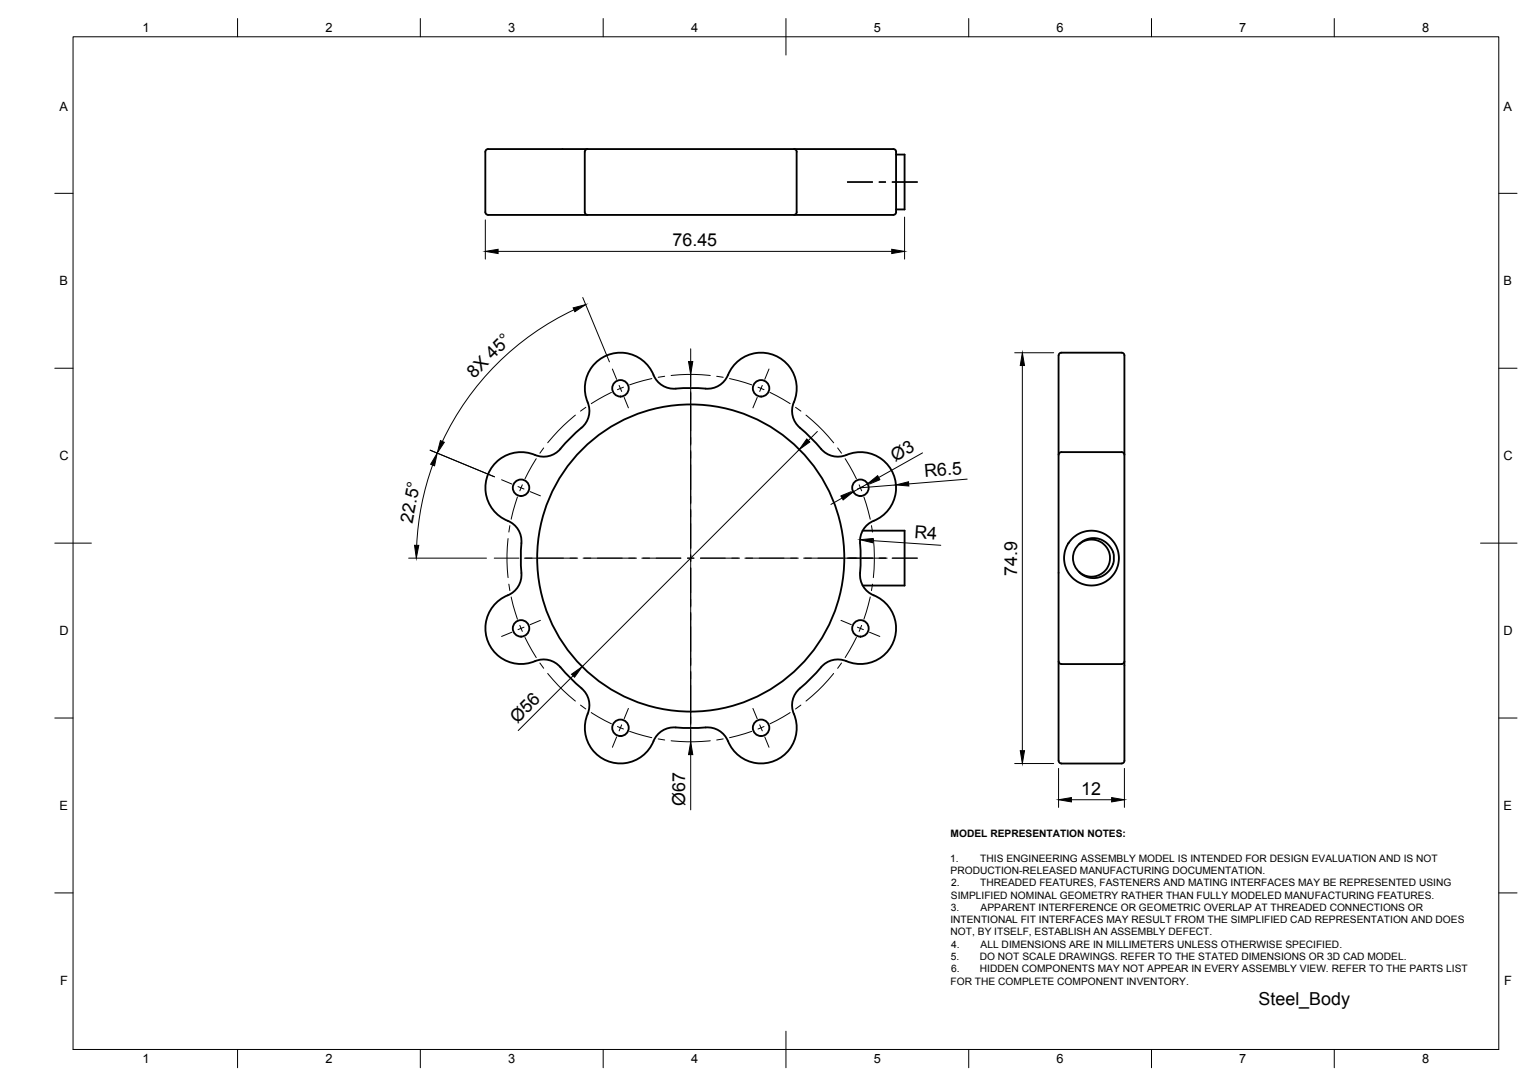
ISO-10303-21;
HEADER;
/* Generated by software containing ST-Developer
 * from STEP Tools, Inc. (www.steptools.com) 
 */

FILE_DESCRIPTION(
/* description */ (''),
/* implementation_level */ '2;1');

FILE_NAME(
/* name */ 'Steel_Body.step',
/* time_stamp */ '2026-10-06T12:52:28-07:00',
/* author */ (''),
/* organization */ (''),
/* preprocessor_version */ 'ST-DEVELOPER v20.2',
/* originating_system */ 'Autodesk Translation Framework v15.15.0.0',
/* authorisation */ '');

FILE_SCHEMA (('AUTOMOTIVE_DESIGN { 1 0 10303 214 3 1 1 }'));
ENDSEC;

DATA;
#10=MECHANICAL_DESIGN_GEOMETRIC_PRESENTATION_REPRESENTATION('',(#79),#34403);
#55=B_SPLINE_SURFACE_WITH_KNOTS('',3,3,((#32660,#32661,#32662,#32663,#32664,
#32665,#32666,#32667,#32668,#32669,#32670,#32671,#32672,#32673,#32674,#32675,
#32676,#32677,#32678,#32679,#32680,#32681,#32682,#32683,#32684,#32685,#32686,
#32687,#32688,#32689,#32690,#32691,#32692,#32693,#32694,#32695,#32696,#32697,
#32698,#32699,#32700,#32701,#32702,#32703,#32704,#32705,#32706,#32707,#32708,
#32709,#32710,#32711,#32712,#32713,#32714,#32715,#32716,#32717,#32718,#32719,
#32720),(#32721,#32722,#32723,#32724,#32725,#32726,#32727,#32728,#32729,
#32730,#32731,#32732,#32733,#32734,#32735,#32736,#32737,#32738,#32739,#32740,
#32741,#32742,#32743,#32744,#32745,#32746,#32747,#32748,#32749,#32750,#32751,
#32752,#32753,#32754,#32755,#32756,#32757,#32758,#32759,#32760,#32761,#32762,
#32763,#32764,#32765,#32766,#32767,#32768,#32769,#32770,#32771,#32772,#32773,
#32774,#32775,#32776,#32777,#32778,#32779,#32780,#32781),(#32782,#32783,
#32784,#32785,#32786,#32787,#32788,#32789,#32790,#32791,#32792,#32793,#32794,
#32795,#32796,#32797,#32798,#32799,#32800,#32801,#32802,#32803,#32804,#32805,
#32806,#32807,#32808,#32809,#32810,#32811,#32812,#32813,#32814,#32815,#32816,
#32817,#32818,#32819,#32820,#32821,#32822,#32823,#32824,#32825,#32826,#32827,
#32828,#32829,#32830,#32831,#32832,#32833,#32834,#32835,#32836,#32837,#32838,
#32839,#32840,#32841,#32842),(#32843,#32844,#32845,#32846,#32847,#32848,
#32849,#32850,#32851,#32852,#32853,#32854,#32855,#32856,#32857,#32858,#32859,
#32860,#32861,#32862,#32863,#32864,#32865,#32866,#32867,#32868,#32869,#32870,
#32871,#32872,#32873,#32874,#32875,#32876,#32877,#32878,#32879,#32880,#32881,
#32882,#32883,#32884,#32885,#32886,#32887,#32888,#32889,#32890,#32891,#32892,
#32893,#32894,#32895,#32896,#32897,#32898,#32899,#32900,#32901,#32902,#32903)),
 .UNSPECIFIED.,.F.,.F.,.F.,(4,4),(4,1,1,1,1,1,1,1,1,1,1,1,1,1,1,1,1,1,1,
1,1,1,1,1,1,1,1,1,1,1,1,1,1,1,1,1,1,1,1,1,1,1,1,1,1,1,1,1,1,1,1,1,1,1,1,
1,1,1,4),(-0.000677904662105755,0.0806892635940671),(11.8568599181543,12.8456361179191,
13.8337344130217,14.8218327081244,15.8099310032271,16.7980292983297,17.7861275934324,
18.774225888535,19.7623241836377,20.7504224787404,21.738520773843,22.7266190689457,
23.7147173640484,24.702815659151,25.6909139542537,26.6790122493564,27.667110544459,
28.6552088395617,29.6433071346644,30.631405429767,31.6195037248697,32.6076020199723,
33.595700315075,34.5837986101777,35.5718969052803,36.559995200383,37.5480934954857,
38.5361917905883,39.524290085691,40.5123883807937,41.5004866758963,42.488584970999,
43.4766832661016,44.4647815612043,45.452879856307,46.4409781514096,47.4290764465123,
48.417174741615,49.4052730367176,50.3933713318203,51.381469626923,52.3695679220256,
53.3576662171283,54.345764512231,55.3338628073336,56.3219611024363,57.3100593975389,
58.2981576926416,59.2862559877443,60.2743542828469,61.2624525779496,62.2505508730523,
63.2386491681549,64.2267474632576,65.2148457583603,66.2029440534629,67.1910423485656,
68.1791406436682,69.1672389387709),.UNSPECIFIED.);
#56=B_SPLINE_SURFACE_WITH_KNOTS('',3,3,((#33092,#33093,#33094,#33095,#33096,
#33097,#33098,#33099,#33100,#33101,#33102,#33103,#33104,#33105,#33106,#33107,
#33108,#33109,#33110,#33111,#33112,#33113,#33114,#33115,#33116,#33117,#33118,
#33119,#33120,#33121,#33122,#33123,#33124,#33125,#33126,#33127,#33128,#33129,
#33130,#33131,#33132,#33133,#33134,#33135,#33136,#33137,#33138,#33139,#33140,
#33141,#33142,#33143,#33144,#33145,#33146,#33147,#33148,#33149,#33150,#33151,
#33152),(#33153,#33154,#33155,#33156,#33157,#33158,#33159,#33160,#33161,
#33162,#33163,#33164,#33165,#33166,#33167,#33168,#33169,#33170,#33171,#33172,
#33173,#33174,#33175,#33176,#33177,#33178,#33179,#33180,#33181,#33182,#33183,
#33184,#33185,#33186,#33187,#33188,#33189,#33190,#33191,#33192,#33193,#33194,
#33195,#33196,#33197,#33198,#33199,#33200,#33201,#33202,#33203,#33204,#33205,
#33206,#33207,#33208,#33209,#33210,#33211,#33212,#33213),(#33214,#33215,
#33216,#33217,#33218,#33219,#33220,#33221,#33222,#33223,#33224,#33225,#33226,
#33227,#33228,#33229,#33230,#33231,#33232,#33233,#33234,#33235,#33236,#33237,
#33238,#33239,#33240,#33241,#33242,#33243,#33244,#33245,#33246,#33247,#33248,
#33249,#33250,#33251,#33252,#33253,#33254,#33255,#33256,#33257,#33258,#33259,
#33260,#33261,#33262,#33263,#33264,#33265,#33266,#33267,#33268,#33269,#33270,
#33271,#33272,#33273,#33274),(#33275,#33276,#33277,#33278,#33279,#33280,
#33281,#33282,#33283,#33284,#33285,#33286,#33287,#33288,#33289,#33290,#33291,
#33292,#33293,#33294,#33295,#33296,#33297,#33298,#33299,#33300,#33301,#33302,
#33303,#33304,#33305,#33306,#33307,#33308,#33309,#33310,#33311,#33312,#33313,
#33314,#33315,#33316,#33317,#33318,#33319,#33320,#33321,#33322,#33323,#33324,
#33325,#33326,#33327,#33328,#33329,#33330,#33331,#33332,#33333,#33334,#33335)),
 .UNSPECIFIED.,.F.,.F.,.F.,(4,4),(4,1,1,1,1,1,1,1,1,1,1,1,1,1,1,1,1,1,1,
1,1,1,1,1,1,1,1,1,1,1,1,1,1,1,1,1,1,1,1,1,1,1,1,1,1,1,1,1,1,1,1,1,1,1,1,
1,1,1,4),(-0.000408738892527466,0.0809585600709479),(14.3991256467175,15.3872239418202,
16.3753222369229,17.3634205320255,18.3515188271282,19.3396171222308,20.3277154173335,
21.3158137124362,22.3039120075388,23.2920103026415,24.2801085977442,25.2682068928468,
26.2563051879495,27.2444034830521,28.2325017781548,29.2206000732575,30.2086983683601,
31.1967966634628,32.1848949585655,33.1729932536681,34.1610915487708,35.1491898438735,
36.1372881389761,37.1253864340788,38.1134847291814,39.1015830242841,40.0896813193868,
41.0777796144894,42.0658779095921,43.0539762046948,44.0420744997974,45.0301727949001,
46.0182710900028,47.0063693851054,47.9944676802081,48.9825659753107,49.9706642704134,
50.9587625655161,51.9468608606187,52.9349591557214,53.9230574508241,54.9111557459267,
55.8992540410294,56.8873523361321,57.8754506312347,58.8635489263374,59.85164722144,
60.8397455165427,61.8278438116454,62.815942106748,63.8040404018507,64.7921386969534,
65.780236992056,66.7683352871587,67.7564335822614,68.744531877364,69.7326301724667,
70.7207284675693,71.7095047678121),.UNSPECIFIED.);
#63=SHAPE_REPRESENTATION_RELATIONSHIP('SRR','None',#34441,#71);
#71=ADVANCED_BREP_SHAPE_REPRESENTATION('',(#87),#34401);
#79=STYLED_ITEM('',(#34484),#87);
#87=MANIFOLD_SOLID_BREP('Body1',#4388);
#102=FACE_BOUND('',#855,.T.);
#103=FACE_BOUND('',#858,.T.);
#104=FACE_BOUND('',#914,.T.);
#105=FACE_BOUND('',#915,.T.);
#106=FACE_BOUND('',#916,.T.);
#107=FACE_BOUND('',#917,.T.);
#108=FACE_BOUND('',#918,.T.);
#109=FACE_BOUND('',#919,.T.);
#110=FACE_BOUND('',#920,.T.);
#111=FACE_BOUND('',#921,.T.);
#112=FACE_BOUND('',#922,.T.);
#113=FACE_BOUND('',#970,.T.);
#114=FACE_BOUND('',#971,.T.);
#115=FACE_BOUND('',#972,.T.);
#116=FACE_BOUND('',#973,.T.);
#117=FACE_BOUND('',#974,.T.);
#118=FACE_BOUND('',#975,.T.);
#119=FACE_BOUND('',#976,.T.);
#120=FACE_BOUND('',#977,.T.);
#121=FACE_BOUND('',#978,.T.);
#122=FACE_BOUND('',#981,.T.);
#123=FACE_BOUND('',#982,.T.);
#143=PLANE('',#4620);
#144=PLANE('',#4625);
#145=PLANE('',#4794);
#146=PLANE('',#4928);
#207=CIRCLE('',#4606,4.085);
#208=CIRCLE('',#4615,4.085);
#209=CIRCLE('',#4617,3.38975);
#210=CIRCLE('',#4618,3.38975);
#211=CIRCLE('',#4621,5.);
#212=CIRCLE('',#4622,5.);
#213=CIRCLE('',#4624,5.);
#214=CIRCLE('',#4630,4.);
#215=CIRCLE('',#4631,4.);
#216=CIRCLE('',#4633,31.);
#217=CIRCLE('',#4635,4.);
#218=CIRCLE('',#4636,4.);
#219=CIRCLE('',#4638,31.);
#220=CIRCLE('',#4640,0.499999999999994);
#221=CIRCLE('',#4641,4.5);
#222=CIRCLE('',#4642,0.5);
#223=CIRCLE('',#4644,0.5);
#224=CIRCLE('',#4645,6.5);
#225=CIRCLE('',#4646,6.);
#226=CIRCLE('',#4648,0.5);
#227=CIRCLE('',#4649,4.);
#228=CIRCLE('',#4650,4.5);
#229=CIRCLE('',#4652,0.5);
#230=CIRCLE('',#4653,31.);
#231=CIRCLE('',#4654,30.5);
#232=CIRCLE('',#4656,0.5);
#233=CIRCLE('',#4657,4.);
#234=CIRCLE('',#4658,4.5);
#235=CIRCLE('',#4660,0.5);
#236=CIRCLE('',#4661,6.5);
#237=CIRCLE('',#4662,6.);
#238=CIRCLE('',#4664,0.5);
#239=CIRCLE('',#4665,4.);
#240=CIRCLE('',#4666,4.5);
#241=CIRCLE('',#4668,0.5);
#242=CIRCLE('',#4669,31.);
#243=CIRCLE('',#4670,30.5);
#244=CIRCLE('',#4672,0.5);
#245=CIRCLE('',#4673,4.);
#246=CIRCLE('',#4674,4.5);
#247=CIRCLE('',#4676,0.5);
#248=CIRCLE('',#4677,6.5);
#249=CIRCLE('',#4678,6.);
#250=CIRCLE('',#4680,0.5);
#251=CIRCLE('',#4681,4.);
#252=CIRCLE('',#4682,4.5);
#253=CIRCLE('',#4684,0.5);
#254=CIRCLE('',#4685,31.);
#255=CIRCLE('',#4686,30.5);
#256=CIRCLE('',#4688,0.5);
#257=CIRCLE('',#4689,4.);
#258=CIRCLE('',#4690,4.5);
#259=CIRCLE('',#4692,0.5);
#260=CIRCLE('',#4693,6.5);
#261=CIRCLE('',#4694,6.);
#262=CIRCLE('',#4696,0.5);
#263=CIRCLE('',#4697,4.5);
#264=CIRCLE('',#4699,0.5);
#265=CIRCLE('',#4700,31.);
#266=CIRCLE('',#4701,30.5);
#267=CIRCLE('',#4703,0.5);
#268=CIRCLE('',#4704,4.);
#269=CIRCLE('',#4705,4.5);
#270=CIRCLE('',#4707,0.5);
#271=CIRCLE('',#4708,6.5);
#272=CIRCLE('',#4709,6.);
#273=CIRCLE('',#4711,0.5);
#274=CIRCLE('',#4712,4.);
#275=CIRCLE('',#4713,4.5);
#276=CIRCLE('',#4715,0.5);
#277=CIRCLE('',#4716,31.);
#278=CIRCLE('',#4717,30.5);
#279=CIRCLE('',#4719,0.5);
#280=CIRCLE('',#4720,4.);
#281=CIRCLE('',#4721,4.5);
#282=CIRCLE('',#4723,0.5);
#283=CIRCLE('',#4724,6.5);
#284=CIRCLE('',#4725,6.);
#285=CIRCLE('',#4727,0.5);
#286=CIRCLE('',#4728,4.);
#287=CIRCLE('',#4729,4.5);
#288=CIRCLE('',#4731,0.5);
#289=CIRCLE('',#4732,31.);
#290=CIRCLE('',#4733,30.5);
#291=CIRCLE('',#4735,0.5);
#292=CIRCLE('',#4736,4.);
#293=CIRCLE('',#4737,4.5);
#294=CIRCLE('',#4739,0.5);
#295=CIRCLE('',#4740,6.5);
#296=CIRCLE('',#4741,6.);
#297=CIRCLE('',#4743,0.5);
#298=CIRCLE('',#4744,4.);
#299=CIRCLE('',#4745,4.5);
#300=CIRCLE('',#4747,0.5);
#301=CIRCLE('',#4748,31.);
#302=CIRCLE('',#4749,30.5);
#303=CIRCLE('',#4751,0.5);
#304=CIRCLE('',#4752,4.);
#305=CIRCLE('',#4753,4.5);
#306=CIRCLE('',#4755,0.5);
#307=CIRCLE('',#4756,6.5);
#308=CIRCLE('',#4757,6.);
#309=CIRCLE('',#4759,0.5);
#310=CIRCLE('',#4760,4.);
#311=CIRCLE('',#4761,4.5);
#312=CIRCLE('',#4763,30.5);
#313=CIRCLE('',#4765,6.5);
#314=CIRCLE('',#4767,4.);
#315=CIRCLE('',#4769,31.);
#316=CIRCLE('',#4771,4.);
#317=CIRCLE('',#4773,6.5);
#318=CIRCLE('',#4775,4.);
#319=CIRCLE('',#4777,31.);
#320=CIRCLE('',#4779,4.);
#321=CIRCLE('',#4781,6.5);
#322=CIRCLE('',#4783,4.);
#323=CIRCLE('',#4785,31.);
#324=CIRCLE('',#4787,4.);
#325=CIRCLE('',#4789,6.5);
#326=CIRCLE('',#4791,4.);
#327=CIRCLE('',#4793,31.);
#328=CIRCLE('',#4795,28.5);
#329=CIRCLE('',#4796,1.5);
#330=CIRCLE('',#4797,1.5);
#331=CIRCLE('',#4798,1.5);
#332=CIRCLE('',#4799,1.5);
#333=CIRCLE('',#4800,1.5);
#334=CIRCLE('',#4801,1.5);
#335=CIRCLE('',#4802,1.5);
#336=CIRCLE('',#4803,1.5);
#337=CIRCLE('',#4805,0.500000000000001);
#338=CIRCLE('',#4806,4.5);
#339=CIRCLE('',#4807,0.5);
#340=CIRCLE('',#4808,4.);
#341=CIRCLE('',#4810,0.5);
#342=CIRCLE('',#4811,6.5);
#343=CIRCLE('',#4812,6.);
#344=CIRCLE('',#4814,0.5);
#345=CIRCLE('',#4815,4.5);
#346=CIRCLE('',#4817,0.5);
#347=CIRCLE('',#4818,30.5);
#348=CIRCLE('',#4820,0.5);
#349=CIRCLE('',#4821,4.5);
#350=CIRCLE('',#4823,0.5);
#351=CIRCLE('',#4824,6.);
#352=CIRCLE('',#4826,0.5);
#353=CIRCLE('',#4827,4.5);
#354=CIRCLE('',#4829,0.5);
#355=CIRCLE('',#4830,30.5);
#356=CIRCLE('',#4832,0.5);
#357=CIRCLE('',#4833,4.5);
#358=CIRCLE('',#4835,0.5);
#359=CIRCLE('',#4836,6.);
#360=CIRCLE('',#4838,0.5);
#361=CIRCLE('',#4839,4.5);
#362=CIRCLE('',#4841,0.5);
#363=CIRCLE('',#4842,30.5);
#364=CIRCLE('',#4844,0.5);
#365=CIRCLE('',#4845,4.5);
#366=CIRCLE('',#4847,0.5);
#367=CIRCLE('',#4848,6.);
#368=CIRCLE('',#4850,0.5);
#369=CIRCLE('',#4851,4.5);
#370=CIRCLE('',#4853,0.5);
#371=CIRCLE('',#4854,30.5);
#372=CIRCLE('',#4856,0.5);
#373=CIRCLE('',#4857,4.5);
#374=CIRCLE('',#4859,0.5);
#375=CIRCLE('',#4860,6.);
#376=CIRCLE('',#4862,0.5);
#377=CIRCLE('',#4863,4.);
#378=CIRCLE('',#4864,4.5);
#379=CIRCLE('',#4866,0.5);
#380=CIRCLE('',#4867,30.5);
#381=CIRCLE('',#4869,0.5);
#382=CIRCLE('',#4870,4.5);
#383=CIRCLE('',#4872,0.5);
#384=CIRCLE('',#4873,6.5);
#385=CIRCLE('',#4874,6.);
#386=CIRCLE('',#4876,0.5);
#387=CIRCLE('',#4877,4.);
#388=CIRCLE('',#4878,4.5);
#389=CIRCLE('',#4880,0.5);
#390=CIRCLE('',#4881,31.);
#391=CIRCLE('',#4882,30.5);
#392=CIRCLE('',#4884,0.5);
#393=CIRCLE('',#4885,4.);
#394=CIRCLE('',#4886,4.5);
#395=CIRCLE('',#4888,0.5);
#396=CIRCLE('',#4889,6.5);
#397=CIRCLE('',#4890,6.);
#398=CIRCLE('',#4892,0.5);
#399=CIRCLE('',#4893,4.);
#400=CIRCLE('',#4894,4.5);
#401=CIRCLE('',#4896,0.5);
#402=CIRCLE('',#4897,31.);
#403=CIRCLE('',#4898,30.5);
#404=CIRCLE('',#4900,0.5);
#405=CIRCLE('',#4901,4.);
#406=CIRCLE('',#4902,4.5);
#407=CIRCLE('',#4904,0.5);
#408=CIRCLE('',#4905,6.5);
#409=CIRCLE('',#4906,6.);
#410=CIRCLE('',#4908,0.5);
#411=CIRCLE('',#4909,4.);
#412=CIRCLE('',#4910,4.5);
#413=CIRCLE('',#4912,30.5);
#414=CIRCLE('',#4913,31.);
#415=CIRCLE('',#4929,28.5);
#416=CIRCLE('',#4930,1.5);
#417=CIRCLE('',#4931,1.5);
#418=CIRCLE('',#4932,1.5);
#419=CIRCLE('',#4933,1.5);
#420=CIRCLE('',#4934,1.5);
#421=CIRCLE('',#4935,1.5);
#422=CIRCLE('',#4936,1.5);
#423=CIRCLE('',#4937,1.5);
#424=CIRCLE('',#4939,0.5);
#425=CIRCLE('',#4940,28.);
#426=CIRCLE('',#4941,28.);
#427=CIRCLE('',#4943,28.);
#428=CIRCLE('',#4944,28.);
#429=CIRCLE('',#4946,0.5);
#450=TOROIDAL_SURFACE('',#4639,4.5,0.5);
#451=TOROIDAL_SURFACE('',#4643,6.,0.5);
#452=TOROIDAL_SURFACE('',#4647,4.5,0.5);
#453=TOROIDAL_SURFACE('',#4651,30.5,0.5);
#454=TOROIDAL_SURFACE('',#4655,4.5,0.5);
#455=TOROIDAL_SURFACE('',#4659,6.,0.5);
#456=TOROIDAL_SURFACE('',#4663,4.5,0.5);
#457=TOROIDAL_SURFACE('',#4667,30.5,0.5);
#458=TOROIDAL_SURFACE('',#4671,4.5,0.5);
#459=TOROIDAL_SURFACE('',#4675,6.,0.5);
#460=TOROIDAL_SURFACE('',#4679,4.5,0.5);
#461=TOROIDAL_SURFACE('',#4683,30.5,0.5);
#462=TOROIDAL_SURFACE('',#4687,4.5,0.5);
#463=TOROIDAL_SURFACE('',#4691,6.,0.5);
#464=TOROIDAL_SURFACE('',#4695,4.5,0.5);
#465=TOROIDAL_SURFACE('',#4698,30.5,0.5);
#466=TOROIDAL_SURFACE('',#4702,4.5,0.5);
#467=TOROIDAL_SURFACE('',#4706,6.,0.5);
#468=TOROIDAL_SURFACE('',#4710,4.5,0.5);
#469=TOROIDAL_SURFACE('',#4714,30.5,0.5);
#470=TOROIDAL_SURFACE('',#4718,4.5,0.5);
#471=TOROIDAL_SURFACE('',#4722,6.,0.5);
#472=TOROIDAL_SURFACE('',#4726,4.5,0.5);
#473=TOROIDAL_SURFACE('',#4730,30.5,0.5);
#474=TOROIDAL_SURFACE('',#4734,4.5,0.5);
#475=TOROIDAL_SURFACE('',#4738,6.,0.5);
#476=TOROIDAL_SURFACE('',#4742,4.5,0.5);
#477=TOROIDAL_SURFACE('',#4746,30.5,0.5);
#478=TOROIDAL_SURFACE('',#4750,4.5,0.5);
#479=TOROIDAL_SURFACE('',#4754,6.,0.5);
#480=TOROIDAL_SURFACE('',#4758,4.5,0.5);
#481=TOROIDAL_SURFACE('',#4762,30.5,0.5);
#482=TOROIDAL_SURFACE('',#4804,4.5,0.5);
#483=TOROIDAL_SURFACE('',#4809,6.,0.5);
#484=TOROIDAL_SURFACE('',#4813,4.5,0.5);
#485=TOROIDAL_SURFACE('',#4816,30.5,0.5);
#486=TOROIDAL_SURFACE('',#4819,4.5,0.5);
#487=TOROIDAL_SURFACE('',#4822,6.,0.5);
#488=TOROIDAL_SURFACE('',#4825,4.5,0.5);
#489=TOROIDAL_SURFACE('',#4828,30.5,0.5);
#490=TOROIDAL_SURFACE('',#4831,4.5,0.5);
#491=TOROIDAL_SURFACE('',#4834,6.,0.5);
#492=TOROIDAL_SURFACE('',#4837,4.5,0.5);
#493=TOROIDAL_SURFACE('',#4840,30.5,0.5);
#494=TOROIDAL_SURFACE('',#4843,4.5,0.5);
#495=TOROIDAL_SURFACE('',#4846,6.,0.5);
#496=TOROIDAL_SURFACE('',#4849,4.5,0.5);
#497=TOROIDAL_SURFACE('',#4852,30.5,0.5);
#498=TOROIDAL_SURFACE('',#4855,4.5,0.5);
#499=TOROIDAL_SURFACE('',#4858,6.,0.5);
#500=TOROIDAL_SURFACE('',#4861,4.5,0.5);
#501=TOROIDAL_SURFACE('',#4865,30.5,0.5);
#502=TOROIDAL_SURFACE('',#4868,4.5,0.5);
#503=TOROIDAL_SURFACE('',#4871,6.,0.5);
#504=TOROIDAL_SURFACE('',#4875,4.5,0.5);
#505=TOROIDAL_SURFACE('',#4879,30.5,0.5);
#506=TOROIDAL_SURFACE('',#4883,4.5,0.5);
#507=TOROIDAL_SURFACE('',#4887,6.,0.5);
#508=TOROIDAL_SURFACE('',#4891,4.5,0.5);
#509=TOROIDAL_SURFACE('',#4895,30.5,0.5);
#510=TOROIDAL_SURFACE('',#4899,4.5,0.5);
#511=TOROIDAL_SURFACE('',#4903,6.,0.5);
#512=TOROIDAL_SURFACE('',#4907,4.5,0.5);
#513=TOROIDAL_SURFACE('',#4911,30.5,0.5);
#514=TOROIDAL_SURFACE('',#4938,28.5,0.5);
#515=TOROIDAL_SURFACE('',#4945,28.5,0.5);
#597=FACE_OUTER_BOUND('',#841,.T.);
#598=FACE_OUTER_BOUND('',#842,.T.);
#599=FACE_OUTER_BOUND('',#843,.T.);
#600=FACE_OUTER_BOUND('',#844,.T.);
#601=FACE_OUTER_BOUND('',#845,.T.);
#602=FACE_OUTER_BOUND('',#846,.T.);
#603=FACE_OUTER_BOUND('',#847,.T.);
#604=FACE_OUTER_BOUND('',#848,.T.);
#605=FACE_OUTER_BOUND('',#849,.T.);
#606=FACE_OUTER_BOUND('',#850,.T.);
#607=FACE_OUTER_BOUND('',#851,.T.);
#608=FACE_OUTER_BOUND('',#852,.T.);
#609=FACE_OUTER_BOUND('',#853,.T.);
#610=FACE_OUTER_BOUND('',#854,.T.);
#611=FACE_OUTER_BOUND('',#856,.T.);
#612=FACE_OUTER_BOUND('',#857,.T.);
#613=FACE_OUTER_BOUND('',#859,.T.);
#614=FACE_OUTER_BOUND('',#860,.T.);
#615=FACE_OUTER_BOUND('',#861,.T.);
#616=FACE_OUTER_BOUND('',#862,.T.);
#617=FACE_OUTER_BOUND('',#863,.T.);
#618=FACE_OUTER_BOUND('',#864,.T.);
#619=FACE_OUTER_BOUND('',#865,.T.);
#620=FACE_OUTER_BOUND('',#866,.T.);
#621=FACE_OUTER_BOUND('',#867,.T.);
#622=FACE_OUTER_BOUND('',#868,.T.);
#623=FACE_OUTER_BOUND('',#869,.T.);
#624=FACE_OUTER_BOUND('',#870,.T.);
#625=FACE_OUTER_BOUND('',#871,.T.);
#626=FACE_OUTER_BOUND('',#872,.T.);
#627=FACE_OUTER_BOUND('',#873,.T.);
#628=FACE_OUTER_BOUND('',#874,.T.);
#629=FACE_OUTER_BOUND('',#875,.T.);
#630=FACE_OUTER_BOUND('',#876,.T.);
#631=FACE_OUTER_BOUND('',#877,.T.);
#632=FACE_OUTER_BOUND('',#878,.T.);
#633=FACE_OUTER_BOUND('',#879,.T.);
#634=FACE_OUTER_BOUND('',#880,.T.);
#635=FACE_OUTER_BOUND('',#881,.T.);
#636=FACE_OUTER_BOUND('',#882,.T.);
#637=FACE_OUTER_BOUND('',#883,.T.);
#638=FACE_OUTER_BOUND('',#884,.T.);
#639=FACE_OUTER_BOUND('',#885,.T.);
#640=FACE_OUTER_BOUND('',#886,.T.);
#641=FACE_OUTER_BOUND('',#887,.T.);
#642=FACE_OUTER_BOUND('',#888,.T.);
#643=FACE_OUTER_BOUND('',#889,.T.);
#644=FACE_OUTER_BOUND('',#890,.T.);
#645=FACE_OUTER_BOUND('',#891,.T.);
#646=FACE_OUTER_BOUND('',#892,.T.);
#647=FACE_OUTER_BOUND('',#893,.T.);
#648=FACE_OUTER_BOUND('',#894,.T.);
#649=FACE_OUTER_BOUND('',#895,.T.);
#650=FACE_OUTER_BOUND('',#896,.T.);
#651=FACE_OUTER_BOUND('',#897,.T.);
#652=FACE_OUTER_BOUND('',#898,.T.);
#653=FACE_OUTER_BOUND('',#899,.T.);
#654=FACE_OUTER_BOUND('',#900,.T.);
#655=FACE_OUTER_BOUND('',#901,.T.);
#656=FACE_OUTER_BOUND('',#902,.T.);
#657=FACE_OUTER_BOUND('',#903,.T.);
#658=FACE_OUTER_BOUND('',#904,.T.);
#659=FACE_OUTER_BOUND('',#905,.T.);
#660=FACE_OUTER_BOUND('',#906,.T.);
#661=FACE_OUTER_BOUND('',#907,.T.);
#662=FACE_OUTER_BOUND('',#908,.T.);
#663=FACE_OUTER_BOUND('',#909,.T.);
#664=FACE_OUTER_BOUND('',#910,.T.);
#665=FACE_OUTER_BOUND('',#911,.T.);
#666=FACE_OUTER_BOUND('',#912,.T.);
#667=FACE_OUTER_BOUND('',#913,.T.);
#668=FACE_OUTER_BOUND('',#923,.T.);
#669=FACE_OUTER_BOUND('',#924,.T.);
#670=FACE_OUTER_BOUND('',#925,.T.);
#671=FACE_OUTER_BOUND('',#926,.T.);
#672=FACE_OUTER_BOUND('',#927,.T.);
#673=FACE_OUTER_BOUND('',#928,.T.);
#674=FACE_OUTER_BOUND('',#929,.T.);
#675=FACE_OUTER_BOUND('',#930,.T.);
#676=FACE_OUTER_BOUND('',#931,.T.);
#677=FACE_OUTER_BOUND('',#932,.T.);
#678=FACE_OUTER_BOUND('',#933,.T.);
#679=FACE_OUTER_BOUND('',#934,.T.);
#680=FACE_OUTER_BOUND('',#935,.T.);
#681=FACE_OUTER_BOUND('',#936,.T.);
#682=FACE_OUTER_BOUND('',#937,.T.);
#683=FACE_OUTER_BOUND('',#938,.T.);
#684=FACE_OUTER_BOUND('',#939,.T.);
#685=FACE_OUTER_BOUND('',#940,.T.);
#686=FACE_OUTER_BOUND('',#941,.T.);
#687=FACE_OUTER_BOUND('',#942,.T.);
#688=FACE_OUTER_BOUND('',#943,.T.);
#689=FACE_OUTER_BOUND('',#944,.T.);
#690=FACE_OUTER_BOUND('',#945,.T.);
#691=FACE_OUTER_BOUND('',#946,.T.);
#692=FACE_OUTER_BOUND('',#947,.T.);
#693=FACE_OUTER_BOUND('',#948,.T.);
#694=FACE_OUTER_BOUND('',#949,.T.);
#695=FACE_OUTER_BOUND('',#950,.T.);
#696=FACE_OUTER_BOUND('',#951,.T.);
#697=FACE_OUTER_BOUND('',#952,.T.);
#698=FACE_OUTER_BOUND('',#953,.T.);
#699=FACE_OUTER_BOUND('',#954,.T.);
#700=FACE_OUTER_BOUND('',#955,.T.);
#701=FACE_OUTER_BOUND('',#956,.T.);
#702=FACE_OUTER_BOUND('',#957,.T.);
#703=FACE_OUTER_BOUND('',#958,.T.);
#704=FACE_OUTER_BOUND('',#959,.T.);
#705=FACE_OUTER_BOUND('',#960,.T.);
#706=FACE_OUTER_BOUND('',#961,.T.);
#707=FACE_OUTER_BOUND('',#962,.T.);
#708=FACE_OUTER_BOUND('',#963,.T.);
#709=FACE_OUTER_BOUND('',#964,.T.);
#710=FACE_OUTER_BOUND('',#965,.T.);
#711=FACE_OUTER_BOUND('',#966,.T.);
#712=FACE_OUTER_BOUND('',#967,.T.);
#713=FACE_OUTER_BOUND('',#968,.T.);
#714=FACE_OUTER_BOUND('',#969,.T.);
#715=FACE_OUTER_BOUND('',#979,.T.);
#716=FACE_OUTER_BOUND('',#980,.T.);
#717=FACE_OUTER_BOUND('',#983,.T.);
#718=FACE_OUTER_BOUND('',#984,.T.);
#719=FACE_OUTER_BOUND('',#985,.T.);
#720=FACE_OUTER_BOUND('',#986,.T.);
#721=FACE_OUTER_BOUND('',#987,.T.);
#722=FACE_OUTER_BOUND('',#988,.T.);
#723=FACE_OUTER_BOUND('',#989,.T.);
#724=FACE_OUTER_BOUND('',#990,.T.);
#725=FACE_OUTER_BOUND('',#991,.T.);
#726=FACE_OUTER_BOUND('',#992,.T.);
#841=EDGE_LOOP('',(#3249,#3250,#3251,#3252));
#842=EDGE_LOOP('',(#3253,#3254,#3255,#3256,#3257,#3258));
#843=EDGE_LOOP('',(#3259,#3260,#3261,#3262,#3263,#3264));
#844=EDGE_LOOP('',(#3265,#3266,#3267,#3268,#3269,#3270));
#845=EDGE_LOOP('',(#3271,#3272,#3273,#3274,#3275,#3276));
#846=EDGE_LOOP('',(#3277,#3278,#3279,#3280,#3281,#3282));
#847=EDGE_LOOP('',(#3283,#3284,#3285,#3286,#3287,#3288));
#848=EDGE_LOOP('',(#3289,#3290,#3291,#3292,#3293,#3294));
#849=EDGE_LOOP('',(#3295,#3296,#3297,#3298,#3299,#3300));
#850=EDGE_LOOP('',(#3301,#3302,#3303,#3304,#3305,#3306,#3307,#3308,#3309,
#3310,#3311,#3312,#3313,#3314,#3315));
#851=EDGE_LOOP('',(#3316,#3317,#3318,#3319,#3320,#3321));
#852=EDGE_LOOP('',(#3322,#3323,#3324,#3325,#3326,#3327,#3328,#3329,#3330,
#3331,#3332,#3333,#3334,#3335,#3336,#3337,#3338,#3339,#3340,#3341,#3342,
#3343,#3344,#3345,#3346,#3347,#3348,#3349));
#853=EDGE_LOOP('',(#3350,#3351,#3352,#3353,#3354,#3355,#3356,#3357,#3358,
#3359,#3360,#3361,#3362,#3363,#3364,#3365,#3366,#3367,#3368,#3369,#3370,
#3371,#3372,#3373,#3374,#3375,#3376));
#854=EDGE_LOOP('',(#3377,#3378));
#855=EDGE_LOOP('',(#3379,#3380,#3381,#3382));
#856=EDGE_LOOP('',(#3383,#3384,#3385,#3386,#3387,#3388,#3389,#3390));
#857=EDGE_LOOP('',(#3391));
#858=EDGE_LOOP('',(#3392,#3393,#3394,#3395));
#859=EDGE_LOOP('',(#3396,#3397));
#860=EDGE_LOOP('',(#3398,#3399));
#861=EDGE_LOOP('',(#3400,#3401,#3402,#3403,#3404,#3405,#3406,#3407));
#862=EDGE_LOOP('',(#3408,#3409,#3410,#3411,#3412,#3413,#3414));
#863=EDGE_LOOP('',(#3415,#3416,#3417,#3418));
#864=EDGE_LOOP('',(#3419,#3420,#3421,#3422,#3423,#3424,#3425));
#865=EDGE_LOOP('',(#3426,#3427,#3428,#3429));
#866=EDGE_LOOP('',(#3430,#3431,#3432,#3433));
#867=EDGE_LOOP('',(#3434,#3435,#3436,#3437));
#868=EDGE_LOOP('',(#3438,#3439,#3440,#3441));
#869=EDGE_LOOP('',(#3442,#3443,#3444,#3445));
#870=EDGE_LOOP('',(#3446,#3447,#3448,#3449));
#871=EDGE_LOOP('',(#3450,#3451,#3452,#3453));
#872=EDGE_LOOP('',(#3454,#3455,#3456,#3457));
#873=EDGE_LOOP('',(#3458,#3459,#3460,#3461));
#874=EDGE_LOOP('',(#3462,#3463,#3464,#3465));
#875=EDGE_LOOP('',(#3466,#3467,#3468,#3469));
#876=EDGE_LOOP('',(#3470,#3471,#3472,#3473));
#877=EDGE_LOOP('',(#3474,#3475,#3476,#3477));
#878=EDGE_LOOP('',(#3478,#3479,#3480,#3481));
#879=EDGE_LOOP('',(#3482,#3483,#3484,#3485));
#880=EDGE_LOOP('',(#3486,#3487,#3488,#3489));
#881=EDGE_LOOP('',(#3490,#3491,#3492,#3493));
#882=EDGE_LOOP('',(#3494,#3495,#3496,#3497));
#883=EDGE_LOOP('',(#3498,#3499,#3500,#3501));
#884=EDGE_LOOP('',(#3502,#3503,#3504,#3505));
#885=EDGE_LOOP('',(#3506,#3507,#3508,#3509));
#886=EDGE_LOOP('',(#3510,#3511,#3512,#3513));
#887=EDGE_LOOP('',(#3514,#3515,#3516,#3517));
#888=EDGE_LOOP('',(#3518,#3519,#3520,#3521));
#889=EDGE_LOOP('',(#3522,#3523,#3524,#3525));
#890=EDGE_LOOP('',(#3526,#3527,#3528,#3529));
#891=EDGE_LOOP('',(#3530,#3531,#3532,#3533));
#892=EDGE_LOOP('',(#3534,#3535,#3536,#3537));
#893=EDGE_LOOP('',(#3538,#3539,#3540,#3541));
#894=EDGE_LOOP('',(#3542,#3543,#3544,#3545));
#895=EDGE_LOOP('',(#3546,#3547,#3548,#3549));
#896=EDGE_LOOP('',(#3550,#3551,#3552,#3553));
#897=EDGE_LOOP('',(#3554,#3555,#3556,#3557));
#898=EDGE_LOOP('',(#3558,#3559,#3560,#3561));
#899=EDGE_LOOP('',(#3562,#3563,#3564,#3565));
#900=EDGE_LOOP('',(#3566,#3567,#3568,#3569));
#901=EDGE_LOOP('',(#3570,#3571,#3572,#3573));
#902=EDGE_LOOP('',(#3574,#3575,#3576,#3577));
#903=EDGE_LOOP('',(#3578,#3579,#3580,#3581));
#904=EDGE_LOOP('',(#3582,#3583,#3584,#3585));
#905=EDGE_LOOP('',(#3586,#3587,#3588,#3589));
#906=EDGE_LOOP('',(#3590,#3591,#3592,#3593));
#907=EDGE_LOOP('',(#3594,#3595,#3596,#3597));
#908=EDGE_LOOP('',(#3598,#3599,#3600,#3601));
#909=EDGE_LOOP('',(#3602,#3603,#3604,#3605));
#910=EDGE_LOOP('',(#3606,#3607,#3608,#3609));
#911=EDGE_LOOP('',(#3610,#3611,#3612,#3613,#3614,#3615));
#912=EDGE_LOOP('',(#3616,#3617,#3618,#3619));
#913=EDGE_LOOP('',(#3620,#3621,#3622,#3623,#3624,#3625,#3626,#3627,#3628,
#3629,#3630,#3631,#3632,#3633,#3634,#3635,#3636,#3637,#3638,#3639,#3640,
#3641,#3642,#3643,#3644,#3645,#3646,#3647,#3648,#3649,#3650,#3651));
#914=EDGE_LOOP('',(#3652));
#915=EDGE_LOOP('',(#3653));
#916=EDGE_LOOP('',(#3654));
#917=EDGE_LOOP('',(#3655));
#918=EDGE_LOOP('',(#3656));
#919=EDGE_LOOP('',(#3657));
#920=EDGE_LOOP('',(#3658));
#921=EDGE_LOOP('',(#3659));
#922=EDGE_LOOP('',(#3660));
#923=EDGE_LOOP('',(#3661,#3662,#3663,#3664));
#924=EDGE_LOOP('',(#3665,#3666,#3667,#3668));
#925=EDGE_LOOP('',(#3669,#3670,#3671,#3672));
#926=EDGE_LOOP('',(#3673,#3674,#3675,#3676));
#927=EDGE_LOOP('',(#3677,#3678,#3679,#3680));
#928=EDGE_LOOP('',(#3681,#3682,#3683,#3684));
#929=EDGE_LOOP('',(#3685,#3686,#3687,#3688));
#930=EDGE_LOOP('',(#3689,#3690,#3691,#3692));
#931=EDGE_LOOP('',(#3693,#3694,#3695,#3696));
#932=EDGE_LOOP('',(#3697,#3698,#3699,#3700));
#933=EDGE_LOOP('',(#3701,#3702,#3703,#3704));
#934=EDGE_LOOP('',(#3705,#3706,#3707,#3708));
#935=EDGE_LOOP('',(#3709,#3710,#3711,#3712));
#936=EDGE_LOOP('',(#3713,#3714,#3715,#3716));
#937=EDGE_LOOP('',(#3717,#3718,#3719,#3720));
#938=EDGE_LOOP('',(#3721,#3722,#3723,#3724));
#939=EDGE_LOOP('',(#3725,#3726,#3727,#3728));
#940=EDGE_LOOP('',(#3729,#3730,#3731,#3732));
#941=EDGE_LOOP('',(#3733,#3734,#3735,#3736));
#942=EDGE_LOOP('',(#3737,#3738,#3739,#3740));
#943=EDGE_LOOP('',(#3741,#3742,#3743,#3744));
#944=EDGE_LOOP('',(#3745,#3746,#3747,#3748));
#945=EDGE_LOOP('',(#3749,#3750,#3751,#3752));
#946=EDGE_LOOP('',(#3753,#3754,#3755,#3756));
#947=EDGE_LOOP('',(#3757,#3758,#3759,#3760));
#948=EDGE_LOOP('',(#3761,#3762,#3763,#3764));
#949=EDGE_LOOP('',(#3765,#3766,#3767,#3768));
#950=EDGE_LOOP('',(#3769,#3770,#3771,#3772));
#951=EDGE_LOOP('',(#3773,#3774,#3775,#3776));
#952=EDGE_LOOP('',(#3777,#3778,#3779,#3780));
#953=EDGE_LOOP('',(#3781,#3782,#3783,#3784));
#954=EDGE_LOOP('',(#3785,#3786,#3787,#3788));
#955=EDGE_LOOP('',(#3789,#3790,#3791,#3792,#3793,#3794));
#956=EDGE_LOOP('',(#3795,#3796,#3797,#3798));
#957=EDGE_LOOP('',(#3799,#3800,#3801,#3802));
#958=EDGE_LOOP('',(#3803,#3804,#3805,#3806));
#959=EDGE_LOOP('',(#3807,#3808,#3809,#3810));
#960=EDGE_LOOP('',(#3811,#3812,#3813,#3814));
#961=EDGE_LOOP('',(#3815,#3816,#3817,#3818));
#962=EDGE_LOOP('',(#3819,#3820,#3821,#3822));
#963=EDGE_LOOP('',(#3823,#3824,#3825,#3826));
#964=EDGE_LOOP('',(#3827,#3828,#3829,#3830));
#965=EDGE_LOOP('',(#3831,#3832,#3833,#3834));
#966=EDGE_LOOP('',(#3835,#3836,#3837,#3838));
#967=EDGE_LOOP('',(#3839,#3840,#3841,#3842));
#968=EDGE_LOOP('',(#3843,#3844,#3845,#3846));
#969=EDGE_LOOP('',(#3847,#3848,#3849,#3850,#3851,#3852,#3853,#3854,#3855,
#3856,#3857,#3858,#3859,#3860,#3861,#3862,#3863,#3864,#3865,#3866,#3867,
#3868,#3869,#3870,#3871,#3872,#3873,#3874,#3875,#3876,#3877,#3878));
#970=EDGE_LOOP('',(#3879));
#971=EDGE_LOOP('',(#3880));
#972=EDGE_LOOP('',(#3881));
#973=EDGE_LOOP('',(#3882));
#974=EDGE_LOOP('',(#3883));
#975=EDGE_LOOP('',(#3884));
#976=EDGE_LOOP('',(#3885));
#977=EDGE_LOOP('',(#3886));
#978=EDGE_LOOP('',(#3887));
#979=EDGE_LOOP('',(#3888,#3889,#3890,#3891,#3892));
#980=EDGE_LOOP('',(#3893,#3894,#3895,#3896,#3897,#3898));
#981=EDGE_LOOP('',(#3899));
#982=EDGE_LOOP('',(#3900,#3901));
#983=EDGE_LOOP('',(#3902,#3903,#3904,#3905,#3906));
#984=EDGE_LOOP('',(#3907,#3908,#3909,#3910));
#985=EDGE_LOOP('',(#3911,#3912,#3913,#3914));
#986=EDGE_LOOP('',(#3915,#3916,#3917,#3918));
#987=EDGE_LOOP('',(#3919,#3920,#3921,#3922));
#988=EDGE_LOOP('',(#3923,#3924,#3925,#3926));
#989=EDGE_LOOP('',(#3927,#3928,#3929,#3930));
#990=EDGE_LOOP('',(#3931,#3932,#3933,#3934));
#991=EDGE_LOOP('',(#3935,#3936,#3937,#3938));
#992=EDGE_LOOP('',(#3939,#3940,#3941,#3942));
#1068=LINE('',#26046,#1205);
#1069=LINE('',#26112,#1206);
#1070=LINE('',#26503,#1207);
#1071=LINE('',#26969,#1208);
#1072=LINE('',#27435,#1209);
#1073=LINE('',#27755,#1210);
#1074=LINE('',#28145,#1211);
#1075=LINE('',#28611,#1212);
#1076=LINE('',#29077,#1213);
#1077=LINE('',#33533,#1214);
#1078=LINE('',#33665,#1215);
#1079=LINE('',#33722,#1216);
#1080=LINE('',#33726,#1217);
#1081=LINE('',#33729,#1218);
#1082=LINE('',#33732,#1219);
#1083=LINE('',#33736,#1220);
#1084=LINE('',#33740,#1221);
#1085=LINE('',#33743,#1222);
#1086=LINE('',#33746,#1223);
#1087=LINE('',#33934,#1224);
#1088=LINE('',#33937,#1225);
#1089=LINE('',#33940,#1226);
#1090=LINE('',#33944,#1227);
#1091=LINE('',#33948,#1228);
#1092=LINE('',#33952,#1229);
#1093=LINE('',#33956,#1230);
#1094=LINE('',#33960,#1231);
#1095=LINE('',#33964,#1232);
#1096=LINE('',#33968,#1233);
#1097=LINE('',#33972,#1234);
#1098=LINE('',#33976,#1235);
#1099=LINE('',#33980,#1236);
#1100=LINE('',#33984,#1237);
#1101=LINE('',#33988,#1238);
#1102=LINE('',#34166,#1239);
#1103=LINE('',#34169,#1240);
#1104=LINE('',#34171,#1241);
#1105=LINE('',#34173,#1242);
#1106=LINE('',#34175,#1243);
#1107=LINE('',#34177,#1244);
#1108=LINE('',#34179,#1245);
#1109=LINE('',#34181,#1246);
#1110=LINE('',#34183,#1247);
#1111=LINE('',#34185,#1248);
#1112=LINE('',#34187,#1249);
#1113=LINE('',#34189,#1250);
#1114=LINE('',#34191,#1251);
#1115=LINE('',#34219,#1252);
#1116=LINE('',#34227,#1253);
#1117=LINE('',#34229,#1254);
#1118=LINE('',#34231,#1255);
#1119=LINE('',#34233,#1256);
#1120=LINE('',#34235,#1257);
#1121=LINE('',#34237,#1258);
#1122=LINE('',#34239,#1259);
#1123=LINE('',#34241,#1260);
#1205=VECTOR('',#5311,4.085);
#1206=VECTOR('',#5316,4.085);
#1207=VECTOR('',#5319,4.085);
#1208=VECTOR('',#5322,4.085);
#1209=VECTOR('',#5325,4.085);
#1210=VECTOR('',#5328,4.085);
#1211=VECTOR('',#5331,4.085);
#1212=VECTOR('',#5334,4.085);
#1213=VECTOR('',#5337,4.085);
#1214=VECTOR('',#5358,5.);
#1215=VECTOR('',#5367,5.);
#1216=VECTOR('',#5370,10.);
#1217=VECTOR('',#5373,10.);
#1218=VECTOR('',#5376,10.);
#1219=VECTOR('',#5379,10.);
#1220=VECTOR('',#5384,10.);
#1221=VECTOR('',#5387,10.);
#1222=VECTOR('',#5390,10.);
#1223=VECTOR('',#5393,10.);
#1224=VECTOR('',#5648,10.);
#1225=VECTOR('',#5651,10.);
#1226=VECTOR('',#5654,10.);
#1227=VECTOR('',#5659,10.);
#1228=VECTOR('',#5664,10.);
#1229=VECTOR('',#5669,10.);
#1230=VECTOR('',#5674,10.);
#1231=VECTOR('',#5679,10.);
#1232=VECTOR('',#5684,10.);
#1233=VECTOR('',#5689,10.);
#1234=VECTOR('',#5694,10.);
#1235=VECTOR('',#5699,10.);
#1236=VECTOR('',#5704,10.);
#1237=VECTOR('',#5709,10.);
#1238=VECTOR('',#5714,10.);
#1239=VECTOR('',#5963,10.);
#1240=VECTOR('',#5968,10.);
#1241=VECTOR('',#5971,10.);
#1242=VECTOR('',#5974,10.);
#1243=VECTOR('',#5977,10.);
#1244=VECTOR('',#5980,10.);
#1245=VECTOR('',#5983,10.);
#1246=VECTOR('',#5986,10.);
#1247=VECTOR('',#5989,10.);
#1248=VECTOR('',#5992,10.);
#1249=VECTOR('',#5995,10.);
#1250=VECTOR('',#5998,10.);
#1251=VECTOR('',#6001,10.);
#1252=VECTOR('',#6032,28.);
#1253=VECTOR('',#6045,1.5);
#1254=VECTOR('',#6048,1.5);
#1255=VECTOR('',#6051,1.5);
#1256=VECTOR('',#6054,1.5);
#1257=VECTOR('',#6057,1.5);
#1258=VECTOR('',#6060,1.5);
#1259=VECTOR('',#6063,1.5);
#1260=VECTOR('',#6066,1.5);
#1470=B_SPLINE_CURVE_WITH_KNOTS('',3,(#26048,#26049,#26050,#26051),
 .UNSPECIFIED.,.F.,.F.,(4,4),(68.198771421486,69.1672389387709),
 .UNSPECIFIED.);
#1471=B_SPLINE_CURVE_WITH_KNOTS('',3,(#26054,#26055,#26056,#26057,#26058,
#26059,#26060,#26061,#26062,#26063,#26064,#26065,#26066,#26067,#26068,#26069,
#26070,#26071,#26072,#26073,#26074,#26075,#26076,#26077,#26078,#26079,#26080,
#26081,#26082,#26083,#26084,#26085,#26086,#26087,#26088,#26089,#26090,#26091,
#26092,#26093,#26094,#26095,#26096,#26097,#26098,#26099,#26100,#26101,#26102,
#26103,#26104,#26105,#26106,#26107,#26108),.UNSPECIFIED.,.F.,.F.,(4,3,3,
3,3,3,3,3,3,3,3,3,3,3,3,3,3,3,4),(68.1990165158139,68.2867039372834,68.3743981543787,
68.4621196239386,68.5499348194578,68.6378063115861,68.7257986904822,68.744531877364,
68.8318666265745,68.9190930016561,69.0062345365395,69.0933171048388,69.1803688850522,
69.2674110254065,69.354464662252,69.4416035010195,69.5287857172442,69.6161043390497,
69.6911556575798),.UNSPECIFIED.);
#1472=B_SPLINE_CURVE_WITH_KNOTS('',3,(#26114,#26115,#26116,#26117,#26118,
#26119,#26120,#26121,#26122,#26123,#26124,#26125,#26126,#26127,#26128,#26129,
#26130,#26131,#26132,#26133,#26134,#26135,#26136,#26137,#26138,#26139,#26140,
#26141,#26142,#26143,#26144,#26145,#26146,#26147,#26148,#26149,#26150,#26151,
#26152,#26153,#26154,#26155,#26156,#26157,#26158,#26159,#26160,#26161,#26162,
#26163,#26164,#26165,#26166,#26167,#26168,#26169,#26170,#26171,#26172,#26173,
#26174,#26175,#26176,#26177,#26178,#26179,#26180,#26181,#26182,#26183,#26184,
#26185,#26186,#26187,#26188,#26189,#26190,#26191,#26192,#26193,#26194,#26195,
#26196,#26197,#26198,#26199,#26200,#26201,#26202,#26203,#26204,#26205,#26206,
#26207,#26208,#26209,#26210,#26211,#26212,#26213,#26214,#26215,#26216,#26217,
#26218,#26219,#26220,#26221,#26222,#26223,#26224,#26225,#26226,#26227,#26228,
#26229,#26230,#26231,#26232,#26233,#26234,#26235,#26236,#26237,#26238,#26239,
#26240,#26241,#26242,#26243,#26244,#26245,#26246,#26247,#26248,#26249,#26250,
#26251,#26252,#26253,#26254,#26255,#26256,#26257,#26258,#26259,#26260,#26261),
 .UNSPECIFIED.,.F.,.F.,(4,3,3,3,3,3,3,3,3,3,3,3,3,3,3,3,3,3,3,3,3,3,3,3,
3,3,3,3,3,3,3,3,3,3,3,3,3,3,3,3,3,3,3,3,3,3,3,3,3,4),(61.9152074670456,
62.0028392502741,62.0905179625085,62.1783353503388,62.2505508730523,62.3384131475251,
62.4261650959704,62.5138296608294,62.6044320992451,62.6919987313428,62.779552535813,
62.8671141164615,62.9547040775598,63.0423902308967,63.1301338862199,63.2180014802831,
63.2386491681549,63.3265146658182,63.4142701282254,63.5019384895468,63.5925396112606,
63.6801107100817,63.7676692197789,63.8552357377434,63.9428308619984,64.0305224830768,
64.1182717900469,64.2061452583331,64.2267474632576,64.3144870789918,64.4021162042687,
64.4896579267435,64.5803064056956,64.6677509157514,64.7551830721912,64.8426236080885,
64.9300932575184,65.0176607782296,65.1052866424268,65.1930385556437,65.2148457583603,
65.3017898443855,65.3885981523834,65.4753288625677,65.5620035755417,65.6486438406302,
65.7352974265419,65.8219556596735,65.9086836728027,65.9734457253856),
 .UNSPECIFIED.);
#1473=B_SPLINE_CURVE_WITH_KNOTS('',3,(#26262,#26263,#26264,#26265,#26266,
#26267,#26268),.UNSPECIFIED.,.F.,.F.,(4,1,1,1,4),(65.9734462067016,66.2029440534629,
67.1910423485656,68.1791406436682,68.198771421486),.UNSPECIFIED.);
#1474=B_SPLINE_CURVE_WITH_KNOTS('',3,(#26270,#26271,#26272,#26273,#26274,
#26275,#26276,#26277,#26278,#26279,#26280,#26281,#26282,#26283,#26284,#26285,
#26286,#26287,#26288,#26289,#26290,#26291,#26292,#26293,#26294,#26295,#26296,
#26297,#26298,#26299,#26300,#26301,#26302,#26303,#26304,#26305,#26306,#26307,
#26308,#26309,#26310,#26311,#26312,#26313,#26314,#26315,#26316,#26317,#26318,
#26319,#26320,#26321,#26322,#26323,#26324,#26325,#26326,#26327,#26328,#26329,
#26330,#26331,#26332,#26333,#26334,#26335,#26336,#26337,#26338,#26339,#26340,
#26341,#26342,#26343,#26344,#26345,#26346,#26347,#26348,#26349,#26350,#26351),
 .UNSPECIFIED.,.F.,.F.,(4,3,3,3,3,3,3,3,3,3,3,3,3,3,3,3,3,3,3,3,3,3,3,3,
3,3,3,4),(65.9734457255614,66.0599244006815,66.1484757614912,66.2348343901556,
66.3211731338775,66.4075137224388,66.4977191136188,66.5841760425287,66.6706891415639,
66.7573212530809,66.7683352871587,66.8560751038854,66.9437044304637,67.0312463543199,
67.1218947578126,67.2093394682341,67.2967718243368,67.3842125589907,67.4716824060662,
67.5592501218174,67.6468761797695,67.7346282834129,67.7564335822614,67.8444394353351,
67.9330837054548,68.0208783079558,68.1099474118848,68.1990165158139),
 .UNSPECIFIED.);
#1475=B_SPLINE_CURVE_WITH_KNOTS('',3,(#26352,#26353,#26354,#26355,#26356,
#26357,#26358,#26359,#26360,#26361,#26362,#26363,#26364,#26365,#26366,#26367,
#26368,#26369,#26370,#26371,#26372,#26373,#26374,#26375,#26376,#26377,#26378,
#26379,#26380,#26381,#26382,#26383,#26384,#26385,#26386,#26387,#26388,#26389,
#26390,#26391,#26392,#26393,#26394,#26395,#26396,#26397,#26398,#26399,#26400,
#26401,#26402,#26403,#26404,#26405,#26406,#26407,#26408,#26409,#26410,#26411,
#26412,#26413,#26414,#26415,#26416,#26417,#26418,#26419,#26420,#26421,#26422,
#26423,#26424,#26425,#26426,#26427,#26428,#26429,#26430,#26431,#26432,#26433,
#26434,#26435,#26436,#26437,#26438,#26439,#26440,#26441,#26442,#26443,#26444,
#26445,#26446,#26447,#26448,#26449,#26450,#26451,#26452,#26453,#26454,#26455,
#26456,#26457,#26458,#26459,#26460,#26461,#26462,#26463,#26464,#26465,#26466,
#26467,#26468,#26469,#26470,#26471,#26472,#26473,#26474,#26475,#26476,#26477,
#26478,#26479,#26480,#26481,#26482,#26483,#26484,#26485,#26486,#26487,#26488,
#26489,#26490,#26491,#26492,#26493,#26494,#26495,#26496,#26497,#26498,#26499),
 .UNSPECIFIED.,.F.,.F.,(4,3,3,3,3,3,3,3,3,3,3,3,3,3,3,3,3,3,3,3,3,3,3,3,
3,3,3,3,3,3,3,3,3,3,3,3,3,3,3,3,3,3,3,3,3,3,3,3,3,4),(61.9160292898655,
62.003765986239,62.0914154584642,62.1819812894997,62.2695333123404,62.3570727013311,
62.4446200755284,62.532196054615,62.6198685560932,62.7075987803768,62.7954531982411,
62.815942106748,62.9037916043167,62.9915308699443,63.0791828597822,63.1697900525408,
63.2573444543976,63.3448861767483,63.4324358359914,63.520014049116,63.6076887678098,
63.6954211583331,63.7832778180181,63.8040404018507,63.8918717835893,63.979592882304,
64.0672266762862,64.1578406788696,64.2453769286839,64.3329005466778,64.4204321688873,
64.5079924320004,64.5956494187184,64.6833641842158,64.7712035068591,64.7921386969534,
64.8800009524886,64.9677528821818,65.0554174284929,65.1460198739383,65.2335864881031,
65.3211402748971,65.4087018381435,65.4962917821319,65.5839779188708,65.6717215578754,
65.7595891361461,65.780236992056,65.9057469402362,65.9734457253856),
 .UNSPECIFIED.);
#1476=B_SPLINE_CURVE_WITH_KNOTS('',3,(#26505,#26506,#26507,#26508,#26509,
#26510,#26511,#26512,#26513,#26514,#26515,#26516,#26517,#26518,#26519,#26520,
#26521,#26522,#26523,#26524,#26525,#26526,#26527,#26528,#26529,#26530,#26531,
#26532,#26533,#26534,#26535,#26536,#26537,#26538,#26539,#26540,#26541,#26542,
#26543,#26544,#26545,#26546,#26547,#26548,#26549,#26550,#26551,#26552,#26553,
#26554,#26555,#26556,#26557,#26558,#26559,#26560,#26561,#26562,#26563,#26564,
#26565,#26566,#26567,#26568,#26569,#26570,#26571,#26572,#26573,#26574,#26575,
#26576,#26577,#26578,#26579,#26580,#26581,#26582,#26583,#26584,#26585,#26586,
#26587,#26588,#26589,#26590,#26591,#26592,#26593,#26594,#26595,#26596,#26597,
#26598,#26599,#26600,#26601,#26602,#26603,#26604,#26605,#26606,#26607,#26608,
#26609,#26610,#26611,#26612,#26613,#26614,#26615,#26616,#26617,#26618,#26619,
#26620,#26621,#26622,#26623,#26624,#26625,#26626,#26627,#26628,#26629,#26630,
#26631,#26632,#26633,#26634,#26635,#26636,#26637,#26638,#26639,#26640,#26641,
#26642,#26643,#26644,#26645,#26646,#26647,#26648,#26649,#26650,#26651,#26652),
 .UNSPECIFIED.,.F.,.F.,(4,3,3,3,3,3,3,3,3,3,3,3,3,3,3,3,3,3,3,3,3,3,3,3,
3,3,3,3,3,3,3,3,3,3,3,3,3,3,3,3,3,3,3,3,3,3,3,3,3,4),(55.6329415823545,
55.7205103087394,55.8080534505669,55.8955916358262,55.9831454839555,56.0707895120438,
56.1584796275128,56.2463091812715,56.3219611024363,56.4098069678268,56.4975425704886,
56.5851908713359,56.6757994371112,56.7633501093486,56.8508880936569,56.9384340105917,
57.0260084812995,57.1136794763125,57.2014081498481,57.2892611303658,57.3100593975389,
57.3979057700926,57.4856418852267,57.5732907031754,57.6638990768587,57.7514502743065,
57.8389887858891,57.9265352315721,58.014110231911,58.1017817551768,58.1895109567624,
58.2773644610362,58.2981576926416,58.3860015379222,58.4737351205031,58.5613814036833,
58.6519907266909,58.7395393999614,58.8270753956588,58.9146193364734,59.0021918456963,
59.0898609105614,59.1775876700309,59.265438774201,59.2862559877443,59.3872570953136,
59.4837999140162,59.5800852540891,59.6759906400734,59.6902604180213),
 .UNSPECIFIED.);
#1477=B_SPLINE_CURVE_WITH_KNOTS('',3,(#26653,#26654,#26655,#26656,#26657,
#26658,#26659,#26660,#26661,#26662,#26663,#26664,#26665,#26666,#26667,#26668,
#26669,#26670,#26671,#26672,#26673,#26674,#26675,#26676,#26677,#26678,#26679,
#26680,#26681,#26682,#26683,#26684,#26685,#26686,#26687,#26688,#26689,#26690,
#26691,#26692,#26693,#26694,#26695,#26696,#26697,#26698,#26699,#26700,#26701,
#26702,#26703,#26704,#26705,#26706,#26707,#26708,#26709,#26710,#26711,#26712,
#26713,#26714,#26715,#26716,#26717,#26718,#26719,#26720,#26721,#26722,#26723,
#26724,#26725,#26726,#26727,#26728,#26729,#26730,#26731,#26732,#26733,#26734),
 .UNSPECIFIED.,.F.,.F.,(4,3,3,3,3,3,3,3,3,3,3,3,3,3,3,3,3,3,3,3,3,3,3,3,
3,3,3,4),(59.6902604182061,59.7791601363368,59.8680903388289,59.9570692322848,
60.0461757616844,60.1353527655857,60.2246849720358,60.2743542828469,60.362203797533,
60.4499430803699,60.5375950874869,60.6282022737948,60.715756692995,60.8032984326827,
60.8908481092374,60.978426339629,61.0661010754383,61.153833483008,61.2416901595109,
61.2624525779496,61.350268063159,61.4379804811472,61.525610640487,61.6131792828027,
61.7007144613418,61.7882299492699,61.875765618165,61.9152074670456),
 .UNSPECIFIED.);
#1478=B_SPLINE_CURVE_WITH_KNOTS('',3,(#26736,#26737,#26738,#26739,#26740,
#26741,#26742,#26743,#26744,#26745,#26746,#26747,#26748,#26749,#26750,#26751,
#26752,#26753,#26754,#26755,#26756,#26757,#26758,#26759,#26760,#26761,#26762,
#26763,#26764,#26765,#26766,#26767,#26768,#26769,#26770,#26771,#26772,#26773,
#26774,#26775,#26776,#26777,#26778,#26779,#26780,#26781,#26782,#26783,#26784,
#26785,#26786,#26787,#26788,#26789,#26790,#26791,#26792,#26793,#26794,#26795,
#26796,#26797,#26798,#26799,#26800,#26801,#26802,#26803,#26804,#26805,#26806,
#26807,#26808,#26809,#26810,#26811,#26812,#26813,#26814,#26815,#26816,#26817),
 .UNSPECIFIED.,.F.,.F.,(4,3,3,3,3,3,3,3,3,3,3,3,3,3,3,3,3,3,3,3,3,3,3,3,
3,3,3,4),(59.6902604182061,59.8288576938286,59.85164722144,59.9394935907456,
60.0272297026167,60.114878517291,60.2054868921975,60.2930380863645,60.3805765946698,
60.4681230370823,60.5556980341614,60.6433695541988,60.7310987525705,60.8189522536764,
60.8397455165427,60.9275893686412,61.0153229580445,61.1029692480439,61.1935785684941,
61.2811272485317,61.3686632509655,61.4562071984788,61.5437797143553,61.6314487857747,
61.7191755517482,61.8070266623,61.8278438116454,61.9160292898655),
 .UNSPECIFIED.);
#1479=B_SPLINE_CURVE_WITH_KNOTS('',3,(#26818,#26819,#26820,#26821,#26822,
#26823,#26824,#26825,#26826,#26827,#26828,#26829,#26830,#26831,#26832,#26833,
#26834,#26835,#26836,#26837,#26838,#26839,#26840,#26841,#26842,#26843,#26844,
#26845,#26846,#26847,#26848,#26849,#26850,#26851,#26852,#26853,#26854,#26855,
#26856,#26857,#26858,#26859,#26860,#26861,#26862,#26863,#26864,#26865,#26866,
#26867,#26868,#26869,#26870,#26871,#26872,#26873,#26874,#26875,#26876,#26877,
#26878,#26879,#26880,#26881,#26882,#26883,#26884,#26885,#26886,#26887,#26888,
#26889,#26890,#26891,#26892,#26893,#26894,#26895,#26896,#26897,#26898,#26899,
#26900,#26901,#26902,#26903,#26904,#26905,#26906,#26907,#26908,#26909,#26910,
#26911,#26912,#26913,#26914,#26915,#26916,#26917,#26918,#26919,#26920,#26921,
#26922,#26923,#26924,#26925,#26926,#26927,#26928,#26929,#26930,#26931,#26932,
#26933,#26934,#26935,#26936,#26937,#26938,#26939,#26940,#26941,#26942,#26943,
#26944,#26945,#26946,#26947,#26948,#26949,#26950,#26951,#26952,#26953,#26954,
#26955,#26956,#26957,#26958,#26959,#26960,#26961,#26962,#26963,#26964,#26965),
 .UNSPECIFIED.,.F.,.F.,(4,3,3,3,3,3,3,3,3,3,3,3,3,3,3,3,3,3,3,3,3,3,3,3,
3,3,3,3,3,3,3,3,3,3,3,3,3,3,3,3,3,3,3,3,3,3,3,3,3,4),(55.6319201599848,
55.7196005837777,55.8094273124036,55.8992540410294,55.9870997806171,56.0748352588762,
56.162483436848,56.2530920492585,56.3406426031537,56.4281804709919,56.5157262734477,
56.603300631787,56.6909715180913,56.7787000849292,56.8665529624602,56.8873523361321,
56.9751981693186,57.0629337418575,57.1505820146696,57.2411905917402,57.3287412412526,
57.4162792048268,57.5038251030318,57.591399557027,57.6790705383681,57.7667991999897,
57.8546521712214,57.8754506312347,57.9632961259926,58.051031359628,58.1386792934676,
58.2292879975763,58.3168383100931,58.4043759379858,58.4919215021854,58.5794956242163,
58.6671662782576,58.7548946149278,58.8427472670603,58.8635489263374,58.9501115740607,
59.0365644100789,59.1229218421432,59.2092266551714,59.2955006634414,59.3817656498755,
59.4680807244374,59.554422813523,59.6408625970588,59.6902604180514),
 .UNSPECIFIED.);
#1480=B_SPLINE_CURVE_WITH_KNOTS('',3,(#26971,#26972,#26973,#26974,#26975,
#26976,#26977,#26978,#26979,#26980,#26981,#26982,#26983,#26984,#26985,#26986,
#26987,#26988,#26989,#26990,#26991,#26992,#26993,#26994,#26995,#26996,#26997,
#26998,#26999,#27000,#27001,#27002,#27003,#27004,#27005,#27006,#27007,#27008,
#27009,#27010,#27011,#27012,#27013,#27014,#27015,#27016,#27017,#27018,#27019,
#27020,#27021,#27022,#27023,#27024,#27025,#27026,#27027,#27028,#27029,#27030,
#27031,#27032,#27033,#27034,#27035,#27036,#27037,#27038,#27039,#27040,#27041,
#27042,#27043,#27044,#27045,#27046,#27047,#27048,#27049,#27050,#27051,#27052,
#27053,#27054,#27055,#27056,#27057,#27058,#27059,#27060,#27061,#27062,#27063,
#27064,#27065,#27066,#27067,#27068,#27069,#27070,#27071,#27072,#27073,#27074,
#27075,#27076,#27077,#27078,#27079,#27080,#27081,#27082,#27083,#27084,#27085,
#27086,#27087,#27088,#27089,#27090,#27091,#27092,#27093,#27094,#27095,#27096,
#27097,#27098,#27099,#27100,#27101,#27102,#27103,#27104,#27105,#27106,#27107,
#27108,#27109,#27110,#27111,#27112,#27113,#27114,#27115,#27116,#27117,#27118,
#27119,#27120,#27121),.UNSPECIFIED.,.F.,.F.,(4,3,3,3,3,3,3,3,3,3,3,3,3,
3,3,3,3,3,3,3,3,3,3,3,3,3,3,3,3,3,3,3,3,3,3,3,3,3,3,3,3,3,3,3,3,3,3,3,3,
3,4),(49.3489872945652,49.4052730367176,49.4931187667722,49.5808542357431,
49.6685024046791,49.7591110205717,49.8466615661085,49.9341994258518,50.0217452204837,
50.109319571278,50.1969904504838,50.2847190104756,50.3725718815769,50.3933713318203,
50.4812170646052,50.5689525362668,50.6566007078512,50.7472093227352,50.8347598707998,
50.9222977330224,51.0098435300823,51.0974178832511,51.1850887647406,51.2728173269658,
51.3606702002109,51.381469626923,51.4693153753648,51.5570508627688,51.6446990501612,
51.7353076591443,51.8228582230782,51.9103961011649,51.9979419140664,52.0855162830366,
52.1731871801893,52.2609157580148,52.3487686466512,52.3695679220256,52.4574136261298,
52.5451490691642,52.6327972122078,52.7234058378229,52.8109563577401,52.8984941920087,
52.9860399613381,53.0736142870294,53.1612851415514,53.2490136770757,53.3368665242072,
53.3576662171283,53.4070751110265),.UNSPECIFIED.);
#1481=B_SPLINE_CURVE_WITH_KNOTS('',3,(#27122,#27123,#27124,#27125,#27126,
#27127,#27128,#27129,#27130,#27131,#27132,#27133,#27134,#27135,#27136,#27137,
#27138,#27139,#27140,#27141,#27142,#27143,#27144,#27145,#27146,#27147,#27148,
#27149,#27150,#27151,#27152,#27153,#27154,#27155,#27156,#27157,#27158,#27159,
#27160,#27161,#27162,#27163,#27164,#27165,#27166,#27167,#27168,#27169,#27170,
#27171,#27172,#27173,#27174,#27175,#27176,#27177,#27178,#27179,#27180,#27181,
#27182,#27183,#27184,#27185,#27186,#27187,#27188,#27189,#27190,#27191,#27192,
#27193,#27194,#27195,#27196,#27197,#27198,#27199,#27200,#27201,#27202,#27203),
 .UNSPECIFIED.,.F.,.F.,(4,3,3,3,3,3,3,3,3,3,3,3,3,3,3,3,3,3,3,3,3,3,3,3,
3,3,3,4),(53.4070751111794,53.4942487792892,53.581315479733,53.6682989026037,
53.7552259023249,53.8421238514233,53.9290140393189,54.0159177450201,54.102908698297,
54.1899450618072,54.2771175328094,54.345764512231,54.4336103459984,54.5213459191207,
54.6089941925175,54.6996027693695,54.7871534194668,54.8746913836249,54.9622372824117,
55.0498117369875,55.1374827189024,55.2252113810947,55.3130643528886,55.3338628073336,
55.4216973721277,55.5094350678335,55.5970786676283,55.6329415823545),
 .UNSPECIFIED.);
#1482=B_SPLINE_CURVE_WITH_KNOTS('',3,(#27205,#27206,#27207,#27208,#27209,
#27210,#27211,#27212,#27213,#27214,#27215,#27216,#27217,#27218,#27219,#27220,
#27221,#27222,#27223,#27224,#27225,#27226,#27227,#27228,#27229,#27230,#27231,
#27232,#27233,#27234,#27235,#27236,#27237,#27238,#27239,#27240,#27241,#27242,
#27243,#27244,#27245,#27246,#27247,#27248,#27249,#27250,#27251,#27252,#27253,
#27254,#27255,#27256,#27257,#27258,#27259,#27260,#27261,#27262,#27263,#27264,
#27265,#27266,#27267,#27268,#27269,#27270,#27271,#27272,#27273,#27274,#27275,
#27276,#27277,#27278,#27279,#27280,#27281,#27282,#27283,#27284,#27285,#27286),
 .UNSPECIFIED.,.F.,.F.,(4,3,3,3,3,3,3,3,3,3,3,3,3,3,3,3,3,3,3,3,3,3,3,3,
3,3,3,4),(53.4070751110265,53.4979084720332,53.5888357596706,53.6799484289355,
53.7711596831757,53.8625643336905,53.9230574508241,54.0109031991677,54.0986386864732,
54.186286873767,54.276895482787,54.3644460466224,54.4519839246107,54.5395297374141,
54.6271041062866,54.7147750033428,54.8025035810724,54.8903564696145,54.9111557459267,
55.001251297684,55.0889717707487,55.176611913228,55.2641924455928,55.3561243741908,
55.4436628150252,55.5312019731037,55.61878222435,55.6319201599848),
 .UNSPECIFIED.);
#1483=B_SPLINE_CURVE_WITH_KNOTS('',3,(#27287,#27288,#27289,#27290,#27291,
#27292,#27293,#27294,#27295,#27296,#27297,#27298,#27299,#27300,#27301,#27302,
#27303,#27304,#27305,#27306,#27307,#27308,#27309,#27310,#27311,#27312,#27313,
#27314,#27315,#27316,#27317,#27318,#27319,#27320,#27321,#27322,#27323,#27324,
#27325,#27326,#27327,#27328,#27329,#27330,#27331,#27332,#27333,#27334,#27335,
#27336,#27337,#27338,#27339,#27340,#27341,#27342,#27343,#27344,#27345,#27346,
#27347,#27348,#27349,#27350,#27351,#27352,#27353,#27354,#27355,#27356,#27357,
#27358,#27359,#27360,#27361,#27362,#27363,#27364,#27365,#27366,#27367,#27368,
#27369,#27370,#27371,#27372,#27373,#27374,#27375,#27376,#27377,#27378,#27379,
#27380,#27381,#27382,#27383,#27384,#27385,#27386,#27387,#27388,#27389,#27390,
#27391,#27392,#27393,#27394,#27395,#27396,#27397,#27398,#27399,#27400,#27401,
#27402,#27403,#27404,#27405,#27406,#27407,#27408,#27409,#27410,#27411,#27412,
#27413,#27414,#27415,#27416,#27417,#27418,#27419,#27420,#27421,#27422,#27423,
#27424,#27425,#27426,#27427,#27428,#27429,#27430,#27431),.UNSPECIFIED.,
 .F.,.F.,(4,3,3,3,3,3,3,3,3,3,3,3,3,3,3,3,3,3,3,3,3,3,3,3,3,3,3,3,3,3,3,
3,3,3,3,3,3,3,3,3,3,3,3,3,3,3,3,3,4),(49.3496195384547,49.4371668507027,
49.5247045899421,49.612253376003,49.7018560996056,49.7895356797267,49.8800999750701,
49.9706642704134,50.0585100036378,50.1462454757683,50.2338936478499,50.3245022625582,
50.4120528111866,50.4995906739965,50.5871364716665,50.6747108254672,50.7623817076176,
50.8501102705212,50.9379631444655,50.9587625655161,51.0466083011504,51.134343775701,
51.2219919502098,51.3126005640109,51.4001511150689,51.487688980305,51.5752347803949,
51.6628091366067,51.7504800211437,51.8382085864225,51.9260614627063,51.9468608606187,
52.0347065906943,52.1224420596861,52.2100902286431,52.3006988445279,52.3882493900852,
52.4757872498489,52.5633330445013,52.650907395315,52.7385782745406,52.8263068345526,
52.9141597056729,52.9349591557214,53.0281706542195,53.1228967683669,53.2156926069346,
53.311383858872,53.4070751108094),.UNSPECIFIED.);
#1484=B_SPLINE_CURVE_WITH_KNOTS('',3,(#27437,#27438,#27439,#27440,#27441,
#27442,#27443,#27444),.UNSPECIFIED.,.F.,.F.,(4,1,1,1,1,4),(43.0656672236125,
43.4766832661016,44.4647815612043,45.452879856307,46.4409781514096,47.1238898038469),
 .UNSPECIFIED.);
#1485=B_SPLINE_CURVE_WITH_KNOTS('',3,(#27445,#27446,#27447,#27448,#27449,
#27450,#27451,#27452,#27453,#27454,#27455,#27456,#27457,#27458,#27459,#27460,
#27461,#27462,#27463,#27464,#27465,#27466,#27467,#27468,#27469,#27470,#27471,
#27472,#27473,#27474,#27475,#27476,#27477,#27478,#27479,#27480,#27481,#27482,
#27483,#27484,#27485,#27486,#27487,#27488,#27489,#27490,#27491,#27492,#27493,
#27494,#27495,#27496,#27497,#27498,#27499,#27500,#27501,#27502,#27503,#27504,
#27505,#27506,#27507,#27508,#27509,#27510,#27511,#27512,#27513,#27514,#27515,
#27516,#27517,#27518,#27519,#27520,#27521,#27522,#27523),.UNSPECIFIED.,
 .F.,.F.,(4,3,3,3,3,3,3,3,3,3,3,3,3,3,3,3,3,3,3,3,3,3,3,3,3,3,4),(47.1238899834251,
47.2279237124283,47.3331422464939,47.4290764465123,47.5169221797334,47.6046576518605,
47.6923058239389,47.7829144386485,47.8704649872736,47.9580028500801,48.0455486477467,
48.1331230015439,48.2207938836911,48.3085224465917,48.3963753205325,48.417174741615,
48.5050237765636,48.5927617437342,48.6804116075757,48.7679951400718,48.8555434981,
48.9430773171428,49.0306172170903,49.1182278887984,49.2058765988617,49.2936398438844,
49.3489872945652),.UNSPECIFIED.);
#1486=B_SPLINE_CURVE_WITH_KNOTS('',3,(#27525,#27526,#27527,#27528,#27529,
#27530,#27531,#27532,#27533,#27534,#27535,#27536,#27537,#27538,#27539,#27540,
#27541,#27542,#27543,#27544,#27545,#27546,#27547,#27548,#27549,#27550,#27551,
#27552,#27553,#27554,#27555,#27556,#27557,#27558,#27559,#27560,#27561,#27562,
#27563,#27564,#27565,#27566,#27567,#27568,#27569,#27570,#27571,#27572,#27573,
#27574,#27575,#27576,#27577,#27578,#27579,#27580,#27581,#27582,#27583,#27584,
#27585,#27586,#27587,#27588,#27589,#27590,#27591,#27592,#27593,#27594,#27595,
#27596,#27597,#27598,#27599,#27600,#27601,#27602,#27603,#27604,#27605,#27606),
 .UNSPECIFIED.,.F.,.F.,(4,3,3,3,3,3,3,3,3,3,3,3,3,3,3,3,3,3,3,3,3,3,3,3,
3,3,3,4),(47.1238898040527,47.210492156019,47.2969993784341,47.3841829161559,
47.4705790288969,47.5569581549671,47.6433419919605,47.7311234140224,47.8176268261185,
47.9060472531633,47.9944676802081,48.0823134140176,48.1700488867384,48.2576970594146,
48.3483056739016,48.4358562231318,48.5233940865448,48.6109398848189,48.6985142392238,
48.7861851219757,48.8739136854801,48.9617665600191,48.9825659753107,49.0743293660967,
49.162052739274,49.2496992777742,49.3372797397587,49.3496195384547),
 .UNSPECIFIED.);
#1487=B_SPLINE_CURVE_WITH_KNOTS('',3,(#27607,#27608,#27609,#27610,#27611,
#27612,#27613,#27614,#27615,#27616,#27617,#27618,#27619,#27620,#27621,#27622,
#27623,#27624,#27625,#27626,#27627,#27628,#27629,#27630,#27631,#27632,#27633,
#27634,#27635,#27636,#27637,#27638,#27639,#27640,#27641,#27642,#27643,#27644,
#27645,#27646,#27647,#27648,#27649,#27650,#27651,#27652,#27653,#27654,#27655,
#27656,#27657,#27658,#27659,#27660,#27661,#27662,#27663,#27664,#27665,#27666,
#27667,#27668,#27669,#27670,#27671,#27672,#27673,#27674,#27675,#27676,#27677,
#27678,#27679,#27680,#27681,#27682,#27683,#27684,#27685,#27686,#27687,#27688,
#27689,#27690,#27691,#27692,#27693,#27694,#27695,#27696,#27697,#27698,#27699,
#27700,#27701,#27702,#27703,#27704,#27705,#27706,#27707,#27708,#27709,#27710,
#27711,#27712,#27713,#27714,#27715,#27716,#27717,#27718,#27719,#27720,#27721,
#27722,#27723,#27724,#27725,#27726,#27727,#27728,#27729,#27730,#27731,#27732,
#27733,#27734,#27735,#27736,#27737,#27738,#27739,#27740,#27741,#27742,#27743,
#27744,#27745,#27746,#27747,#27748,#27749,#27750,#27751),.UNSPECIFIED.,
 .F.,.F.,(4,3,3,3,3,3,3,3,3,3,3,3,3,3,3,3,3,3,3,3,3,3,3,3,3,3,3,3,3,3,3,
3,3,3,3,3,3,3,3,3,3,3,3,3,3,3,3,3,4),(43.0661513688595,43.1539804562812,
43.2417024687189,43.3293403545273,43.4184321226861,43.505980034342,43.5935177611447,
43.6810659230641,43.7713180672474,43.8589965048089,43.9505355023032,44.0420744997974,
44.1299202333019,44.217655705717,44.3053038780874,44.395912492689,44.4834630416144,
44.5710009047237,44.6585467026954,44.7461210567996,44.8337919392548,44.9215205024643,
45.0093733767133,45.0301727949001,45.1180185284566,45.2057540009238,45.2934021733465,
45.3840107879285,45.471561336906,45.5590992000672,45.6466449980905,45.7342193522462,
45.8218902347522,45.9096187980123,45.997471672311,46.0182710900028,46.1061168234813,
46.1938522958706,46.2815004682155,46.3721090828267,46.4596596317277,46.5471974948129,
46.6347432927609,46.7223176468418,46.8099885292745,46.8977170924621,46.9855699666899,
47.0063693851054,47.1238898038469),.UNSPECIFIED.);
#1488=B_SPLINE_CURVE_WITH_KNOTS('',3,(#27757,#27758,#27759,#27760,#27761,
#27762,#27763,#27764,#27765,#27766,#27767,#27768,#27769,#27770,#27771,#27772,
#27773,#27774,#27775,#27776,#27777,#27778,#27779,#27780,#27781,#27782,#27783,
#27784,#27785,#27786,#27787,#27788,#27789,#27790,#27791,#27792,#27793,#27794,
#27795,#27796,#27797,#27798,#27799,#27800,#27801,#27802,#27803,#27804,#27805,
#27806,#27807,#27808,#27809,#27810,#27811,#27812,#27813,#27814,#27815,#27816,
#27817,#27818,#27819,#27820,#27821,#27822,#27823,#27824,#27825,#27826,#27827,
#27828,#27829,#27830,#27831,#27832,#27833,#27834,#27835,#27836,#27837,#27838,
#27839,#27840,#27841,#27842,#27843,#27844,#27845,#27846,#27847,#27848,#27849,
#27850,#27851,#27852,#27853,#27854,#27855,#27856,#27857,#27858,#27859,#27860,
#27861,#27862,#27863,#27864,#27865,#27866,#27867,#27868,#27869,#27870,#27871,
#27872,#27873,#27874,#27875,#27876,#27877,#27878,#27879,#27880,#27881,#27882,
#27883,#27884,#27885,#27886,#27887,#27888,#27889,#27890,#27891,#27892,#27893,
#27894,#27895,#27896,#27897,#27898,#27899,#27900,#27901,#27902,#27903,#27904),
 .UNSPECIFIED.,.F.,.F.,(4,3,3,3,3,3,3,3,3,3,3,3,3,3,3,3,3,3,3,3,3,3,3,3,
3,3,3,3,3,3,3,3,3,3,3,3,3,3,3,3,3,3,3,3,3,3,3,3,3,4),(36.7834594513572,
36.8710696055442,36.9586338461866,37.0461753273144,37.1337146746301,37.2212725072833,
37.308921977867,37.3966200728502,37.4844541454934,37.5480934954857,37.6359392290401,
37.7236747015056,37.811322873927,37.9019314885097,37.9894820374872,38.0770199006489,
38.1645656986731,38.2521400528301,38.3398109353381,38.4275394986005,38.5153923729021,
38.5361917905883,38.6240375240927,38.7117729965076,38.7994211688778,38.8900297834795,
38.9775803324048,39.0651181955139,39.1526639934854,39.2402383475895,39.3279092300444,
39.4156377932538,39.5034906675027,39.524290085691,39.6121358192108,39.6998712916411,
39.7875194640268,39.8781280786227,39.9656786275633,40.0532164906878,40.1407622886745,
40.2283366427937,40.3160075252636,40.4037360884876,40.491588962751,40.5123883807937,
40.6152734140351,40.7176836287931,40.819249582201,40.8407042874444),
 .UNSPECIFIED.);
#1489=B_SPLINE_CURVE_WITH_KNOTS('',3,(#27905,#27906,#27907,#27908,#27909,
#27910),.UNSPECIFIED.,.F.,.F.,(4,1,1,4),(40.8407044966673,41.5004866758963,
42.488584970999,43.0656672236125),.UNSPECIFIED.);
#1490=B_SPLINE_CURVE_WITH_KNOTS('',3,(#27912,#27913,#27914,#27915,#27916,
#27917,#27918,#27919,#27920,#27921,#27922,#27923,#27924,#27925,#27926,#27927,
#27928,#27929,#27930,#27931,#27932,#27933,#27934,#27935,#27936,#27937,#27938,
#27939,#27940,#27941,#27942,#27943,#27944,#27945,#27946,#27947,#27948,#27949,
#27950,#27951,#27952,#27953,#27954,#27955,#27956,#27957,#27958,#27959,#27960,
#27961,#27962,#27963,#27964,#27965,#27966,#27967,#27968,#27969,#27970,#27971,
#27972,#27973,#27974,#27975,#27976,#27977,#27978,#27979,#27980,#27981,#27982,
#27983,#27984,#27985,#27986,#27987,#27988,#27989,#27990,#27991,#27992,#27993),
 .UNSPECIFIED.,.F.,.F.,(4,3,3,3,3,3,3,3,3,3,3,3,3,3,3,3,3,3,3,3,3,3,3,3,
3,3,3,4),(40.840704496801,40.9592420556452,41.0777796144894,41.165625347994,
41.2533608204091,41.3410089927796,41.4316176073812,41.5191681563067,41.606706019416,
41.6942518173877,41.7818261714919,41.869497053947,41.9572256171564,42.0450784914055,
42.0658779095921,42.1537236431118,42.2414591155421,42.3291072879277,42.4197159025236,
42.5072664514642,42.5948043145885,42.6823501125752,42.7699244666943,42.8575953491641,
42.9453239123882,43.0331767866515,43.0539762046948,43.0661513688595),
 .UNSPECIFIED.);
#1491=B_SPLINE_CURVE_WITH_KNOTS('',3,(#27994,#27995,#27996,#27997,#27998,
#27999,#28000,#28001,#28002,#28003,#28004,#28005,#28006,#28007,#28008,#28009,
#28010,#28011,#28012,#28013,#28014,#28015,#28016,#28017,#28018,#28019,#28020,
#28021,#28022,#28023,#28024,#28025,#28026,#28027,#28028,#28029,#28030,#28031,
#28032,#28033,#28034,#28035,#28036,#28037,#28038,#28039,#28040,#28041,#28042,
#28043,#28044,#28045,#28046,#28047,#28048,#28049,#28050,#28051,#28052,#28053,
#28054,#28055,#28056,#28057,#28058,#28059,#28060,#28061,#28062,#28063,#28064,
#28065,#28066,#28067,#28068,#28069,#28070,#28071,#28072,#28073,#28074,#28075,
#28076,#28077,#28078,#28079,#28080,#28081,#28082,#28083,#28084,#28085,#28086,
#28087,#28088,#28089,#28090,#28091,#28092,#28093,#28094,#28095,#28096,#28097,
#28098,#28099,#28100,#28101,#28102,#28103,#28104,#28105,#28106,#28107,#28108,
#28109,#28110,#28111,#28112,#28113,#28114,#28115,#28116,#28117,#28118,#28119,
#28120,#28121,#28122,#28123,#28124,#28125,#28126,#28127,#28128,#28129,#28130,
#28131,#28132,#28133,#28134,#28135,#28136,#28137,#28138,#28139,#28140,#28141),
 .UNSPECIFIED.,.F.,.F.,(4,3,3,3,3,3,3,3,3,3,3,3,3,3,3,3,3,3,3,3,3,3,3,3,
3,3,3,3,3,3,3,3,3,3,3,3,3,3,3,3,3,3,3,3,3,3,3,3,3,4),(36.782489025435,36.8701315883539,
36.9578193726307,37.0456477851092,37.1253864340788,37.2132321678722,37.3009676405799,
37.388615813246,37.4792244277379,37.5667749769658,37.6543128403794,37.7418586386567,
37.8294329930681,37.9171038758305,38.004832439348,38.0926853139034,38.1134847291814,
38.2013304626339,38.2890659349965,38.3767141073143,38.4673227219356,38.5548732708085,
38.6424111338651,38.7299569317841,38.8175312858352,38.9052021682385,38.9929307313962,
39.0807836055944,39.1015830242841,39.1894287577675,39.2771642301606,39.3648124025089,
39.4554210171186,39.5429715660202,39.6305094291052,39.7180552270518,39.8056295811307,
39.8933004635602,39.9810290267434,40.0688819009665,40.0896813193868,40.1764746119568,
40.2631324614172,40.3497129319938,40.4362377296806,40.5227285080445,40.609232549189,
40.6957418296306,40.7823191590372,40.8407044966673),.UNSPECIFIED.);
#1492=B_SPLINE_CURVE_WITH_KNOTS('',3,(#28147,#28148,#28149,#28150,#28151,
#28152,#28153,#28154,#28155,#28156,#28157,#28158,#28159,#28160,#28161,#28162,
#28163,#28164,#28165,#28166,#28167,#28168,#28169,#28170,#28171,#28172,#28173,
#28174,#28175,#28176,#28177,#28178,#28179,#28180,#28181,#28182,#28183,#28184,
#28185,#28186,#28187,#28188,#28189,#28190,#28191,#28192,#28193,#28194,#28195,
#28196,#28197,#28198,#28199,#28200,#28201,#28202,#28203,#28204,#28205,#28206,
#28207,#28208,#28209,#28210,#28211,#28212,#28213,#28214,#28215,#28216,#28217,
#28218,#28219,#28220,#28221,#28222,#28223,#28224,#28225,#28226,#28227,#28228,
#28229,#28230,#28231,#28232,#28233,#28234,#28235,#28236,#28237,#28238,#28239,
#28240,#28241,#28242,#28243,#28244,#28245,#28246,#28247,#28248,#28249,#28250,
#28251,#28252,#28253,#28254,#28255,#28256,#28257,#28258,#28259,#28260,#28261,
#28262,#28263,#28264,#28265,#28266,#28267,#28268,#28269,#28270,#28271,#28272,
#28273,#28274,#28275,#28276,#28277,#28278,#28279,#28280,#28281,#28282,#28283,
#28284,#28285,#28286,#28287,#28288,#28289,#28290,#28291,#28292,#28293,#28294),
 .UNSPECIFIED.,.F.,.F.,(4,3,3,3,3,3,3,3,3,3,3,3,3,3,3,3,3,3,3,3,3,3,3,3,
3,3,3,3,3,3,3,3,3,3,3,3,3,3,3,3,3,3,3,3,3,3,3,3,3,4),(30.4992123502324,
30.5870542145733,30.631405429767,30.7192511601337,30.8069866293569,30.8946347984857,
30.9852434142837,31.0727939598643,31.1603318195962,31.2478776141616,31.3354519648342,
31.4231228438373,31.5108514035789,31.5987042743628,31.6195037248697,31.707349460417,
31.7950849349003,31.8827331093615,31.9733417231879,32.0608922742473,32.1484301395027,
32.2359759396303,32.3235502958981,32.4112211805172,32.4989497458933,32.5868026222967,
32.6076020199723,32.69544775317,32.7831832252783,32.8708313973422,32.9614400120588,
33.0489905606806,33.1365284234879,33.2240742211596,33.311648574966,33.3993194571285,
33.4870480200478,33.5749008940125,33.595700315075,33.6831656270259,33.7705208710584,
33.857789457399,33.9452556738879,34.0324300625443,34.1195929028326,34.2067652159563,
34.2944537092947,34.3817525654606,34.4696358773854,34.5575191893102),
 .UNSPECIFIED.);
#1493=B_SPLINE_CURVE_WITH_KNOTS('',3,(#28295,#28296,#28297,#28298,#28299,
#28300,#28301,#28302,#28303,#28304,#28305,#28306,#28307,#28308,#28309,#28310,
#28311,#28312,#28313,#28314,#28315,#28316,#28317,#28318,#28319,#28320,#28321,
#28322,#28323,#28324,#28325,#28326,#28327,#28328,#28329,#28330,#28331,#28332,
#28333,#28334,#28335,#28336,#28337,#28338,#28339,#28340,#28341,#28342,#28343,
#28344,#28345,#28346,#28347,#28348,#28349,#28350,#28351,#28352,#28353,#28354,
#28355,#28356,#28357,#28358,#28359,#28360,#28361,#28362,#28363,#28364,#28365,
#28366,#28367,#28368,#28369,#28370,#28371,#28372,#28373,#28374,#28375,#28376,
#28377,#28378,#28379),.UNSPECIFIED.,.F.,.F.,(4,3,3,3,3,3,3,3,3,3,3,3,3,
3,3,3,3,3,3,3,3,3,3,3,3,3,3,3,4),(34.5575191894877,34.5837986101777,34.6716443439734,
34.7593798166834,34.8470279893519,34.937636603843,35.0251871530733,35.1127250164892,
35.2002708147692,35.287845169183,35.3755160519479,35.4632446154677,35.5510974900254,
35.5718969052803,35.6597426387321,35.7474781110943,35.8351262834116,35.925734898033,
36.0132854469052,36.1008233099611,36.1883691078795,36.2759434619307,36.3636143443333,
36.4513429074904,36.5391957816878,36.559995200383,36.6478465408607,36.7355748488331,
36.7834594513572),.UNSPECIFIED.);
#1494=B_SPLINE_CURVE_WITH_KNOTS('',3,(#28381,#28382,#28383,#28384,#28385,
#28386,#28387,#28388,#28389,#28390,#28391,#28392,#28393,#28394,#28395,#28396,
#28397,#28398,#28399,#28400,#28401,#28402,#28403,#28404,#28405,#28406,#28407,
#28408,#28409,#28410,#28411,#28412,#28413,#28414,#28415,#28416,#28417,#28418,
#28419,#28420,#28421,#28422,#28423,#28424,#28425,#28426,#28427,#28428,#28429,
#28430,#28431,#28432,#28433,#28434,#28435,#28436,#28437,#28438,#28439,#28440,
#28441,#28442,#28443,#28444,#28445,#28446,#28447,#28448,#28449,#28450,#28451,
#28452,#28453,#28454,#28455,#28456,#28457,#28458,#28459,#28460,#28461,#28462),
 .UNSPECIFIED.,.F.,.F.,(4,3,3,3,3,3,3,3,3,3,3,3,3,3,3,3,3,3,3,3,3,3,3,3,
3,3,3,4),(34.5575191894877,34.6462452281606,34.7349963989685,34.8237912713786,
34.9127093964719,35.001694277295,35.0908349295251,35.1491898438735,35.2370355770745,
35.3247710491863,35.4124192212535,35.5030278359688,35.5905783845939,35.6781162474045,
35.7656620450795,35.8532363988891,35.9409072810548,36.0286358439772,36.1164887179452,
36.1372881389761,36.2251186640309,36.3128459868409,36.4004909011797,36.4880741337705,
36.5756228794804,36.6631518391531,36.7506985294834,36.782489025435),
 .UNSPECIFIED.);
#1495=B_SPLINE_CURVE_WITH_KNOTS('',3,(#28463,#28464,#28465,#28466,#28467,
#28468,#28469,#28470,#28471,#28472,#28473,#28474,#28475,#28476,#28477,#28478,
#28479,#28480,#28481,#28482,#28483,#28484,#28485,#28486,#28487,#28488,#28489,
#28490,#28491,#28492,#28493,#28494,#28495,#28496,#28497,#28498,#28499,#28500,
#28501,#28502,#28503,#28504,#28505,#28506,#28507,#28508,#28509,#28510,#28511,
#28512,#28513,#28514,#28515,#28516,#28517,#28518,#28519,#28520,#28521,#28522,
#28523,#28524,#28525,#28526,#28527,#28528,#28529,#28530,#28531,#28532,#28533,
#28534,#28535,#28536,#28537,#28538,#28539,#28540,#28541,#28542,#28543,#28544,
#28545,#28546,#28547,#28548,#28549,#28550,#28551,#28552,#28553,#28554,#28555,
#28556,#28557,#28558,#28559,#28560,#28561,#28562,#28563,#28564,#28565,#28566,
#28567,#28568,#28569,#28570,#28571,#28572,#28573,#28574,#28575,#28576,#28577,
#28578,#28579,#28580,#28581,#28582,#28583,#28584,#28585,#28586,#28587,#28588,
#28589,#28590,#28591,#28592,#28593,#28594,#28595,#28596,#28597,#28598,#28599,
#28600,#28601,#28602,#28603,#28604,#28605,#28606,#28607),.UNSPECIFIED.,
 .F.,.F.,(4,3,3,3,3,3,3,3,3,3,3,3,3,3,3,3,3,3,3,3,3,3,3,3,3,3,3,3,3,3,3,
3,3,3,3,3,3,3,3,3,3,3,3,3,3,3,3,3,4),(30.5002119601245,30.5877840746677,
30.6753288207514,30.7628668275658,30.8504187144882,30.9380598353038,31.0257454406997,
31.1135727002447,31.1967966634628,31.2846424112103,31.3723778980337,31.4600260849591,
31.5506346941599,31.6381852579116,31.7257231359216,31.8132689488522,31.9008433179572,
31.9885142154005,32.0762427936085,32.1640956827569,32.1848949585655,32.2727406910854,
32.3604761625352,32.4481243339609,32.5387329489243,32.6262834969632,32.7138213592091,
32.8013671563419,32.888941509632,32.9766123913153,33.0643409537762,33.1521938273171,
33.1729932536681,33.2608389840538,33.3485744532963,33.4362226224444,33.5268312382352,
33.614381783836,33.7019196435887,33.7894654381741,33.8770397888678,33.9647106678921,
34.0524392276545,34.1402920984597,34.1610915487708,34.2601984589017,34.3572237828832,
34.4573714860888,34.5575191892943),.UNSPECIFIED.);
#1496=B_SPLINE_CURVE_WITH_KNOTS('',3,(#28613,#28614,#28615,#28616,#28617,
#28618,#28619,#28620,#28621,#28622,#28623,#28624,#28625,#28626,#28627,#28628,
#28629,#28630,#28631,#28632,#28633,#28634,#28635,#28636,#28637,#28638,#28639,
#28640,#28641,#28642,#28643,#28644,#28645,#28646,#28647,#28648,#28649,#28650,
#28651,#28652,#28653,#28654,#28655,#28656,#28657,#28658,#28659,#28660,#28661,
#28662,#28663,#28664,#28665,#28666,#28667,#28668,#28669,#28670,#28671,#28672,
#28673,#28674,#28675,#28676,#28677,#28678,#28679,#28680,#28681,#28682,#28683,
#28684,#28685,#28686,#28687,#28688,#28689,#28690,#28691,#28692,#28693,#28694,
#28695,#28696,#28697,#28698,#28699,#28700,#28701,#28702,#28703,#28704,#28705,
#28706,#28707,#28708,#28709,#28710,#28711,#28712,#28713,#28714,#28715,#28716,
#28717,#28718,#28719,#28720,#28721,#28722,#28723,#28724,#28725,#28726,#28727,
#28728,#28729,#28730,#28731,#28732,#28733,#28734,#28735,#28736,#28737,#28738,
#28739,#28740,#28741,#28742,#28743,#28744,#28745,#28746,#28747,#28748,#28749,
#28750,#28751,#28752,#28753,#28754,#28755,#28756,#28757,#28758,#28759,#28760),
 .UNSPECIFIED.,.F.,.F.,(4,3,3,3,3,3,3,3,3,3,3,3,3,3,3,3,3,3,3,3,3,3,3,3,
3,3,3,3,3,3,3,3,3,3,3,3,3,3,3,3,3,3,3,3,3,3,3,3,3,4),(24.2165026702176,
24.304043926345,24.3916073461436,24.479264250075,24.5669730854259,24.6548135226413,
24.702815659151,24.7906611702751,24.8783964169397,24.9660443604867,25.0566530597075,
25.1442033736151,25.2317409998204,25.3192865592566,25.406860673447,25.4945313151421,
25.5822596368198,25.6701122702235,25.6909139542537,25.7787597849543,25.8664953555964,
25.9541436270979,26.0447522048802,26.1323028545467,26.2198408188163,26.3073867182571,
26.3949611740288,26.4826321579353,26.5703608225863,26.6582137974992,26.6790122493564,
26.7668579861124,26.854593462076,26.9422416382858,27.0328502515574,27.1204008050279,
27.2079386729366,27.2954844759584,27.3830588353586,27.470729723451,27.5584582925036,
27.6463111728529,27.667110544459,27.7558874872272,27.844547755712,27.9331107998525,
28.02158503414,28.1100063153203,28.198402509401,28.2743338823081),
 .UNSPECIFIED.);
#1497=B_SPLINE_CURVE_WITH_KNOTS('',3,(#28761,#28762,#28763,#28764,#28765,
#28766,#28767,#28768,#28769,#28770,#28771,#28772,#28773,#28774,#28775,#28776,
#28777,#28778,#28779,#28780,#28781,#28782,#28783,#28784,#28785,#28786,#28787,
#28788,#28789,#28790,#28791,#28792,#28793,#28794,#28795,#28796,#28797,#28798,
#28799,#28800,#28801,#28802,#28803,#28804,#28805,#28806,#28807,#28808,#28809,
#28810,#28811,#28812,#28813,#28814,#28815,#28816,#28817,#28818,#28819,#28820,
#28821,#28822,#28823,#28824,#28825,#28826,#28827,#28828,#28829,#28830,#28831,
#28832,#28833,#28834,#28835,#28836,#28837,#28838,#28839),.UNSPECIFIED.,
 .F.,.F.,(4,3,3,3,3,3,3,3,3,3,3,3,3,3,3,3,3,3,3,3,3,3,3,3,3,3,4),(28.274333882515,
28.3719019718884,28.4698037533802,28.5681844676917,28.6552088395617,28.7430545874032,
28.8307900743218,28.9184382613433,29.0090468705085,29.0965974343581,29.1841353124666,
29.271681125496,29.3592554947003,29.4469263922428,29.5346549705495,29.6225078597965,
29.6433071346644,29.731160848353,29.8189024061471,29.9065417520996,29.9941237136733,
30.0816689585669,30.169198122729,30.2567665282248,30.34435384216,30.4320320091579,
30.4992123502324),.UNSPECIFIED.);
#1498=B_SPLINE_CURVE_WITH_KNOTS('',3,(#28841,#28842,#28843,#28844,#28845,
#28846,#28847,#28848,#28849,#28850,#28851,#28852,#28853,#28854,#28855,#28856,
#28857,#28858,#28859,#28860,#28861,#28862,#28863,#28864,#28865,#28866,#28867,
#28868,#28869,#28870,#28871,#28872,#28873,#28874,#28875,#28876,#28877,#28878,
#28879,#28880,#28881,#28882,#28883,#28884,#28885,#28886,#28887,#28888,#28889,
#28890,#28891,#28892,#28893,#28894,#28895,#28896,#28897,#28898,#28899,#28900,
#28901,#28902,#28903,#28904,#28905,#28906,#28907,#28908,#28909,#28910,#28911,
#28912,#28913,#28914,#28915,#28916,#28917,#28918,#28919,#28920,#28921,#28922),
 .UNSPECIFIED.,.F.,.F.,(4,3,3,3,3,3,3,3,3,3,3,3,3,3,3,3,3,3,3,3,3,3,3,3,
3,3,3,4),(28.2743338824402,28.3615964636159,28.4487512272485,28.5358217800874,
28.6228345545296,28.709817282874,28.796791179032,28.883777445679,28.970850571241,
29.0579679319872,29.1452235371721,29.2206000732575,29.3084458100498,29.3961812860485,
29.4838294622926,29.5744380755511,29.6619886290536,29.7495264969936,29.8370723000451,
29.9246466594751,30.0123175475949,30.1000461166736,30.1878989970478,30.2086983683601,
30.2965346095156,30.3842739178244,30.471919062604,30.5002119601245),
 .UNSPECIFIED.);
#1499=B_SPLINE_CURVE_WITH_KNOTS('',3,(#28923,#28924,#28925,#28926,#28927,
#28928,#28929,#28930,#28931,#28932,#28933,#28934,#28935,#28936,#28937,#28938,
#28939,#28940,#28941,#28942,#28943,#28944,#28945,#28946,#28947,#28948,#28949,
#28950,#28951,#28952,#28953,#28954,#28955,#28956,#28957,#28958,#28959,#28960,
#28961,#28962,#28963,#28964,#28965,#28966,#28967,#28968,#28969,#28970,#28971,
#28972,#28973,#28974,#28975,#28976,#28977,#28978,#28979,#28980,#28981,#28982,
#28983,#28984,#28985,#28986,#28987,#28988,#28989,#28990,#28991,#28992,#28993,
#28994,#28995,#28996,#28997,#28998,#28999,#29000,#29001,#29002,#29003,#29004,
#29005,#29006,#29007,#29008,#29009,#29010,#29011,#29012,#29013,#29014,#29015,
#29016,#29017,#29018,#29019,#29020,#29021,#29022,#29023,#29024,#29025,#29026,
#29027,#29028,#29029,#29030,#29031,#29032,#29033,#29034,#29035,#29036,#29037,
#29038,#29039,#29040,#29041,#29042,#29043,#29044,#29045,#29046,#29047,#29048,
#29049,#29050,#29051,#29052,#29053,#29054,#29055,#29056,#29057,#29058,#29059,
#29060,#29061,#29062,#29063,#29064,#29065,#29066,#29067,#29068,#29069,#29070,
#29071,#29072,#29073),.UNSPECIFIED.,.F.,.F.,(4,3,3,3,3,3,3,3,3,3,3,3,3,
3,3,3,3,3,3,3,3,3,3,3,3,3,3,3,3,3,3,3,3,3,3,3,3,3,3,3,3,3,3,3,3,3,3,3,3,
3,4),(24.2162169687424,24.2801085977442,24.3679525734171,24.4556862627458,
24.5433326291174,24.6339419120835,24.7214906094836,24.809026607426,24.8965705285987,
24.9841429962742,25.0718119874431,25.1595386543509,25.2473896392159,25.2682068928468,
25.3560532509127,25.443789353695,25.531438161423,25.6220465397388,25.7095977323268,
25.7971362410408,25.8846826858492,25.9722576873129,26.0599292146498,26.1476584220326,
26.2355119345706,26.2563051879495,26.3441510274158,26.4318866090919,26.5195348938718,
26.6101434675193,26.6976941360126,26.7852321211407,26.8727780434585,26.9603525241144,
27.0480235357698,27.1357522298776,27.2236052365278,27.2444034830521,27.332248995167,
27.4199842428374,27.507632187404,27.5982408862479,27.6857912012032,27.7733288284647,
27.8608743889645,27.9484485042248,28.0361191469941,28.1238474697496,28.2117001042282,
28.2325017781548,28.2743338823081),.UNSPECIFIED.);
#1500=B_SPLINE_CURVE_WITH_KNOTS('',3,(#29079,#29080,#29081,#29082,#29083,
#29084,#29085,#29086,#29087,#29088,#29089,#29090,#29091,#29092,#29093,#29094,
#29095,#29096,#29097,#29098,#29099,#29100,#29101,#29102,#29103,#29104,#29105,
#29106,#29107,#29108,#29109,#29110,#29111,#29112,#29113,#29114,#29115,#29116,
#29117,#29118,#29119,#29120,#29121,#29122,#29123,#29124,#29125,#29126,#29127,
#29128,#29129,#29130,#29131,#29132,#29133,#29134,#29135,#29136,#29137,#29138,
#29139,#29140,#29141,#29142,#29143,#29144,#29145,#29146,#29147,#29148,#29149,
#29150,#29151,#29152,#29153,#29154,#29155,#29156,#29157,#29158,#29159,#29160),
 .UNSPECIFIED.,.F.,.F.,(4,3,3,3,3,3,3,3,3,3,3,3,3,3,3,3,3,3,3,3,3,3,3,3,
3,3,3,4),(15.7079632679489,15.7947000247825,15.8814152765578,15.9681303731201,
16.0548666599654,16.1417000066177,16.2285855560594,16.3156125279741,16.3753222369229,
16.4632671529562,16.551101682674,16.6388486586907,16.7294201428575,16.8170681804461,
16.904702862179,16.9923446932266,17.0800141787253,17.1677783645445,17.2555992653293,
17.3435423677208,17.3634205320255,17.4513971777302,17.5392714562485,17.6270639960291,
17.7147927338977,17.8024841872462,17.8901701658632,17.9330836177785),
 .UNSPECIFIED.);
#1501=B_SPLINE_CURVE_WITH_KNOTS('',3,(#29162,#29163,#29164,#29165,#29166),
 .UNSPECIFIED.,.F.,.F.,(4,1,4),(14.3991256467175,15.3872239418202,15.7079550816507),
 .UNSPECIFIED.);
#1502=B_SPLINE_CURVE_WITH_KNOTS('',3,(#29170,#29171,#29172,#29173,#29174,
#29175,#29176,#29177,#29178,#29179,#29180,#29181,#29182,#29183,#29184,#29185,
#29186,#29187,#29188,#29189,#29190,#29191,#29192,#29193,#29194,#29195,#29196,
#29197,#29198,#29199,#29200,#29201,#29202,#29203,#29204,#29205,#29206,#29207,
#29208,#29209,#29210,#29211,#29212,#29213,#29214,#29215,#29216,#29217,#29218,
#29219,#29220,#29221,#29222,#29223,#29224,#29225,#29226,#29227,#29228,#29229,
#29230,#29231,#29232,#29233,#29234,#29235,#29236),.UNSPECIFIED.,.F.,.F.,
(4,3,3,3,3,3,3,3,3,3,3,3,3,3,3,3,3,3,3,3,3,3,4),(13.8752089252097,13.9625451768154,
14.0497728503132,14.1369154800046,14.2239988322353,14.3110512064015,14.3980937504697,
14.4851476003848,14.5722863531229,14.6594683187599,14.7467864178897,14.8218327081244,
14.9086977820188,14.9954555529545,15.0845190173028,15.1711346234622,15.2577220080351,
15.3443027284837,15.435217863298,15.5218933969664,15.6086174094582,15.6954502207414,
15.7079632677406),.UNSPECIFIED.);
#1503=B_SPLINE_CURVE_WITH_KNOTS('',3,(#29237,#29238,#29239,#29240,#29241,
#29242,#29243,#29244,#29245,#29246,#29247,#29248,#29249,#29250,#29251,#29252,
#29253,#29254,#29255,#29256,#29257,#29258,#29259,#29260,#29261,#29262,#29263,
#29264,#29265,#29266,#29267,#29268,#29269,#29270,#29271,#29272,#29273,#29274,
#29275,#29276,#29277,#29278,#29279,#29280,#29281,#29282,#29283,#29284,#29285,
#29286,#29287,#29288,#29289,#29290,#29291,#29292,#29293,#29294,#29295,#29296,
#29297,#29298,#29299,#29300,#29301,#29302,#29303,#29304,#29305,#29306,#29307,
#29308,#29309,#29310,#29311,#29312,#29313,#29314,#29315,#29316,#29317,#29318),
 .UNSPECIFIED.,.F.,.F.,(4,3,3,3,3,3,3,3,3,3,3,3,3,3,3,3,3,3,3,3,3,3,3,3,
3,3,3,4),(15.7079632679489,15.8099310032271,15.8976761278721,15.985309708943,
16.0728548384208,16.1635016459094,16.2509469329345,16.3383788932871,16.4258182602526,
16.5132857674034,16.6008497171709,16.6884711726235,16.7762174884443,16.7980292983297,
16.8858955432857,16.9736516099389,17.0613204330381,17.1519213280874,17.2394925318178,
17.3270510142323,17.4146173727509,17.5022122053289,17.589903340914,17.6776520485815,
17.7655247566336,17.7861275934324,17.873977809986,17.9338553089788),
 .UNSPECIFIED.);
#1504=B_SPLINE_CURVE_WITH_KNOTS('',3,(#29324,#29325,#29326,#29327,#29328,
#29329,#29330,#29331,#29332,#29333,#29334,#29335,#29336,#29337,#29338,#29339,
#29340,#29341,#29342,#29343,#29344,#29345,#29346,#29347,#29348,#29349,#29350,
#29351,#29352,#29353,#29354,#29355,#29356,#29357,#29358,#29359,#29360,#29361,
#29362,#29363),.UNSPECIFIED.,.F.,.F.,(4,3,3,3,3,3,3,3,3,3,3,3,3,4),(-55.2918140047847,
-55.200308089966,-55.1089206909327,-55.013481383397,-54.9222481364232,-54.8310438513113,
-54.7398442083826,-54.6486248978994,-54.5573105633689,-54.4659402820255,
-54.3744361879659,-54.3454062306465,-54.2237243441527,-54.1159079025692),
 .UNSPECIFIED.);
#1505=B_SPLINE_CURVE_WITH_KNOTS('',3,(#29365,#29366,#29367,#29368,#29369,
#29370,#29371,#29372,#29373,#29374),.UNSPECIFIED.,.F.,.F.,(4,1,1,1,1,1,
1,4),(-54.1159079025692,-53.3573079355439,-52.3692096404412,-51.3811113453385,
-50.3930130502359,-49.4049147551332,-48.4168164600305,-47.8327225953897),
 .UNSPECIFIED.);
#1506=B_SPLINE_CURVE_WITH_KNOTS('',3,(#29376,#29377,#29378,#29379,#29380,
#29381,#29382,#29383,#29384,#29385,#29386,#29387,#29388,#29389,#29390,#29391,
#29392,#29393,#29394,#29395,#29396,#29397,#29398,#29399,#29400,#29401,#29402,
#29403,#29404,#29405,#29406,#29407,#29408,#29409,#29410,#29411,#29412,#29413,
#29414,#29415,#29416,#29417,#29418,#29419,#29420,#29421,#29422,#29423,#29424,
#29425,#29426,#29427,#29428,#29429,#29430,#29431,#29432,#29433,#29434,#29435,
#29436,#29437,#29438,#29439,#29440,#29441,#29442,#29443,#29444,#29445,#29446,
#29447,#29448,#29449,#29450,#29451,#29452,#29453,#29454,#29455,#29456,#29457,
#29458,#29459,#29460,#29461,#29462,#29463,#29464,#29465,#29466,#29467,#29468,
#29469,#29470,#29471,#29472,#29473,#29474,#29475,#29476,#29477,#29478,#29479,
#29480,#29481,#29482,#29483,#29484,#29485,#29486,#29487,#29488,#29489,#29490,
#29491,#29492,#29493,#29494,#29495,#29496,#29497,#29498,#29499,#29500,#29501,
#29502,#29503,#29504,#29505,#29506,#29507,#29508,#29509,#29510,#29511,#29512,
#29513,#29514,#29515,#29516,#29517,#29518,#29519,#29520,#29521,#29522,#29523,
#29524,#29525,#29526,#29527,#29528,#29529,#29530,#29531,#29532,#29533,#29534,
#29535,#29536,#29537,#29538,#29539,#29540,#29541,#29542,#29543,#29544,#29545,
#29546,#29547,#29548,#29549,#29550,#29551,#29552,#29553,#29554,#29555,#29556,
#29557,#29558,#29559,#29560,#29561,#29562,#29563,#29564,#29565,#29566,#29567,
#29568,#29569,#29570,#29571,#29572,#29573,#29574,#29575,#29576,#29577,#29578,
#29579,#29580,#29581,#29582,#29583,#29584,#29585,#29586,#29587,#29588,#29589,
#29590,#29591,#29592,#29593,#29594,#29595,#29596,#29597,#29598,#29599,#29600,
#29601,#29602,#29603,#29604,#29605,#29606,#29607,#29608,#29609,#29610,#29611,
#29612,#29613,#29614,#29615,#29616,#29617,#29618,#29619,#29620,#29621,#29622,
#29623,#29624,#29625,#29626,#29627,#29628,#29629,#29630,#29631,#29632,#29633,
#29634,#29635,#29636,#29637,#29638,#29639,#29640,#29641,#29642,#29643,#29644,
#29645,#29646,#29647,#29648,#29649,#29650,#29651,#29652,#29653,#29654,#29655,
#29656,#29657,#29658,#29659,#29660,#29661,#29662,#29663,#29664,#29665,#29666,
#29667,#29668,#29669,#29670,#29671,#29672,#29673,#29674,#29675,#29676,#29677,
#29678,#29679,#29680,#29681,#29682,#29683,#29684,#29685,#29686,#29687,#29688,
#29689,#29690,#29691,#29692,#29693,#29694,#29695,#29696,#29697,#29698,#29699,
#29700,#29701,#29702,#29703,#29704,#29705,#29706,#29707,#29708,#29709,#29710,
#29711,#29712,#29713,#29714,#29715,#29716,#29717,#29718,#29719),
 .UNSPECIFIED.,.F.,.F.,(4,2,2,2,2,2,2,2,2,2,2,2,2,2,2,2,2,2,2,2,2,2,2,2,
2,2,2,2,2,2,2,2,2,2,2,2,2,2,2,2,2,2,2,2,2,2,2,2,2,2,2,2,2,2,2,2,2,2,2,2,
2,2,2,2,2,2,2,2,2,2,2,2,2,2,2,2,2,2,2,2,2,2,2,2,2,2,2,2,2,2,2,2,2,2,2,2,
2,2,2,2,2,2,2,2,2,2,2,2,2,2,2,2,2,2,2,2,2,2,2,2,2,2,2,2,2,2,2,2,2,2,2,2,
2,2,2,2,2,2,2,2,2,2,2,2,2,2,2,2,2,2,2,2,2,2,2,2,2,2,2,2,2,2,2,2,2,2,2,2,
2,2,2,4),(-4.26994477188097,-4.18620642098893,-4.14748543155145,-4.13836516395927,
-4.13271644558837,-4.1270209789431,-4.11767887414803,-4.07387176272375,
-4.01754675939132,-3.98526852873032,-3.97244252517069,-3.962928101753,-3.95263455188417,
-3.93561297279341,-3.86906486919751,-3.83032039001781,-3.80888467938486,
-3.80115287219542,-3.79576180824508,-3.78960303190388,-3.77835581422881,
-3.7362332495788,-3.68241613757305,-3.64973455052119,-3.63685676513584,
-3.62733391275226,-3.61705919469465,-3.60013604758476,-3.53178867699976,
-3.49419379877283,-3.4731285686711,-3.46544214860115,-3.46005724725163,
-3.45387538386639,-3.44251852409717,-3.39772741841958,-3.35693498688948,
-3.3294400047532,-3.30871723415067,-3.29770329336156,-3.28926037190288,
-3.27811268307046,-3.25732552411916,-3.18265367848997,-3.14387805607392,
-3.13291347210378,-3.12687793802281,-3.1215052928004,-3.11482851828834,
-3.09758541865381,-3.01707586610079,-2.97968868891503,-2.96627243337736,
-2.95666593248693,-2.9465806454064,-2.93060660716385,-2.84360477723358,
-2.80473702597104,-2.79560979365303,-2.7899593655879,-2.78426455654238,
-2.77492746042689,-2.73211187317539,-2.67505866187918,-2.64257356381414,
-2.62972052078187,-2.62020133905442,-2.60991692082377,-2.59294487551698,
-2.52538738746047,-2.48729318260763,-2.46606554778313,-2.45835895299769,
-2.4529712260203,-2.4467995486916,-2.43549124031871,-2.39171201103291,-2.35042959737762,
-2.30917187563767,-2.29538278530595,-2.2857123488288,-2.27573191572309,
-2.26029141076709,-2.17923413867982,-2.14829963663161,-2.13533478824122,
-2.12516345695904,-2.11929233086499,-2.11377547208397,-2.10531130332818,
-2.07676876291054,-2.00666750220054,-1.97247547910195,-1.95909672289662,
-1.94959075765524,-1.93951659775975,-1.92360179357811,-1.8514479429695,
-1.80226477432625,-1.79069313230599,-1.78446566593839,-1.77909249592087,
-1.7714923613653,-1.7511068894382,-1.71554791286426,-1.64362474358197,-1.62699472507492,
-1.61677806746921,-1.60723191970796,-1.594200400812,-1.56026258045255,-1.49766369007068,
-1.461899074237,-1.45279208968934,-1.44714568458261,-1.4414459482241,-1.43208640880257,
-1.38696841275484,-1.3053997793046,-1.29002649639216,-1.2800590989145,-1.2703795523322,
-1.25653905821626,-1.2146844741299,-1.17235755187968,-1.1302969132056,-1.11905357834372,
-1.11289563802632,-1.10750398798881,-1.09976958887906,-1.07831825775197,
-1.03952673566653,-0.972988352111049,-0.955961612124122,-0.945666289777868,
-0.936151098026857,-0.923325275213903,-0.891051311495818,-0.834734568395268,
-0.790981030348268,-0.781640398928958,-0.775944849883415,-0.77029522471581,
-0.761171506665113,-0.722397011506791,-0.63515619010766,-0.619222062684149,
-0.609144749818193,-0.599534133867639,-0.586092366400709,-0.548451508328222,
-0.466073284500351,-0.449999401583243,-0.443099403504667,-0.437782511925628,
-0.43116817181859,-0.417199430816387,-0.39719431811366,-0.321105245779795,
-0.292257616498562,-0.28080797748469,-0.271268815467881,-0.261256811036364,
-0.245652941595711,-0.183326665219496,-0.122229251623277,-0.111399598244366,
-0.105391929826403,-0.0999461477571767,-0.0918711243274098,-0.067426883443743,
-0.000960198174506648),.UNSPECIFIED.);
#1507=B_SPLINE_CURVE_WITH_KNOTS('',3,(#29721,#29722,#29723,#29724,#29725,
#29726,#29727,#29728,#29729,#29730,#29731,#29732,#29733,#29734,#29735,#29736,
#29737,#29738,#29739,#29740,#29741,#29742,#29743,#29744,#29745,#29746,#29747,
#29748,#29749,#29750,#29751,#29752,#29753,#29754,#29755,#29756,#29757,#29758,
#29759,#29760,#29761,#29762,#29763,#29764,#29765,#29766,#29767,#29768,#29769,
#29770,#29771,#29772,#29773,#29774,#29775,#29776,#29777,#29778,#29779,#29780,
#29781,#29782,#29783,#29784,#29785,#29786,#29787,#29788,#29789,#29790,#29791,
#29792,#29793,#29794,#29795,#29796,#29797,#29798,#29799,#29800,#29801,#29802,
#29803,#29804,#29805,#29806,#29807,#29808,#29809,#29810,#29811,#29812,#29813,
#29814,#29815,#29816,#29817,#29818,#29819,#29820,#29821,#29822,#29823,#29824,
#29825,#29826,#29827,#29828,#29829,#29830,#29831,#29832,#29833,#29834,#29835,
#29836,#29837,#29838,#29839,#29840,#29841,#29842,#29843,#29844,#29845,#29846,
#29847,#29848,#29849,#29850,#29851,#29852,#29853,#29854,#29855,#29856,#29857,
#29858,#29859,#29860,#29861,#29862,#29863,#29864,#29865,#29866,#29867,#29868,
#29869,#29870,#29871,#29872,#29873,#29874,#29875,#29876,#29877,#29878,#29879,
#29880,#29881,#29882,#29883,#29884,#29885,#29886,#29887,#29888,#29889,#29890,
#29891,#29892,#29893,#29894,#29895,#29896,#29897,#29898,#29899,#29900,#29901,
#29902,#29903,#29904,#29905,#29906,#29907,#29908,#29909,#29910,#29911,#29912,
#29913,#29914,#29915,#29916,#29917,#29918,#29919,#29920,#29921,#29922,#29923,
#29924,#29925,#29926,#29927,#29928,#29929,#29930,#29931,#29932,#29933,#29934,
#29935,#29936,#29937,#29938,#29939,#29940,#29941,#29942,#29943,#29944,#29945,
#29946,#29947,#29948,#29949,#29950,#29951,#29952,#29953,#29954,#29955,#29956,
#29957,#29958,#29959,#29960,#29961,#29962,#29963,#29964,#29965,#29966,#29967,
#29968,#29969,#29970,#29971,#29972,#29973,#29974,#29975,#29976,#29977,#29978,
#29979,#29980,#29981,#29982,#29983,#29984,#29985,#29986,#29987,#29988,#29989,
#29990,#29991,#29992,#29993,#29994,#29995,#29996,#29997,#29998,#29999,#30000,
#30001,#30002,#30003,#30004,#30005,#30006,#30007,#30008,#30009,#30010,#30011,
#30012,#30013,#30014,#30015,#30016,#30017,#30018,#30019,#30020,#30021,#30022,
#30023,#30024,#30025,#30026,#30027,#30028,#30029,#30030,#30031,#30032,#30033,
#30034,#30035,#30036,#30037,#30038,#30039,#30040,#30041,#30042,#30043,#30044,
#30045,#30046,#30047,#30048,#30049,#30050,#30051,#30052,#30053,#30054,#30055,
#30056,#30057,#30058,#30059,#30060,#30061,#30062,#30063,#30064,#30065,#30066,
#30067,#30068,#30069,#30070,#30071,#30072),.UNSPECIFIED.,.F.,.F.,(4,2,2,
2,2,2,2,2,2,2,2,2,2,2,2,2,2,2,2,2,2,2,2,2,2,2,2,2,2,2,2,2,2,2,2,2,2,2,2,
2,2,2,2,2,2,2,2,2,2,2,2,2,2,2,2,2,2,2,2,2,2,2,2,2,2,2,2,2,2,2,2,2,2,2,2,
2,2,2,2,2,2,2,2,2,2,2,2,2,2,2,2,2,2,2,2,2,2,2,2,2,2,2,2,2,2,2,2,2,2,2,2,
2,2,2,2,2,2,2,2,2,2,2,2,2,2,2,2,2,2,2,2,2,2,2,2,2,2,2,2,2,2,2,2,2,2,2,2,
2,2,2,2,2,2,2,2,2,2,2,2,2,2,2,2,2,2,2,2,2,2,2,2,2,2,2,2,4),(-4.27059191801562,
-4.24196876919374,-4.22385973473245,-4.21436402168296,-4.2047751676493,
-4.1946519009215,-4.17849128458808,-4.10207530338911,-4.05747736067456,
-4.04585741665701,-4.03968862220837,-4.03429922385486,-4.02658418269025,
-4.00679767812497,-3.9310481657219,-3.89246027380088,-3.87892045828133,
-3.86929214802734,-3.86044047903144,-3.8457657369372,-3.79189565768603,
-3.74022540558451,-3.7152300526998,-3.70709742187507,-3.70164114629446,
-3.69565476708377,-3.68493039532081,-3.61049175689382,-3.57596808241161,
-3.55175292576472,-3.5401162660358,-3.53072659874922,-3.51975526209588,
-3.49985900339185,-3.42410203867415,-3.38181942257708,-3.37255216081011,
-3.36687202864412,-3.36120720764951,-3.35201198631407,-3.31420107234795,
-3.25323492456459,-3.21970159510757,-3.2067186663568,-3.19718017740198,
-3.18694605318795,-3.17022679534539,-3.09929802141095,-3.04794558651569,
-3.03769477720689,-3.03180690703177,-3.02636517558088,-3.01801162993682,
-2.99289972927415,-2.92837390344399,-2.88610869428038,-2.87223170651612,
-2.86254525807201,-2.85258627550684,-2.83725810609607,-2.75543053189016,
-2.71051949034609,-2.70116659430284,-2.69546802786206,-2.69049786443901,
-2.68204508448587,-2.65583878926124,-2.59236284249322,-2.55030675706438,
-2.53644714973095,-2.52676350204291,-2.51797328147161,-2.50366247518195,
-2.46132376792588,-2.39983496424085,-2.37276281360786,-2.36442868823619,
-2.35893608386402,-2.35302212044934,-2.34264660271004,-2.27692567609068,
-2.21880559498243,-2.20296746036063,-2.19290845743233,-2.18339444586113,
-2.16996592539066,-2.13525690721975,-2.06667648989202,-2.03778568923793,
-2.02909722412373,-2.02408557196433,-2.01844794309958,-2.00938220832573,
-1.97181297484136,-1.88660392951311,-1.86890798361453,-1.85847973501213,
-1.8490062034207,-1.83648414335042,-1.80649587787756,-1.75750249923547,
-1.70720830751179,-1.69585139718436,-1.68966948180517,-1.68428492311556,
-1.67659913041973,-1.65553851933186,-1.6179587234071,-1.54951016229661,
-1.53258769638991,-1.52231333433264,-1.51279091052716,-1.49991386167171,
-1.46723239588009,-1.41340729504675,-1.37135559917556,-1.36011268812664,
-1.35395488018644,-1.34856327250305,-1.34082883144026,-1.31937668193981,
-1.28058225159961,-1.21404980802564,-1.19702304675881,-1.18672779987367,
-1.17721273327544,-1.16438716502752,-1.13211441026811,-1.07580124171744,
-1.03204421945698,-1.02270368075276,-1.01700819448616,-1.01135863898363,
-1.00223504342647,-0.963461333270413,-0.876220907429709,-0.860287097017765,
-0.850209928659237,-0.840599412291213,-0.8271577199114,-0.789516498328059,
-0.707133350560775,-0.691064464453122,-0.684165315413099,-0.678848525449104,
-0.672233600903381,-0.658261341206739,-0.638249000282644,-0.562076359109543,
-0.533305600417685,-0.521863388103103,-0.51232601324372,-0.502311323061108,
-0.48669338720172,-0.426505026314306,-0.362914715334719,-0.352305199504254,
-0.346343060858523,-0.340876490943651,-0.332682258085611,-0.307070922609296,
-0.252718367043309,-0.202067395795723,-0.187470412963257,-0.178632854184781,
-0.168995201225525,-0.155394106272744,-0.116158525585101,-0.0675072931087099,
-0.0670493361224295,-0.0450770216706815,-0.022366969529527,-0.0144508372849338,
-0.00907719224608754,-0.0047451534040328,-0.000959030470956043),
 .UNSPECIFIED.);
#1508=B_SPLINE_CURVE_WITH_KNOTS('',3,(#30074,#30075,#30076,#30077,#30078,
#30079,#30080,#30081,#30082,#30083,#30084,#30085,#30086,#30087,#30088,#30089,
#30090,#30091,#30092,#30093,#30094,#30095,#30096,#30097,#30098,#30099,#30100,
#30101,#30102,#30103,#30104,#30105,#30106,#30107,#30108,#30109,#30110,#30111,
#30112,#30113,#30114,#30115,#30116,#30117,#30118,#30119,#30120,#30121,#30122,
#30123,#30124,#30125,#30126,#30127,#30128,#30129,#30130,#30131,#30132,#30133,
#30134,#30135,#30136,#30137,#30138,#30139,#30140,#30141,#30142,#30143,#30144,
#30145,#30146,#30147,#30148,#30149,#30150,#30151,#30152,#30153,#30154,#30155,
#30156,#30157,#30158,#30159,#30160,#30161,#30162,#30163,#30164,#30165,#30166,
#30167,#30168,#30169,#30170,#30171,#30172,#30173,#30174,#30175,#30176,#30177,
#30178,#30179,#30180,#30181,#30182,#30183,#30184,#30185,#30186,#30187,#30188,
#30189,#30190,#30191,#30192,#30193,#30194,#30195,#30196,#30197,#30198,#30199,
#30200,#30201,#30202,#30203,#30204,#30205,#30206,#30207,#30208,#30209,#30210,
#30211,#30212,#30213,#30214,#30215,#30216,#30217,#30218,#30219,#30220,#30221,
#30222,#30223,#30224,#30225,#30226,#30227,#30228,#30229,#30230,#30231,#30232,
#30233,#30234,#30235,#30236,#30237,#30238,#30239,#30240,#30241,#30242,#30243,
#30244,#30245,#30246,#30247,#30248,#30249,#30250,#30251,#30252,#30253,#30254,
#30255,#30256,#30257,#30258,#30259,#30260,#30261,#30262,#30263,#30264,#30265,
#30266,#30267,#30268,#30269,#30270,#30271,#30272,#30273,#30274,#30275,#30276,
#30277,#30278,#30279,#30280,#30281,#30282,#30283,#30284,#30285,#30286,#30287,
#30288,#30289,#30290,#30291,#30292,#30293,#30294,#30295,#30296,#30297,#30298,
#30299,#30300,#30301,#30302,#30303,#30304,#30305,#30306,#30307,#30308,#30309,
#30310,#30311,#30312,#30313,#30314,#30315,#30316,#30317,#30318,#30319,#30320,
#30321,#30322,#30323,#30324,#30325,#30326,#30327,#30328,#30329,#30330,#30331,
#30332,#30333,#30334,#30335,#30336,#30337,#30338,#30339,#30340,#30341,#30342,
#30343,#30344,#30345,#30346,#30347,#30348,#30349,#30350,#30351,#30352,#30353,
#30354,#30355,#30356,#30357,#30358,#30359,#30360,#30361,#30362,#30363,#30364,
#30365,#30366,#30367,#30368,#30369,#30370,#30371,#30372,#30373,#30374,#30375,
#30376,#30377,#30378,#30379,#30380,#30381,#30382,#30383,#30384,#30385,#30386,
#30387,#30388,#30389,#30390,#30391,#30392,#30393,#30394,#30395,#30396,#30397,
#30398,#30399,#30400,#30401,#30402,#30403,#30404,#30405,#30406,#30407,#30408,
#30409,#30410,#30411,#30412,#30413,#30414,#30415,#30416,#30417,#30418,#30419,
#30420,#30421),.UNSPECIFIED.,.F.,.F.,(4,2,2,2,2,2,2,2,2,2,2,2,2,2,2,2,2,
2,2,2,2,2,2,2,2,2,2,2,2,2,2,2,2,2,2,2,2,2,2,2,2,2,2,2,2,2,2,2,2,2,2,2,2,
2,2,2,2,2,2,2,2,2,2,2,2,2,2,2,2,2,2,2,2,2,2,2,2,2,2,2,2,2,2,2,2,2,2,2,2,
2,2,2,2,2,2,2,2,2,2,2,2,2,2,2,2,2,2,2,2,2,2,2,2,2,2,2,2,2,2,2,2,2,2,2,2,
2,2,2,2,2,2,2,2,2,2,2,2,2,2,2,2,2,2,2,2,2,2,2,2,2,2,2,2,2,2,2,2,2,2,2,2,
2,2,2,2,2,2,2,2,2,2,2,2,4),(-4.27099291113195,-4.266464075548,-4.25846610092608,
-4.22284627987283,-4.14635119199378,-4.12647918566429,-4.1156252107863,
-4.1062249692604,-4.09442948881289,-4.06926244810299,-3.99011528523554,
-3.96830854467324,-3.95346837490451,-3.94670007660745,-3.94138754650563,
-3.93453804617796,-3.91922072323176,-3.83584698203982,-3.79806031281057,
-3.78460172090393,-3.77498736201644,-3.7649133777217,-3.7490002974327,-3.66762253793479,
-3.62340905519277,-3.61407699980543,-3.60838289395051,-3.60273079761969,
-3.59359710676578,-3.55710914958582,-3.49504748197602,-3.46123755733844,
-3.44822066030172,-3.43867653977123,-3.42845412352372,-3.41179586747999,
-3.34021578835372,-3.30450202143598,-3.29041457656111,-3.27959073875487,
-3.27358360377101,-3.26819858381542,-3.26146880012321,-3.24340801540968,
-3.16369703152365,-3.12642415779366,-3.11301856627768,-3.10341281972251,
-3.09332229619814,-3.07732659932846,-3.00017490859292,-2.95592437902261,
-2.94434122084579,-2.93817978999186,-2.93278823333152,-2.92627709777846,
-2.91016961746748,-2.82829614018731,-2.79071216369558,-2.77727426492673,
-2.76766321536158,-2.75758269966035,-2.74163727572168,-2.65447839340239,
-2.61568461334936,-2.60655987211153,-2.6009094857119,-2.5952131896192,-2.58587111963385,
-2.54248341076492,-2.48584218022855,-2.45347152157958,-2.44063196235395,
-2.43111386450161,-2.420822269382,-2.40381814841478,-2.33682795930802,-2.29836226612503,
-2.27701414368539,-2.26929205754578,-2.26390161694497,-2.25773650472261,
-2.24646125443373,-2.20357032769012,-2.16700473506239,-2.13606478807834,
-2.1135685383291,-2.10222937034251,-2.09284818677295,-2.08161537459901,
-2.05971027894229,-2.02994806028376,-1.99186116166522,-1.94848061949773,
-1.93718865135284,-1.93102000245057,-1.92563076012284,-1.91791598320443,
-1.89662793927592,-1.85835013282568,-1.79100066448291,-1.77401034316466,
-1.76372156539718,-1.75420267842852,-1.74135673226162,-1.7089312763956,
-1.65208699634823,-1.60903933941161,-1.59970120932987,-1.59400579612362,
-1.58835482119974,-1.57922670532033,-1.54037476529806,-1.45326322400859,
-1.43729871276704,-1.4272146040629,-1.41760598670955,-1.40418125471026,
-1.3667153212992,-1.28561399789435,-1.26891543270601,-1.2623120143564,-1.25690172972326,
-1.25080046643083,-1.23951427236896,-1.19797493461773,-1.11624440267149,
-1.10089580363026,-1.0909334432926,-1.08125090775278,-1.06739220833942,
-1.02532173857338,-0.961712205757408,-0.935704859037054,-0.927270708071229,
-0.922304264842921,-0.916601822835038,-0.907227809063822,-0.861559780905584,
-0.780832725859486,-0.765336953352046,-0.75534614776708,-0.745683764837783,
-0.731937761270912,-0.691145525187078,-0.650394722631387,-0.605678622013436,
-0.59432687984587,-0.588146235882582,-0.582761387013465,-0.575073374129285,
-0.553995070382472,-0.516359572221459,-0.448017162750547,-0.43108946189134,
-0.420814126135779,-0.411292149147035,-0.398417761941058,-0.365756510244991,
-0.31199608865096,-0.269864906689862,-0.258619690997774,-0.252461531790012,
-0.247070793091353,-0.239338863655453,-0.217901235764803,-0.179150092056855,
-0.112958905251992,-0.095720350753044,-0.0853839561810169,-0.0758848815394095,
-0.0631639249328616,-0.0421650876622171,-0.000963736707009938),
 .UNSPECIFIED.);
#1509=B_SPLINE_CURVE_WITH_KNOTS('',3,(#30423,#30424,#30425,#30426,#30427,
#30428,#30429,#30430,#30431,#30432,#30433,#30434,#30435,#30436,#30437,#30438,
#30439,#30440,#30441,#30442,#30443,#30444,#30445,#30446,#30447,#30448,#30449,
#30450,#30451,#30452,#30453,#30454,#30455,#30456,#30457,#30458,#30459,#30460,
#30461,#30462,#30463,#30464,#30465,#30466,#30467,#30468,#30469,#30470,#30471,
#30472,#30473,#30474,#30475,#30476,#30477,#30478,#30479,#30480,#30481,#30482,
#30483,#30484,#30485,#30486,#30487,#30488,#30489,#30490,#30491,#30492,#30493,
#30494,#30495,#30496,#30497,#30498,#30499,#30500,#30501,#30502,#30503,#30504,
#30505,#30506,#30507,#30508,#30509,#30510,#30511,#30512,#30513,#30514,#30515,
#30516,#30517,#30518,#30519,#30520,#30521,#30522,#30523,#30524,#30525,#30526,
#30527,#30528,#30529,#30530,#30531,#30532,#30533,#30534,#30535,#30536,#30537,
#30538,#30539,#30540,#30541,#30542,#30543,#30544,#30545,#30546,#30547,#30548,
#30549,#30550,#30551,#30552,#30553,#30554,#30555,#30556,#30557,#30558,#30559,
#30560,#30561,#30562,#30563,#30564,#30565,#30566,#30567,#30568,#30569,#30570,
#30571,#30572,#30573,#30574,#30575,#30576,#30577,#30578,#30579,#30580,#30581,
#30582,#30583,#30584,#30585,#30586,#30587,#30588,#30589,#30590,#30591,#30592,
#30593,#30594,#30595,#30596,#30597,#30598,#30599,#30600,#30601,#30602,#30603,
#30604,#30605,#30606,#30607,#30608,#30609,#30610,#30611,#30612,#30613,#30614,
#30615,#30616,#30617,#30618,#30619,#30620,#30621,#30622,#30623,#30624,#30625,
#30626,#30627,#30628,#30629,#30630,#30631,#30632,#30633),.UNSPECIFIED.,
 .F.,.F.,(4,3,3,3,3,3,3,3,3,3,3,3,3,3,3,3,3,3,3,3,3,3,3,3,3,3,3,3,3,3,3,
3,3,3,3,3,3,3,3,3,3,3,3,3,3,3,3,3,3,3,3,3,3,3,3,3,3,3,3,3,3,3,3,3,3,3,3,
3,3,3,4),(-10.1336107521151,-10.017486513996,-9.89908884700098,-9.88098295102664,
-9.78894122224417,-9.69701994766574,-9.60519272248596,-9.51343026067752,
-9.42170138808768,-9.32998237581279,-9.23824950910818,-9.14642186088112,
-9.05454468136134,-8.96251924502228,-8.89288465592398,-8.80084066000415,
-8.70891707457303,-8.61708749846466,-8.52532263580296,-8.43359133268255,
-8.34186986332005,-8.25013451607053,-8.15830436661682,-8.06642467072822,
-7.97439671930638,-7.90478636082131,-7.81276140508728,-7.72085691549409,
-7.6290464653389,-7.53730069544524,-7.44558845793987,-7.35388600441363,
-7.26216960055253,-7.17035816644906,-7.07849708693619,-6.98648740025403,
-6.91668806571865,-6.82463070078096,-6.73269385008227,-6.64085112820093,
-6.54907335094584,-6.45732927942366,-6.36559520220907,-6.27384742214499,
-6.18200518523899,-6.09011357583558,-5.99807411505652,-5.92858977061598,
-5.83652902859249,-5.74458848180794,-5.6527417543435,-5.56095952832278,
-5.46921073849288,-5.37747168097957,-5.28571866596906,-5.19387083580786,
-5.10197342617237,-5.00992788930343,-4.94049147551332,-4.84856262580369,
-4.75675446703766,-4.66504044681348,-4.57339086587097,-4.4817746379953,
-4.39016790339688,-4.29854681612798,-4.20682949572377,-4.11506200406451,
-4.02314408866267,-3.95239318041066,-3.85042544513253),.UNSPECIFIED.);
#1510=B_SPLINE_CURVE_WITH_KNOTS('',3,(#30635,#30636,#30637,#30638,#30639,
#30640,#30641,#30642,#30643,#30644,#30645,#30646,#30647,#30648,#30649,#30650,
#30651,#30652,#30653,#30654,#30655,#30656,#30657,#30658,#30659,#30660,#30661,
#30662,#30663,#30664,#30665,#30666,#30667,#30668,#30669,#30670,#30671,#30672,
#30673,#30674,#30675,#30676,#30677,#30678,#30679,#30680,#30681,#30682,#30683,
#30684,#30685,#30686,#30687,#30688,#30689,#30690,#30691,#30692,#30693,#30694,
#30695,#30696,#30697,#30698,#30699,#30700,#30701,#30702,#30703,#30704,#30705,
#30706,#30707,#30708,#30709,#30710,#30711,#30712,#30713,#30714,#30715,#30716,
#30717,#30718,#30719,#30720,#30721,#30722,#30723,#30724,#30725,#30726,#30727,
#30728,#30729,#30730,#30731,#30732,#30733,#30734,#30735,#30736,#30737,#30738,
#30739,#30740,#30741,#30742,#30743,#30744,#30745,#30746,#30747,#30748,#30749,
#30750,#30751,#30752,#30753,#30754,#30755,#30756,#30757,#30758,#30759,#30760,
#30761,#30762,#30763,#30764),.UNSPECIFIED.,.F.,.F.,(4,3,3,3,3,3,3,3,3,3,
3,3,3,3,3,3,3,3,3,3,3,3,3,3,3,3,3,3,3,3,3,3,3,3,3,3,3,3,3,3,3,3,3,4),(-3.85042544488316,
-3.75945190295832,-3.66858690682526,-3.5778051867396,-3.48706798717163,
-3.39635049713639,-3.30562792853275,-3.21482096840684,-3.12397023871895,
-3.03297757043926,-2.96429488530799,-2.87216006434223,-2.78014388468642,
-2.68822009607798,-2.59635901488637,-2.50453030368522,-2.41271036638796,
-2.32087562022036,-2.22894526869475,-2.13696478019728,-2.04483612179992,
-1.97619659020533,-1.88505763453743,-1.79403955625527,-1.70311489517017,
-1.61225058727509,-1.52141701981664,-1.43058953389116,-1.33974348102385,
-1.24878999878472,-1.15778146793944,-1.06660647517532,-0.988098295102664,
-0.893598760241011,-0.799235993918247,-0.704988418491972,-0.610850401373128,
-0.516776419061244,-0.422747137412085,-0.328743266848281,-0.234720546922284,
-0.140689749940641,-0.0465973135355168,0.),.UNSPECIFIED.);
#1511=B_SPLINE_CURVE_WITH_KNOTS('',3,(#30768,#30769,#30770,#30771,#30772,
#30773,#30774,#30775,#30776,#30777,#30778,#30779,#30780,#30781,#30782,#30783,
#30784,#30785,#30786,#30787,#30788,#30789,#30790,#30791,#30792,#30793,#30794,
#30795,#30796,#30797,#30798,#30799,#30800,#30801,#30802,#30803,#30804,#30805,
#30806,#30807,#30808,#30809,#30810,#30811,#30812,#30813,#30814,#30815,#30816,
#30817,#30818,#30819,#30820,#30821,#30822,#30823,#30824,#30825,#30826,#30827,
#30828,#30829,#30830,#30831,#30832,#30833,#30834,#30835,#30836,#30837,#30838,
#30839,#30840,#30841,#30842,#30843,#30844,#30845,#30846,#30847,#30848,#30849,
#30850,#30851,#30852,#30853,#30854,#30855,#30856,#30857,#30858,#30859,#30860,
#30861,#30862,#30863,#30864,#30865,#30866,#30867,#30868,#30869,#30870,#30871,
#30872,#30873,#30874,#30875,#30876,#30877,#30878,#30879,#30880,#30881,#30882,
#30883,#30884,#30885,#30886,#30887,#30888,#30889,#30890,#30891,#30892,#30893,
#30894,#30895,#30896,#30897,#30898,#30899,#30900,#30901,#30902,#30903,#30904,
#30905,#30906,#30907,#30908,#30909,#30910,#30911,#30912,#30913,#30914,#30915,
#30916,#30917,#30918,#30919,#30920,#30921,#30922,#30923,#30924,#30925,#30926,
#30927,#30928,#30929,#30930,#30931,#30932,#30933,#30934,#30935,#30936,#30937,
#30938,#30939,#30940,#30941,#30942,#30943,#30944,#30945,#30946,#30947,#30948,
#30949,#30950,#30951,#30952,#30953,#30954,#30955,#30956,#30957),
 .UNSPECIFIED.,.F.,.F.,(4,3,3,3,3,3,3,3,3,3,3,3,3,3,3,3,3,3,3,3,3,3,3,3,
3,3,3,3,3,3,3,3,3,3,3,3,3,3,3,3,3,3,3,3,3,3,3,3,3,3,3,3,3,3,3,3,3,3,3,3,
3,3,3,4),(2.01768719304049,2.10919291876739,2.20058006524129,2.29604441774963,
2.38727725380577,2.47848107942686,2.56968021481692,2.66089897020055,2.75221272523854,
2.84358238516307,2.93508590684933,2.96429488530799,3.0564803252153,3.14854810958801,
3.24052442375695,3.33243923003933,3.42432238696052,3.51619743540617,3.6080879034695,
3.70007461531119,3.79211190089602,3.88429752531008,3.95239318041065,4.04432800087469,
4.13614097705616,4.22785866602567,4.31951017706319,4.41112726861152,4.5027338011772,
4.59435362057034,4.6860680271731,4.77783168822558,4.8697443072756,4.94049147551332,
5.03255291168521,5.12449399472506,5.21634110133997,5.30812346936105,5.39987225566984,
5.49161116437988,5.5833638854286,5.67521119852403,5.76710796646895,5.85915266427401,
5.92858977061598,6.02064516556175,6.11258043755713,6.20442197039764,6.29619914784264,
6.38794298120279,6.47967718160351,6.57142544618978,6.66326872452,6.75516168605004,
6.84720299360337,6.91668806571864,7.00839095829693,7.09997843134294,7.19147474290257,
7.28290406726057,7.37430063642504,7.46567838122102,7.55708352464962,7.59202292841098),
 .UNSPECIFIED.);
#1512=B_SPLINE_CURVE_WITH_KNOTS('',3,(#30959,#30960,#30961,#30962,#30963,
#30964,#30965,#30966,#30967,#30968,#30969),.UNSPECIFIED.,.F.,.F.,(4,1,1,
1,1,1,1,1,4),(7.59202890078445,7.9047863608213,8.89288465592397,9.88098295102663,
10.8690812461293,11.857179541232,12.8452778363346,13.8333761314373,13.8752082355906),
 .UNSPECIFIED.);
#1513=B_SPLINE_CURVE_WITH_KNOTS('',3,(#30971,#30972,#30973,#30974,#30975,
#30976,#30977,#30978,#30979,#30980,#30981,#30982,#30983,#30984,#30985,#30986,
#30987,#30988,#30989,#30990,#30991,#30992,#30993,#30994,#30995,#30996,#30997,
#30998,#30999,#31000,#31001,#31002,#31003,#31004,#31005,#31006,#31007,#31008,
#31009,#31010,#31011,#31012,#31013,#31014,#31015,#31016,#31017,#31018,#31019,
#31020,#31021,#31022,#31023,#31024,#31025,#31026,#31027,#31028,#31029,#31030,
#31031,#31032,#31033,#31034,#31035,#31036,#31037,#31038,#31039,#31040,#31041,
#31042,#31043,#31044,#31045,#31046,#31047,#31048,#31049,#31050,#31051,#31052,
#31053,#31054,#31055,#31056,#31057,#31058,#31059,#31060,#31061,#31062,#31063,
#31064,#31065,#31066,#31067,#31068,#31069,#31070,#31071,#31072,#31073,#31074,
#31075,#31076,#31077,#31078,#31079,#31080,#31081,#31082,#31083,#31084,#31085,
#31086,#31087,#31088,#31089,#31090,#31091,#31092,#31093,#31094,#31095,#31096,
#31097,#31098,#31099,#31100,#31101,#31102,#31103,#31104,#31105,#31106,#31107,
#31108,#31109,#31110,#31111,#31112,#31113,#31114,#31115,#31116,#31117,#31118,
#31119,#31120,#31121,#31122,#31123,#31124,#31125,#31126,#31127,#31128,#31129,
#31130,#31131,#31132,#31133,#31134,#31135,#31136,#31137,#31138,#31139,#31140,
#31141,#31142,#31143,#31144,#31145,#31146,#31147,#31148,#31149,#31150,#31151,
#31152,#31153,#31154,#31155,#31156,#31157,#31158,#31159,#31160,#31161,#31162,
#31163,#31164,#31165,#31166,#31167,#31168,#31169,#31170,#31171,#31172,#31173,
#31174,#31175,#31176,#31177,#31178,#31179,#31180,#31181,#31182,#31183,#31184,
#31185,#31186,#31187,#31188,#31189,#31190,#31191,#31192,#31193,#31194,#31195,
#31196,#31197,#31198,#31199,#31200,#31201,#31202,#31203,#31204,#31205,#31206,
#31207,#31208,#31209,#31210,#31211,#31212,#31213,#31214,#31215,#31216,#31217,
#31218,#31219,#31220,#31221,#31222,#31223,#31224,#31225,#31226,#31227,#31228,
#31229,#31230,#31231,#31232,#31233,#31234,#31235,#31236,#31237,#31238,#31239,
#31240,#31241,#31242,#31243,#31244,#31245,#31246,#31247,#31248,#31249,#31250,
#31251,#31252,#31253,#31254,#31255,#31256,#31257,#31258,#31259,#31260,#31261,
#31262,#31263,#31264,#31265,#31266,#31267,#31268,#31269,#31270,#31271,#31272,
#31273,#31274,#31275,#31276,#31277,#31278,#31279,#31280,#31281,#31282,#31283,
#31284,#31285,#31286,#31287,#31288,#31289,#31290,#31291,#31292,#31293,#31294,
#31295,#31296,#31297,#31298,#31299,#31300,#31301,#31302,#31303,#31304,#31305,
#31306,#31307,#31308,#31309,#31310,#31311,#31312),.UNSPECIFIED.,.F.,.F.,
(4,2,2,2,2,2,2,2,2,2,2,2,2,2,2,2,2,2,2,2,2,2,2,2,2,2,2,2,2,2,2,2,2,2,2,
2,2,2,2,2,2,2,2,2,2,2,2,2,2,2,2,2,2,2,2,2,2,2,2,2,2,2,2,2,2,2,2,2,2,2,2,
2,2,2,2,2,2,2,2,2,2,2,2,2,2,2,2,2,2,2,2,2,2,2,2,2,2,2,2,2,2,2,2,2,2,2,2,
2,2,2,2,2,2,2,2,2,2,2,2,2,2,2,2,2,2,2,2,2,2,2,2,2,2,2,2,2,2,2,2,2,2,2,2,
2,2,2,2,2,2,2,2,2,2,2,2,2,2,2,2,2,2,2,2,2,2,2,2,2,2,2,4),(-4.27089550160095,
-4.26517093009983,-4.18123377942425,-4.13980108553207,-4.12599656693906,
-4.11632340353083,-4.10634692432074,-4.09092671351489,-4.00973421500502,
-3.96441499067419,-3.95505115903307,-3.94935053670693,-3.94438229721522,
-3.93593906273184,-3.90983752462709,-3.84626927776244,-3.8041967477589,
-3.79033657123392,-3.78065340802285,-3.77069077844753,-3.75534238978773,
-3.67365803391384,-3.63212870657385,-3.62084368969843,-3.61474250017146,
-3.60933198563307,-3.60272781227625,-3.58602573065649,-3.5048816664091,
-3.46740131169902,-3.45397454743088,-3.44436565340207,-3.43428232848595,
-3.41832126817335,-3.34092267968528,-3.29682961633398,-3.28526354800635,
-3.27910572276471,-3.27371342578226,-3.26719761375624,-3.25105995527236,
-3.19051813212376,-3.1446368186399,-3.12453272638999,-3.11363457299039,
-3.10423849812787,-3.09250395483874,-3.06770642499166,-2.98799946304298,
-2.95592737000991,-2.94719050940168,-2.94161991935152,-2.93654941666119,
-2.92754293325874,-2.8944870210215,-2.829609429513,-2.7951264879124,-2.78202987735722,
-2.772473569767,-2.76228023253695,-2.74576771617694,-2.66525527218807,-2.62467953748322,
-2.61350269589351,-2.60742321570966,-2.60200449469963,-2.59409760503653,
-2.57287744220049,-2.51046474718343,-2.462199071591,-2.44788001265044,-2.43811287274056,
-2.42825372293763,-2.41344534966472,-2.35579901995858,-2.30724301837016,
-2.28301056581025,-2.27495728114019,-2.2695144563339,-2.26349655763637,
-2.25262026322153,-2.19237202379743,-2.13597359955294,-2.11694124915784,
-2.10614409607742,-2.09682750617894,-2.08499817093511,-2.05962298215849,
-2.02252994071289,-1.96288673037515,-1.94578058017786,-1.93911857689346,
-1.9336955680881,-1.92762955663532,-1.91651694983403,-1.87649278064731,
-1.79783370866518,-1.77995205978646,-1.7694868830076,-1.76002277520293,
-1.74757650557126,-1.71813133022915,-1.67071097035882,-1.61772008756554,
-1.60645360980525,-1.60035651507718,-1.59494524779244,-1.58708134607396,
-1.56454638328828,-1.52220498480293,-1.46078901403587,-1.4436628033303,
-1.43334763739714,-1.4238392855057,-1.41106156139208,-1.3791631951668,-1.32414037672917,
-1.28223715222047,-1.27099909595084,-1.26484220774146,-1.25945011139248,
-1.25171318800143,-1.2302420421733,-1.19138861738065,-1.1249430073584,-1.10791202952862,
-1.09761573810651,-1.08810065055242,-1.07527651756836,-1.04301705294725,
-0.986751959088537,-0.942925866470926,-0.933584792995982,-0.927889083643446,
-0.922239411376962,-0.913115784663209,-0.874345994377888,-0.787093790670101,
-0.771161480803704,-0.761084405453528,-0.751473390862406,-0.738030012317473,
-0.700375138696203,-0.617897070267363,-0.602099374380554,-0.595138008132656,
-0.589817498414164,-0.583254470744053,-0.569569680107619,-0.499819830595,
-0.448627527377693,-0.434018654330641,-0.425179199719389,-0.415543495170319,
-0.401952960884438,-0.362824529424473,-0.320821812002546,-0.275403697620598,
-0.264007693896237,-0.25781770456701,-0.252435726399069,-0.244766763022211,
-0.223838005099873,-0.186658553656164,-0.118079923396639,-0.100927462738524,
-0.0906075946626851,-0.0811018260956066,-0.0683382198453528,-0.0467905167351216,
-0.000959392972239935),.UNSPECIFIED.);
#1514=B_SPLINE_CURVE_WITH_KNOTS('',3,(#31314,#31315,#31316,#31317,#31318,
#31319,#31320,#31321,#31322,#31323,#31324,#31325,#31326,#31327,#31328,#31329,
#31330,#31331,#31332,#31333,#31334,#31335,#31336,#31337,#31338,#31339,#31340,
#31341,#31342,#31343,#31344,#31345,#31346,#31347,#31348,#31349,#31350,#31351,
#31352,#31353,#31354,#31355,#31356,#31357,#31358,#31359,#31360,#31361,#31362,
#31363,#31364,#31365,#31366,#31367,#31368,#31369,#31370,#31371,#31372,#31373,
#31374,#31375,#31376,#31377,#31378,#31379,#31380,#31381,#31382,#31383,#31384,
#31385,#31386,#31387,#31388,#31389,#31390,#31391,#31392,#31393,#31394,#31395,
#31396,#31397,#31398,#31399,#31400,#31401,#31402,#31403,#31404,#31405,#31406,
#31407,#31408,#31409,#31410,#31411,#31412,#31413,#31414,#31415,#31416,#31417,
#31418,#31419,#31420,#31421,#31422,#31423,#31424,#31425,#31426,#31427,#31428,
#31429,#31430,#31431,#31432,#31433,#31434,#31435,#31436,#31437,#31438,#31439,
#31440,#31441,#31442,#31443,#31444,#31445,#31446,#31447,#31448,#31449,#31450,
#31451,#31452,#31453,#31454,#31455,#31456,#31457,#31458,#31459,#31460,#31461,
#31462,#31463,#31464,#31465,#31466,#31467,#31468,#31469,#31470,#31471,#31472,
#31473,#31474,#31475,#31476,#31477,#31478,#31479,#31480,#31481,#31482,#31483,
#31484,#31485,#31486,#31487,#31488,#31489,#31490,#31491,#31492,#31493,#31494,
#31495,#31496,#31497,#31498,#31499,#31500,#31501,#31502,#31503,#31504,#31505,
#31506,#31507,#31508,#31509,#31510,#31511,#31512,#31513,#31514,#31515,#31516,
#31517,#31518,#31519,#31520,#31521,#31522,#31523,#31524,#31525,#31526,#31527,
#31528,#31529,#31530,#31531,#31532,#31533,#31534,#31535,#31536,#31537,#31538,
#31539,#31540,#31541,#31542,#31543,#31544,#31545,#31546,#31547,#31548,#31549,
#31550,#31551,#31552,#31553,#31554,#31555,#31556,#31557,#31558,#31559,#31560,
#31561,#31562,#31563,#31564,#31565,#31566,#31567,#31568,#31569,#31570,#31571,
#31572,#31573,#31574,#31575,#31576,#31577,#31578,#31579,#31580,#31581,#31582,
#31583,#31584,#31585,#31586,#31587,#31588,#31589,#31590,#31591,#31592,#31593,
#31594,#31595,#31596,#31597,#31598,#31599,#31600,#31601,#31602,#31603,#31604,
#31605,#31606,#31607,#31608,#31609,#31610,#31611,#31612,#31613,#31614,#31615,
#31616,#31617,#31618,#31619,#31620,#31621,#31622,#31623,#31624,#31625,#31626,
#31627,#31628,#31629,#31630,#31631,#31632,#31633,#31634,#31635,#31636,#31637,
#31638,#31639,#31640,#31641,#31642,#31643,#31644,#31645,#31646,#31647,#31648,
#31649,#31650,#31651,#31652,#31653,#31654,#31655,#31656,#31657,#31658,#31659,
#31660,#31661),.UNSPECIFIED.,.F.,.F.,(4,2,2,2,2,2,2,2,2,2,2,2,2,2,2,2,2,
2,2,2,2,2,2,2,2,2,2,2,2,2,2,2,2,2,2,2,2,2,2,2,2,2,2,2,2,2,2,2,2,2,2,2,2,
2,2,2,2,2,2,2,2,2,2,2,2,2,2,2,2,2,2,2,2,2,2,2,2,2,2,2,2,2,2,2,2,2,2,2,2,
2,2,2,2,2,2,2,2,2,2,2,2,2,2,2,2,2,2,2,2,2,2,2,2,2,2,2,2,2,2,2,2,2,2,2,2,
2,2,2,2,2,2,2,2,2,2,2,2,2,2,2,2,2,2,2,2,2,2,2,2,2,2,2,2,2,2,2,2,2,2,2,2,
2,2,2,2,2,2,2,2,2,2,2,2,4),(-4.27016132765278,-4.2112933202812,-4.20202621727073,
-4.1941439983737,-4.18872991176856,-4.18264127270548,-4.17141590587009,
-4.11595626621906,-4.07009735564466,-4.04121112713488,-4.02884459941924,
-4.01939047852455,-4.00888580743757,-3.99080278362926,-3.91246175026595,
-3.87253667468467,-3.86143619608755,-3.85537283050901,-3.84994924814343,
-3.84200841905082,-3.82052645479384,-3.74461384980817,-3.70794553426337,
-3.69460505185852,-3.68501080169383,-3.67490140660616,-3.6588067905035,
-3.57238481555369,-3.53320348741931,-3.52406179256984,-3.51840823148544,
-3.51271651486387,-3.50339420602896,-3.46168860634024,-3.42168424363258,
-3.38991116432299,-3.36700456619755,-3.3555932551898,-3.3462116208593,-3.33504805244734,
-3.31418300921281,-3.23959808303002,-3.20084933621331,-3.18988740258155,
-3.18385203640618,-3.17847855423334,-3.17179972801083,-3.15454027921675,
-3.07404034493659,-3.03665243215943,-3.02323521415283,-3.01362784597951,
-3.00354148483392,-2.98756536511546,-2.90055980055357,-2.86168713740885,
-2.85255900884707,-2.84690804108186,-2.84121277593298,-2.83187493925176,
-2.78905785216877,-2.73199844915205,-2.69951029298848,-2.68665618080192,
-2.67713625246302,-2.66685107389063,-2.64987789974936,-2.5823088934531,
-2.54421466958434,-2.5229862880412,-2.51527921356779,-2.50989108551139,
-2.503718853469,-2.49240941414251,-2.44862204888924,-2.41009652685683,-2.36652312301965,
-2.35253863718015,-2.34283295534659,-2.33290013246453,-2.31770674073402,
-2.23497999469098,-2.19065164227658,-2.18131587386556,-2.17562088259492,
-2.1706483244467,-2.1621820429767,-2.13581900001301,-2.07622559070618,-2.03160467454466,
-2.01724075066862,-2.00844146095637,-1.99876623410861,-1.98495524315478,
-1.9434547363968,-1.90177199693798,-1.85868848206746,-1.8474076777392,-1.84124133775524,
-1.83585130554631,-1.82813153975872,-1.80680383850205,-1.7684028924635,
-1.70124533199585,-1.68424494671686,-1.67395405996442,-1.66443572907638,
-1.65159442865682,-1.61920668485835,-1.56249664292403,-1.51926539518677,
-1.50992598662808,-1.50423025552043,-1.49857949384636,-1.48945247207566,
-1.45062538199959,-1.36346436946267,-1.34750959691089,-1.33742737246164,
-1.32781763989175,-1.31438646629687,-1.27685908989308,-1.19532435209695,
-1.17898205826183,-1.17243380662568,-1.16703497676674,-1.16089863805806,
-1.14943922239367,-1.10633803877844,-1.02724840718897,-1.01151465493938,
-1.00147641792631,-0.991842302640632,-0.978264214302576,-0.939271129256164,
-0.896531646657189,-0.851618226349477,-0.840254431533927,-0.834070969216295,
-0.828686668497398,-0.821003440626908,-0.79996425555181,-0.762450604030013,
-0.693891345236649,-0.676975752088803,-0.666702592654482,-0.657179400770686,
-0.644298369146377,-0.611586782263747,-0.563397731297679,-0.512409737917154,
-0.502906066999759,-0.497175980974361,-0.491557451777441,-0.482582854080362,
-0.446723656507844,-0.370051694683377,-0.346049064324514,-0.334448777622994,
-0.325061346118745,-0.314061961633378,-0.293416407200125,-0.266069109142431,
-0.225172804988896,-0.180290567047164,-0.168929076004839,-0.16274629938351,
-0.157362182986379,-0.149678652385427,-0.12863492964186,-0.0911060083721691,
-0.0216916045340881,-0.00927743633556165,-0.000959649626902801),
 .UNSPECIFIED.);
#1515=B_SPLINE_CURVE_WITH_KNOTS('',3,(#31663,#31664,#31665,#31666,#31667,
#31668,#31669,#31670,#31671,#31672,#31673,#31674,#31675,#31676,#31677,#31678,
#31679,#31680,#31681,#31682,#31683,#31684,#31685,#31686,#31687,#31688,#31689,
#31690,#31691,#31692,#31693,#31694,#31695,#31696,#31697,#31698,#31699,#31700,
#31701,#31702,#31703,#31704,#31705,#31706,#31707,#31708,#31709,#31710,#31711,
#31712,#31713,#31714,#31715,#31716,#31717,#31718,#31719,#31720,#31721,#31722,
#31723,#31724,#31725,#31726,#31727,#31728,#31729,#31730,#31731,#31732,#31733,
#31734,#31735,#31736,#31737,#31738,#31739,#31740,#31741,#31742,#31743,#31744,
#31745,#31746,#31747,#31748,#31749,#31750,#31751,#31752,#31753,#31754,#31755,
#31756,#31757,#31758,#31759,#31760,#31761,#31762,#31763,#31764,#31765,#31766,
#31767,#31768,#31769,#31770,#31771,#31772,#31773,#31774,#31775,#31776,#31777,
#31778,#31779,#31780,#31781,#31782,#31783,#31784,#31785,#31786,#31787,#31788,
#31789,#31790,#31791,#31792,#31793,#31794,#31795,#31796,#31797,#31798,#31799,
#31800,#31801,#31802,#31803,#31804,#31805,#31806,#31807,#31808,#31809,#31810,
#31811,#31812,#31813,#31814,#31815,#31816,#31817,#31818,#31819,#31820,#31821,
#31822,#31823,#31824,#31825,#31826,#31827,#31828,#31829,#31830,#31831,#31832,
#31833,#31834,#31835,#31836,#31837,#31838,#31839,#31840,#31841,#31842,#31843,
#31844,#31845,#31846,#31847,#31848,#31849,#31850,#31851,#31852,#31853,#31854,
#31855,#31856,#31857,#31858,#31859,#31860,#31861,#31862,#31863,#31864,#31865,
#31866,#31867,#31868,#31869,#31870,#31871,#31872,#31873,#31874,#31875,#31876,
#31877,#31878,#31879,#31880,#31881,#31882,#31883,#31884,#31885,#31886,#31887,
#31888,#31889,#31890,#31891,#31892,#31893,#31894,#31895,#31896,#31897,#31898,
#31899,#31900,#31901,#31902,#31903,#31904,#31905,#31906,#31907,#31908,#31909,
#31910,#31911,#31912,#31913,#31914,#31915,#31916,#31917,#31918,#31919,#31920,
#31921,#31922,#31923,#31924,#31925,#31926,#31927,#31928,#31929,#31930,#31931,
#31932,#31933,#31934,#31935,#31936,#31937,#31938,#31939,#31940,#31941,#31942,
#31943,#31944,#31945,#31946,#31947,#31948,#31949,#31950,#31951,#31952,#31953,
#31954,#31955,#31956,#31957,#31958,#31959,#31960,#31961,#31962,#31963,#31964,
#31965,#31966,#31967,#31968,#31969,#31970,#31971,#31972,#31973,#31974,#31975,
#31976,#31977,#31978,#31979,#31980,#31981,#31982,#31983,#31984,#31985,#31986,
#31987,#31988,#31989,#31990,#31991,#31992,#31993,#31994,#31995,#31996,#31997,
#31998,#31999,#32000,#32001,#32002,#32003,#32004,#32005,#32006),
 .UNSPECIFIED.,.F.,.F.,(4,2,2,2,2,2,2,2,2,2,2,2,2,2,2,2,2,2,2,2,2,2,2,2,
2,2,2,2,2,2,2,2,2,2,2,2,2,2,2,2,2,2,2,2,2,2,2,2,2,2,2,2,2,2,2,2,2,2,2,2,
2,2,2,2,2,2,2,2,2,2,2,2,2,2,2,2,2,2,2,2,2,2,2,2,2,2,2,2,2,2,2,2,2,2,2,2,
2,2,2,2,2,2,2,2,2,2,2,2,2,2,2,2,2,2,2,2,2,2,2,2,2,2,2,2,2,2,2,2,2,2,2,2,
2,2,2,2,2,2,2,2,2,2,2,2,2,2,2,2,2,2,2,2,2,2,2,2,2,2,2,2,2,2,2,2,2,2,2,2,
2,2,2,4),(-4.27067861780142,-4.26537209255245,-4.2585959461785,-4.24767254749016,
-4.2272873009378,-4.14877591485979,-4.1100152384294,-4.10089250779693,-4.09524278424705,
-4.0895465358244,-4.08020356065768,-4.03645029757843,-3.98008273700803,
-3.94779107292332,-3.93496210902089,-3.92544603102557,-3.9151511372335,
-3.8981282388189,-3.83157514788041,-3.79283220017504,-3.77139620361843,
-3.76366362016086,-3.75827192944369,-3.75211263088738,-3.74086362864568,
-3.69870262149952,-3.64491001640648,-3.612235334683,-3.59935827587587,-3.58983546157847,
-3.57956035284238,-3.56263564160191,-3.48037186337755,-3.43882949132267,
-3.42958929142758,-3.42391472987895,-3.41824391805605,-3.40902113769835,
-3.37058355451726,-3.31012289936565,-3.27671842366527,-3.26375076897159,
-3.25421423664366,-3.24397366264229,-3.2272235896755,-3.14704924538102,
-3.10657471823022,-3.09540963246718,-3.08933259788933,-3.08391304973467,
-3.07600078710977,-3.05474005296049,-2.97857787688043,-2.94186473405767,
-2.92851816702505,-2.91892189858174,-2.9088124499461,-2.89272237261806,
-2.81627597515997,-2.77158303482065,-2.75995292357337,-2.75378200331587,
-2.74839310432892,-2.74068196566705,-2.72092399617808,-2.64312888050789,
-2.60614988584254,-2.59277503994756,-2.58317420700646,-2.57307382669278,
-2.55702914255223,-2.47034221775661,-2.43129187752549,-2.42215515245212,
-2.41650215942054,-2.41150086844904,-2.40287218523823,-2.37489242807534,
-2.30542949929917,-2.26995189861576,-2.25674068927914,-2.24716603637757,
-2.23701182531611,-2.22069747797986,-2.13532446255829,-2.09574400439092,
-2.08647722656653,-2.08079654930171,-2.07512991249371,-2.06593018061556,
-2.02546182071473,-1.94127043328855,-1.92470967133765,-1.91450603838393,
-1.90495281590672,-1.89188077529545,-1.85760965269131,-1.79362825149057,
-1.75955145527578,-1.75050118153279,-1.74486632306109,-1.73915366613821,
-1.72973266242786,-1.68217952637543,-1.60420617264449,-1.58831454344002,
-1.57824527411859,-1.56862946665225,-1.55515883449638,-1.51724310429662,
-1.4328055655712,-1.41974119733246,-1.41322582650967,-1.40783379076601,
-1.40167652356429,-1.39011240187944,-1.34604199136839,-1.26851379033042,
-1.25255893715664,-1.24247659978013,-1.23286674676947,-1.21943538242946,
-1.18190618232596,-1.10034676426858,-1.08403056184597,-1.07748570490152,
-1.07208649134622,-1.06594356706457,-1.05446086523337,-1.01116088618642,
-0.932468286232639,-0.916684793513309,-0.906634391221016,-0.897001873209618,
-0.883448318572225,-0.844734783202608,-0.778217793336078,-0.751203692416926,
-0.742683469744678,-0.737701932261014,-0.73202756107304,-0.722772157987534,
-0.680725957217797,-0.60569387976744,-0.586940432742266,-0.575279095677745,
-0.565895421002981,-0.554960670205056,-0.534630646378481,-0.490184825086574,
-0.431409910496945,-0.413161728988384,-0.405684177077472,-0.400329386632062,
-0.394039913575364,-0.381802615811599,-0.365163349046766,-0.316253129528295,
-0.259091569371166,-0.244197034621773,-0.234320187011864,-0.224565361362386,
-0.210319249629481,-0.163153509877998,-0.0951768006497754,-0.0773589536685485,
-0.0706388543599413,-0.0652493634815464,-0.0592081465942081,-0.0527098387532521,
-0.0374059006265811,-0.000998075931179162),.UNSPECIFIED.);
#1516=B_SPLINE_CURVE_WITH_KNOTS('',3,(#32007,#32008,#32009,#32010,#32011,
#32012,#32013,#32014,#32015,#32016,#32017,#32018,#32019,#32020,#32021,#32022,
#32023,#32024,#32025,#32026,#32027,#32028,#32029,#32030,#32031,#32032,#32033,
#32034,#32035,#32036,#32037,#32038,#32039,#32040,#32041,#32042,#32043,#32044,
#32045,#32046,#32047,#32048,#32049,#32050,#32051,#32052,#32053,#32054,#32055,
#32056,#32057,#32058,#32059,#32060,#32061,#32062,#32063,#32064,#32065,#32066,
#32067,#32068,#32069,#32070,#32071,#32072,#32073,#32074,#32075,#32076,#32077,
#32078,#32079,#32080,#32081,#32082,#32083,#32084,#32085,#32086,#32087,#32088,
#32089,#32090,#32091,#32092,#32093,#32094,#32095,#32096,#32097,#32098,#32099,
#32100,#32101,#32102,#32103,#32104,#32105,#32106,#32107,#32108,#32109,#32110,
#32111,#32112,#32113,#32114,#32115,#32116,#32117,#32118,#32119,#32120,#32121,
#32122,#32123,#32124,#32125,#32126,#32127,#32128,#32129,#32130,#32131,#32132,
#32133,#32134,#32135,#32136,#32137,#32138,#32139,#32140,#32141,#32142,#32143,
#32144,#32145,#32146,#32147,#32148,#32149,#32150,#32151,#32152,#32153,#32154,
#32155,#32156,#32157,#32158,#32159,#32160,#32161,#32162,#32163,#32164,#32165,
#32166,#32167,#32168,#32169,#32170,#32171,#32172,#32173,#32174,#32175,#32176,
#32177,#32178,#32179,#32180,#32181,#32182,#32183,#32184,#32185,#32186,#32187,
#32188,#32189,#32190,#32191,#32192,#32193,#32194,#32195,#32196,#32197,#32198,
#32199),.UNSPECIFIED.,.F.,.F.,(4,3,3,3,3,3,3,3,3,3,3,3,3,3,3,3,3,3,3,3,
3,3,3,3,3,3,3,3,3,3,3,3,3,3,3,3,3,3,3,3,3,3,3,3,3,3,3,3,3,3,3,3,3,3,3,3,
3,3,3,3,3,3,3,3,4),(51.5743200788773,51.6649277828395,51.7554520784406,
51.8459317845929,51.9363919168048,52.026857467403,52.1174090872171,52.2080050728962,
52.298745910618,52.3692096404412,52.4611387007398,52.5529470704279,52.644661301644,
52.7363110928568,52.8279275304985,52.9195344741252,53.0111557694502,53.1028732951607,
53.1946409909151,53.2865591063539,53.3573079355438,53.4495092586262,53.5415897364067,
53.6335755674778,53.7254950911433,53.8173800174986,53.9092538900192,54.0011402370549,
54.0931182965783,54.1851443977839,54.2773148220531,54.3454062306465,54.4375405184005,
54.5295561626478,54.6214794144077,54.7133399588713,54.8051681336385,54.8969875354656,
54.9888217477981,55.0807515713472,55.1727315343686,55.2648596767482,55.3335045257492,
55.4246445692492,55.5156637380849,55.606589491441,55.6974548906982,55.7882895490156,
55.8791181244371,55.9699652645748,56.0609198246063,56.1519294300429,56.2431054808996,
56.3216028208518,56.4161015484885,56.5104635039292,56.6047102669304,56.6988474743701,
56.7929206502446,56.886949130588,56.9809522068713,57.0749741487432,57.1690041771278,
57.2630958659899,57.3097011159545),.UNSPECIFIED.);
#1517=B_SPLINE_CURVE_WITH_KNOTS('',3,(#32202,#32203,#32204,#32205,#32206,
#32207,#32208,#32209,#32210,#32211,#32212,#32213,#32214,#32215,#32216,#32217,
#32218,#32219,#32220,#32221,#32222,#32223,#32224,#32225,#32226,#32227,#32228,
#32229,#32230,#32231,#32232,#32233,#32234,#32235,#32236,#32237,#32238,#32239,
#32240,#32241,#32242,#32243,#32244,#32245,#32246,#32247,#32248,#32249,#32250,
#32251,#32252,#32253,#32254,#32255,#32256,#32257,#32258,#32259,#32260,#32261,
#32262,#32263,#32264,#32265,#32266,#32267,#32268,#32269,#32270,#32271,#32272,
#32273,#32274,#32275,#32276,#32277,#32278,#32279,#32280,#32281,#32282,#32283,
#32284,#32285,#32286,#32287,#32288,#32289,#32290,#32291,#32292,#32293,#32294,
#32295,#32296,#32297,#32298,#32299,#32300,#32301,#32302,#32303,#32304,#32305,
#32306,#32307,#32308,#32309,#32310,#32311,#32312,#32313,#32314,#32315,#32316,
#32317,#32318,#32319,#32320,#32321,#32322,#32323,#32324,#32325,#32326,#32327,
#32328,#32329,#32330,#32331,#32332,#32333,#32334,#32335,#32336,#32337,#32338,
#32339,#32340,#32341,#32342,#32343,#32344,#32345,#32346,#32347,#32348,#32349),
 .UNSPECIFIED.,.F.,.F.,(4,3,3,3,3,3,3,3,3,3,3,3,3,3,3,3,3,3,3,3,3,3,3,3,
3,3,3,3,3,3,3,3,3,3,3,3,3,3,3,3,3,3,3,3,3,3,3,3,3,4),(17.9338553089788,
18.0215439040059,18.1091610711696,18.1967367502352,18.2842926731967,18.3718494470166,
18.4594276742157,18.5470991128665,18.6348218107834,18.7226771653382,18.774225888535,
18.8620580791135,18.949779824276,19.0374141030197,19.1280278630969,19.2155641927871,
19.3030877407944,19.390619143229,19.4781790367439,19.5658354343701,19.6535494818897,
19.7413879044324,19.7623241836377,19.8501737049915,19.9379129932197,20.0255650044576,
20.1161721887429,20.2037266088798,20.2912683483248,20.3788180234578,20.4663962512482,
20.5540709827269,20.6418033849509,20.7296600546718,20.7504224787404,20.8382696052408,
20.9260065029351,21.0136561309453,21.1042642113075,21.1918162824243,21.2793556897791,
21.3669030524404,21.454478990082,21.5421514761848,21.629881656649,21.7177361559214,
21.738520773843,21.851595669962,21.9625651261396,21.991148574894),
 .UNSPECIFIED.);
#1518=B_SPLINE_CURVE_WITH_KNOTS('',3,(#32350,#32351,#32352,#32353,#32354,
#32355,#32356,#32357,#32358,#32359,#32360,#32361,#32362,#32363,#32364,#32365,
#32366,#32367,#32368,#32369,#32370,#32371,#32372,#32373,#32374,#32375,#32376,
#32377,#32378,#32379,#32380,#32381,#32382,#32383,#32384,#32385,#32386,#32387,
#32388,#32389,#32390,#32391,#32392,#32393,#32394,#32395,#32396,#32397,#32398,
#32399,#32400,#32401,#32402,#32403,#32404,#32405,#32406,#32407,#32408,#32409,
#32410,#32411,#32412,#32413,#32414,#32415,#32416,#32417,#32418,#32419,#32420,
#32421,#32422,#32423,#32424,#32425,#32426,#32427,#32428,#32429,#32430,#32431),
 .UNSPECIFIED.,.F.,.F.,(4,3,3,3,3,3,3,3,3,3,3,3,3,3,3,3,3,3,3,3,3,3,3,3,
3,3,3,4),(21.9911485751285,22.07782353564,22.1644492228726,22.2510509271146,
22.3376501732404,22.4242684800746,22.5109767570387,22.5977358546946,22.6846237111792,
22.7266190689457,22.8144654301682,22.9022015361397,22.9898503470852,23.0804587242056,
23.1680099200613,23.2555484320559,23.3430948801545,23.4306698849134,23.5183414155381,
23.6060706262079,23.6939241420068,23.7147173640484,23.8025623224055,23.8903011418041,
23.9779408712635,24.0655226220768,24.1530722511086,24.2165026702176),
 .UNSPECIFIED.);
#1519=B_SPLINE_CURVE_WITH_KNOTS('',3,(#32433,#32434,#32435,#32436,#32437,
#32438,#32439,#32440,#32441,#32442,#32443,#32444,#32445,#32446,#32447,#32448,
#32449,#32450,#32451,#32452,#32453,#32454,#32455,#32456,#32457,#32458,#32459,
#32460,#32461,#32462,#32463,#32464,#32465,#32466,#32467,#32468,#32469,#32470,
#32471,#32472,#32473,#32474,#32475,#32476,#32477,#32478,#32479,#32480,#32481,
#32482,#32483,#32484,#32485,#32486,#32487,#32488,#32489,#32490,#32491,#32492,
#32493,#32494,#32495,#32496,#32497,#32498,#32499,#32500,#32501,#32502,#32503,
#32504,#32505,#32506,#32507,#32508,#32509,#32510,#32511),.UNSPECIFIED.,
 .F.,.F.,(4,3,3,3,3,3,3,3,3,3,3,3,3,3,3,3,3,3,3,3,3,3,3,3,3,3,4),(21.9911485753101,
22.0943756280195,22.1991438177791,22.3039120075388,22.3917615121359,22.4795007834467,
22.5671527776282,22.6577599682548,22.745314371099,22.832856093194,22.9204057509385,
23.0079839613211,23.09565867545,23.1833910603384,23.2712477128744,23.2920103026415,
23.3798611821018,23.46760091707,23.5552524705408,23.6428372873228,23.7303867997398,
23.8179216416748,23.9054624312907,23.9930721519065,24.0807198637846,24.168477835605,
24.2162169687424),.UNSPECIFIED.);
#1520=B_SPLINE_CURVE_WITH_KNOTS('',3,(#32512,#32513,#32514,#32515,#32516,
#32517,#32518,#32519,#32520,#32521,#32522,#32523,#32524,#32525,#32526,#32527,
#32528,#32529,#32530,#32531,#32532,#32533,#32534,#32535,#32536,#32537,#32538,
#32539,#32540,#32541,#32542,#32543,#32544,#32545,#32546,#32547,#32548,#32549,
#32550,#32551,#32552,#32553,#32554,#32555,#32556,#32557,#32558,#32559,#32560,
#32561,#32562,#32563,#32564,#32565,#32566,#32567,#32568,#32569,#32570,#32571,
#32572,#32573,#32574,#32575,#32576,#32577,#32578,#32579,#32580,#32581,#32582,
#32583,#32584,#32585,#32586,#32587,#32588,#32589,#32590,#32591,#32592,#32593,
#32594,#32595,#32596,#32597,#32598,#32599,#32600,#32601,#32602,#32603,#32604,
#32605,#32606,#32607,#32608,#32609,#32610,#32611,#32612,#32613,#32614,#32615,
#32616,#32617,#32618,#32619,#32620,#32621,#32622,#32623,#32624,#32625,#32626,
#32627,#32628,#32629,#32630,#32631,#32632,#32633,#32634,#32635,#32636,#32637,
#32638,#32639,#32640,#32641,#32642,#32643,#32644,#32645,#32646,#32647,#32648,
#32649,#32650,#32651,#32652,#32653,#32654,#32655,#32656,#32657,#32658,#32659),
 .UNSPECIFIED.,.F.,.F.,(4,3,3,3,3,3,3,3,3,3,3,3,3,3,3,3,3,3,3,3,3,3,3,3,
3,3,3,3,3,3,3,3,3,3,3,3,3,3,3,3,3,3,3,3,3,3,3,3,3,4),(17.9330836177785,
18.0207920357673,18.1085927320213,18.1964419063721,18.2844284749951,18.3515188271282,
18.4392641415273,18.5268979148076,18.6144432387119,18.7050899741517,18.7925354599518,
18.8799676203594,18.9674071884555,19.0548748976097,19.1424390496895,19.2300607078759,
19.3178072255313,19.3396171222308,19.4274832824099,19.5152392634936,19.6029080003411,
19.6935089274652,19.7810800438035,19.8686384385576,19.9562047092435,20.0437994539135,
20.1314905019181,20.2192391220966,20.3071117434506,20.3277154173335,20.4155758115876,
20.503326236269,20.5909896323957,20.6815926424008,20.7691589952233,20.8567128499074,
20.9442748102051,21.0318654805741,21.1195528264309,21.2072979580046,21.2951674297034,
21.3158137124362,21.4033376679948,21.4907559825063,21.5780897484102,21.6653599877815,
21.7525970742007,21.8398129836218,21.9270557282901,21.9911485751285),
 .UNSPECIFIED.);
#1521=B_SPLINE_CURVE_WITH_KNOTS('',3,(#32904,#32905,#32906,#32907,#32908,
#32909,#32910,#32911,#32912,#32913,#32914,#32915,#32916,#32917,#32918,#32919,
#32920,#32921,#32922,#32923,#32924,#32925,#32926,#32927,#32928,#32929,#32930,
#32931,#32932,#32933,#32934,#32935,#32936,#32937,#32938,#32939,#32940,#32941,
#32942,#32943,#32944,#32945,#32946,#32947,#32948,#32949,#32950,#32951,#32952,
#32953,#32954,#32955,#32956,#32957,#32958,#32959,#32960,#32961,#32962,#32963,
#32964,#32965,#32966,#32967,#32968,#32969,#32970,#32971,#32972,#32973,#32974,
#32975,#32976,#32977,#32978,#32979,#32980,#32981,#32982,#32983,#32984,#32985,
#32986,#32987,#32988,#32989,#32990,#32991,#32992,#32993,#32994,#32995,#32996,
#32997,#32998,#32999,#33000),.UNSPECIFIED.,.F.,.F.,(4,3,3,3,3,3,3,3,3,3,
3,3,3,3,3,3,3,3,3,3,3,3,3,3,3,3,3,3,3,3,3,3,4),(0.,0.0371582535577247,0.0748617881856257,
0.112715125949566,0.148381967323058,0.15512741629588,0.16010500092411,0.197066207831433,
0.233851108508262,0.269797208916457,0.300074600064785,0.306206454212408,
0.31126514519064,0.346541882858749,0.381619422387025,0.389927986336217,
0.425938753218444,0.446125992369769,0.452219114700122,0.457530832114577,
0.49237174121568,0.527498764190727,0.562156271439185,0.587436666429045,
0.594976497048954,0.600634884631193,0.63468210758544,0.667951164906714,
0.675839565696752,0.683329187302406,0.715805593816627,0.746543832162165,
0.76075981699454),.UNSPECIFIED.);
#1522=B_SPLINE_CURVE_WITH_KNOTS('',3,(#33001,#33002,#33003,#33004,#33005,
#33006,#33007,#33008,#33009,#33010,#33011,#33012,#33013,#33014,#33015,#33016,
#33017,#33018,#33019,#33020,#33021,#33022,#33023,#33024,#33025,#33026,#33027,
#33028,#33029,#33030,#33031,#33032,#33033,#33034,#33035,#33036,#33037,#33038,
#33039,#33040,#33041,#33042,#33043,#33044,#33045,#33046,#33047,#33048,#33049,
#33050,#33051,#33052,#33053,#33054,#33055,#33056,#33057,#33058,#33059,#33060,
#33061,#33062,#33063,#33064,#33065,#33066,#33067,#33068,#33069,#33070,#33071,
#33072,#33073,#33074,#33075,#33076,#33077,#33078,#33079,#33080,#33081,#33082,
#33083,#33084,#33085,#33086,#33087,#33088,#33089,#33090,#33091),
 .UNSPECIFIED.,.F.,.F.,(4,3,3,3,3,3,3,3,3,3,3,3,3,3,3,3,3,3,3,3,3,3,3,3,
3,3,3,3,3,3,4),(0.,0.0323971454667795,0.0650536488164166,0.0985250267045374,
0.129588581867118,0.13467228593443,0.168838432673145,0.203443204976229,
0.238107726142545,0.26707589046058,0.272862060653106,0.277501012548678,
0.313123984749285,0.348617864081868,0.35417215967219,0.388993021314974,
0.410899893444863,0.417113525277951,0.422029119319603,0.457837540262106,
0.49387383576635,0.530488931026721,0.565262803089615,0.571306516388801,
0.608618623127816,0.645997594535657,0.655870746107889,0.662594569309399,
0.701717300056918,0.740840030804437,0.757688813005636),.UNSPECIFIED.);
#1523=B_SPLINE_CURVE_WITH_KNOTS('',3,(#33336,#33337,#33338,#33339,#33340,
#33341,#33342,#33343,#33344,#33345,#33346,#33347,#33348,#33349,#33350,#33351,
#33352,#33353,#33354,#33355,#33356,#33357,#33358,#33359,#33360,#33361,#33362,
#33363,#33364,#33365,#33366,#33367,#33368,#33369,#33370,#33371,#33372,#33373,
#33374,#33375,#33376,#33377,#33378,#33379,#33380,#33381,#33382,#33383,#33384,
#33385,#33386,#33387,#33388,#33389,#33390,#33391,#33392,#33393,#33394,#33395,
#33396,#33397,#33398,#33399,#33400,#33401,#33402,#33403,#33404,#33405,#33406,
#33407,#33408,#33409,#33410,#33411,#33412,#33413,#33414,#33415,#33416,#33417,
#33418,#33419,#33420,#33421,#33422,#33423,#33424,#33425,#33426,#33427,#33428,
#33429),.UNSPECIFIED.,.F.,.F.,(4,3,3,3,3,3,3,3,3,3,3,3,3,3,3,3,3,3,3,3,
3,3,3,3,3,3,3,3,3,3,3,4),(0.,0.0323971106182625,0.0650535600024233,0.0985249065560379,
0.12958844247305,0.134672211515514,0.168838316865248,0.20344306680887,0.23810760081696,
0.267075785377979,0.272860859709737,0.277498564566242,0.313121517298547,
0.348615432551105,0.354172159672169,0.388993050154282,0.41089992209137,
0.417113614967599,0.422029263005729,0.457357723104148,0.493337814845609,
0.529931916187903,0.556146362990719,0.565213636980827,0.571306505714019,
0.608618620517587,0.645997591303791,0.6558707597048,0.662594586404321,0.70171730860435,
0.74084003080438,0.757688816127246),.UNSPECIFIED.);
#1524=B_SPLINE_CURVE_WITH_KNOTS('',3,(#33430,#33431,#33432,#33433,#33434,
#33435,#33436,#33437,#33438,#33439,#33440,#33441,#33442,#33443,#33444,#33445,
#33446,#33447,#33448,#33449,#33450,#33451,#33452,#33453,#33454,#33455,#33456,
#33457,#33458,#33459,#33460,#33461,#33462,#33463,#33464,#33465,#33466,#33467,
#33468,#33469,#33470,#33471,#33472,#33473,#33474,#33475,#33476,#33477,#33478,
#33479,#33480,#33481,#33482,#33483,#33484,#33485,#33486,#33487,#33488,#33489,
#33490,#33491,#33492,#33493,#33494,#33495,#33496,#33497,#33498,#33499,#33500,
#33501,#33502,#33503,#33504,#33505,#33506,#33507,#33508,#33509,#33510,#33511,
#33512,#33513,#33514,#33515,#33516,#33517,#33518,#33519,#33520,#33521,#33522,
#33523),.UNSPECIFIED.,.F.,.F.,(4,3,3,3,3,3,3,3,3,3,3,3,3,3,3,3,3,3,3,3,
3,3,3,3,3,3,3,3,3,3,3,4),(3.15881253341124E-15,0.037509298934911,0.0752806849453368,
0.113182237345987,0.136543756612647,0.150023018727175,0.156484526466218,
0.162775149619923,0.199734977082873,0.236494912447612,0.272408734754427,
0.300074391479266,0.306205590700807,0.311264773878789,0.346804545360892,
0.381619091867029,0.38992798633622,0.425957306860802,0.454093087159789,
0.459010598705686,0.494000696219774,0.529122663331113,0.563682436557196,
0.594976556680381,0.600634899827219,0.634691065010384,0.662654256798317,
0.675839591841063,0.684660531999309,0.717119975802094,0.746543832162118,
0.760759816994502),.UNSPECIFIED.);
#1525=B_SPLINE_CURVE_WITH_KNOTS('',3,(#33535,#33536,#33537,#33538,#33539,
#33540,#33541,#33542),.UNSPECIFIED.,.F.,.F.,(4,2,2,4),(-1.55140558439687,
-1.49530246566204,-1.28032845030884,-1.06535443495564),.UNSPECIFIED.);
#1526=B_SPLINE_CURVE_WITH_KNOTS('',3,(#33544,#33545,#33546,#33547,#33548,
#33549,#33550,#33551,#33552,#33553),.UNSPECIFIED.,.F.,.F.,(4,2,2,2,4),(0.479243585826225,
0.566096001425061,0.754791726540168,0.943487451655276,1.03033986725411),
 .UNSPECIFIED.);
#1527=B_SPLINE_CURVE_WITH_KNOTS('',3,(#33555,#33556,#33557,#33558,#33559,
#33560,#33561,#33562,#33563,#33564,#33565,#33566,#33567,#33568),
 .UNSPECIFIED.,.F.,.F.,(4,2,2,2,2,2,4),(-1.55140558439687,-1.49530246566204,
-1.28032845030884,-1.06535443495564,-0.850380419602444,-0.635406404249244,
-0.579303285514419),.UNSPECIFIED.);
#1528=B_SPLINE_CURVE_WITH_KNOTS('',3,(#33570,#33571,#33572,#33573,#33574,
#33575,#33576,#33577,#33578,#33579),.UNSPECIFIED.,.F.,.F.,(4,2,2,2,4),(1.98882703890656,
2.0756794545054,2.26437517962051,2.45307090473561,2.53992332033445),
 .UNSPECIFIED.);
#1529=B_SPLINE_CURVE_WITH_KNOTS('',3,(#33580,#33581,#33582,#33583,#33584,
#33585,#33586,#33587),.UNSPECIFIED.,.F.,.F.,(4,2,2,4),(-1.06535443495564,
-0.850380419602443,-0.635406404249243,-0.57930328551442),.UNSPECIFIED.);
#1530=B_SPLINE_CURVE_WITH_KNOTS('',3,(#33590,#33591,#33592,#33593,#33594,
#33595,#33596,#33597,#33598,#33599,#33600,#33601,#33602,#33603,#33604,#33605,
#33606,#33607),.UNSPECIFIED.,.F.,.F.,(4,2,2,2,2,2,2,2,4),(-2.26535091124315,
-2.07657500399737,-1.88779909675158,-1.69901651879018,-1.51023394082877,
-1.32145136286736,-1.13266878490596,-0.94389287766017,-0.755116970414384),
 .UNSPECIFIED.);
#1531=B_SPLINE_CURVE_WITH_KNOTS('',3,(#33609,#33610,#33611,#33612,#33613,
#33614,#33615,#33616,#33617,#33618,#33619,#33620,#33621,#33622,#33623,#33624,
#33625,#33626,#33627),.UNSPECIFIED.,.F.,.F.,(4,2,2,2,3,2,2,2,4),(2.26535091124315,
2.45412681848894,2.64290272573473,2.83168530369613,3.02046788165754,3.20925045961894,
3.39803303758035,3.58680894482614,3.77558485207192),.UNSPECIFIED.);
#1532=B_SPLINE_CURVE_WITH_KNOTS('',3,(#33630,#33631,#33632,#33633,#33634,
#33635,#33636,#33637,#33638,#33639,#33640,#33641,#33642,#33643,#33644,#33645,
#33646,#33647,#33648,#33649,#33650,#33651,#33652,#33653,#33654,#33655,#33656,
#33657,#33658,#33659,#33660,#33661,#33662,#33663),.UNSPECIFIED.,.T.,.F.,
(4,2,2,2,2,2,2,2,2,2,2,2,2,2,2,2,4),(-3.02046788165754,-2.83168530369613,
-2.64290272573473,-2.45412681848894,-2.26535091124315,-2.07657500399737,
-1.88779909675158,-1.69901651879018,-1.51023394082877,-1.32145136286736,
-1.13266878490596,-0.943892877660171,-0.755116970414385,-0.566341063168599,
-0.377565155922813,-0.188782577961406,0.),.UNSPECIFIED.);
#1533=B_SPLINE_CURVE_WITH_KNOTS('',3,(#33667,#33668,#33669,#33670,#33671,
#33672,#33673,#33674),.UNSPECIFIED.,.F.,.F.,(4,2,2,4),(-1.55140558439687,
-1.49530246566204,-1.28032845030884,-1.06535443495564),.UNSPECIFIED.);
#1534=B_SPLINE_CURVE_WITH_KNOTS('',3,(#33676,#33677,#33678,#33679,#33680,
#33681,#33682,#33683,#33684,#33685),.UNSPECIFIED.,.F.,.F.,(4,2,2,2,4),(1.98882703890656,
2.0756794545054,2.26437517962051,2.45307090473561,2.53992332033445),
 .UNSPECIFIED.);
#1535=B_SPLINE_CURVE_WITH_KNOTS('',3,(#33687,#33688,#33689,#33690,#33691,
#33692,#33693,#33694,#33695,#33696,#33697,#33698,#33699,#33700),
 .UNSPECIFIED.,.F.,.F.,(4,2,2,2,2,2,4),(-1.55140558439687,-1.49530246566204,
-1.28032845030884,-1.06535443495564,-0.850380419602444,-0.635406404249244,
-0.57930328551442),.UNSPECIFIED.);
#1536=B_SPLINE_CURVE_WITH_KNOTS('',3,(#33702,#33703,#33704,#33705,#33706,
#33707,#33708,#33709,#33710,#33711),.UNSPECIFIED.,.F.,.F.,(4,2,2,2,4),(0.479243585826223,
0.566096001425061,0.754791726540169,0.943487451655276,1.03033986725411),
 .UNSPECIFIED.);
#1537=B_SPLINE_CURVE_WITH_KNOTS('',3,(#33712,#33713,#33714,#33715,#33716,
#33717,#33718,#33719),.UNSPECIFIED.,.F.,.F.,(4,2,2,4),(-1.06535443495564,
-0.850380419602443,-0.635406404249243,-0.57930328551442),.UNSPECIFIED.);
#1757=VERTEX_POINT('',#26044);
#1758=VERTEX_POINT('',#26045);
#1759=VERTEX_POINT('',#26047);
#1760=VERTEX_POINT('',#26052);
#1761=VERTEX_POINT('',#26110);
#1762=VERTEX_POINT('',#26111);
#1763=VERTEX_POINT('',#26113);
#1764=VERTEX_POINT('',#26269);
#1765=VERTEX_POINT('',#26501);
#1766=VERTEX_POINT('',#26502);
#1767=VERTEX_POINT('',#26504);
#1768=VERTEX_POINT('',#26735);
#1769=VERTEX_POINT('',#26967);
#1770=VERTEX_POINT('',#26968);
#1771=VERTEX_POINT('',#26970);
#1772=VERTEX_POINT('',#27204);
#1773=VERTEX_POINT('',#27433);
#1774=VERTEX_POINT('',#27434);
#1775=VERTEX_POINT('',#27436);
#1776=VERTEX_POINT('',#27524);
#1777=VERTEX_POINT('',#27753);
#1778=VERTEX_POINT('',#27754);
#1779=VERTEX_POINT('',#27756);
#1780=VERTEX_POINT('',#27911);
#1781=VERTEX_POINT('',#28143);
#1782=VERTEX_POINT('',#28144);
#1783=VERTEX_POINT('',#28146);
#1784=VERTEX_POINT('',#28380);
#1785=VERTEX_POINT('',#28609);
#1786=VERTEX_POINT('',#28610);
#1787=VERTEX_POINT('',#28612);
#1788=VERTEX_POINT('',#28840);
#1789=VERTEX_POINT('',#29075);
#1790=VERTEX_POINT('',#29076);
#1791=VERTEX_POINT('',#29078);
#1792=VERTEX_POINT('',#29161);
#1793=VERTEX_POINT('',#29167);
#1794=VERTEX_POINT('',#29169);
#1795=VERTEX_POINT('',#29320);
#1796=VERTEX_POINT('',#29321);
#1797=VERTEX_POINT('',#29323);
#1798=VERTEX_POINT('',#29364);
#1799=VERTEX_POINT('',#29375);
#1800=VERTEX_POINT('',#29720);
#1801=VERTEX_POINT('',#30073);
#1802=VERTEX_POINT('',#30422);
#1803=VERTEX_POINT('',#30634);
#1804=VERTEX_POINT('',#30765);
#1805=VERTEX_POINT('',#30767);
#1806=VERTEX_POINT('',#30958);
#1807=VERTEX_POINT('',#30970);
#1808=VERTEX_POINT('',#31313);
#1809=VERTEX_POINT('',#31662);
#1810=VERTEX_POINT('',#32201);
#1811=VERTEX_POINT('',#32432);
#1812=VERTEX_POINT('',#33525);
#1813=VERTEX_POINT('',#33526);
#1814=VERTEX_POINT('',#33530);
#1815=VERTEX_POINT('',#33532);
#1816=VERTEX_POINT('',#33534);
#1817=VERTEX_POINT('',#33543);
#1818=VERTEX_POINT('',#33554);
#1819=VERTEX_POINT('',#33569);
#1820=VERTEX_POINT('',#33629);
#1821=VERTEX_POINT('',#33664);
#1822=VERTEX_POINT('',#33666);
#1823=VERTEX_POINT('',#33675);
#1824=VERTEX_POINT('',#33686);
#1825=VERTEX_POINT('',#33701);
#1826=VERTEX_POINT('',#33721);
#1827=VERTEX_POINT('',#33723);
#1828=VERTEX_POINT('',#33725);
#1829=VERTEX_POINT('',#33727);
#1830=VERTEX_POINT('',#33731);
#1831=VERTEX_POINT('',#33735);
#1832=VERTEX_POINT('',#33737);
#1833=VERTEX_POINT('',#33739);
#1834=VERTEX_POINT('',#33741);
#1835=VERTEX_POINT('',#33745);
#1836=VERTEX_POINT('',#33749);
#1837=VERTEX_POINT('',#33751);
#1838=VERTEX_POINT('',#33755);
#1839=VERTEX_POINT('',#33756);
#1840=VERTEX_POINT('',#33761);
#1841=VERTEX_POINT('',#33762);
#1842=VERTEX_POINT('',#33767);
#1843=VERTEX_POINT('',#33768);
#1844=VERTEX_POINT('',#33773);
#1845=VERTEX_POINT('',#33774);
#1846=VERTEX_POINT('',#33779);
#1847=VERTEX_POINT('',#33780);
#1848=VERTEX_POINT('',#33785);
#1849=VERTEX_POINT('',#33786);
#1850=VERTEX_POINT('',#33791);
#1851=VERTEX_POINT('',#33792);
#1852=VERTEX_POINT('',#33797);
#1853=VERTEX_POINT('',#33798);
#1854=VERTEX_POINT('',#33803);
#1855=VERTEX_POINT('',#33804);
#1856=VERTEX_POINT('',#33809);
#1857=VERTEX_POINT('',#33810);
#1858=VERTEX_POINT('',#33815);
#1859=VERTEX_POINT('',#33816);
#1860=VERTEX_POINT('',#33821);
#1861=VERTEX_POINT('',#33822);
#1862=VERTEX_POINT('',#33827);
#1863=VERTEX_POINT('',#33832);
#1864=VERTEX_POINT('',#33836);
#1865=VERTEX_POINT('',#33837);
#1866=VERTEX_POINT('',#33842);
#1867=VERTEX_POINT('',#33843);
#1868=VERTEX_POINT('',#33848);
#1869=VERTEX_POINT('',#33849);
#1870=VERTEX_POINT('',#33854);
#1871=VERTEX_POINT('',#33855);
#1872=VERTEX_POINT('',#33860);
#1873=VERTEX_POINT('',#33861);
#1874=VERTEX_POINT('',#33866);
#1875=VERTEX_POINT('',#33867);
#1876=VERTEX_POINT('',#33872);
#1877=VERTEX_POINT('',#33873);
#1878=VERTEX_POINT('',#33878);
#1879=VERTEX_POINT('',#33879);
#1880=VERTEX_POINT('',#33884);
#1881=VERTEX_POINT('',#33885);
#1882=VERTEX_POINT('',#33890);
#1883=VERTEX_POINT('',#33891);
#1884=VERTEX_POINT('',#33896);
#1885=VERTEX_POINT('',#33897);
#1886=VERTEX_POINT('',#33902);
#1887=VERTEX_POINT('',#33903);
#1888=VERTEX_POINT('',#33908);
#1889=VERTEX_POINT('',#33909);
#1890=VERTEX_POINT('',#33914);
#1891=VERTEX_POINT('',#33915);
#1892=VERTEX_POINT('',#33920);
#1893=VERTEX_POINT('',#33921);
#1894=VERTEX_POINT('',#33926);
#1895=VERTEX_POINT('',#33933);
#1896=VERTEX_POINT('',#33935);
#1897=VERTEX_POINT('',#33939);
#1898=VERTEX_POINT('',#33943);
#1899=VERTEX_POINT('',#33947);
#1900=VERTEX_POINT('',#33951);
#1901=VERTEX_POINT('',#33955);
#1902=VERTEX_POINT('',#33959);
#1903=VERTEX_POINT('',#33963);
#1904=VERTEX_POINT('',#33967);
#1905=VERTEX_POINT('',#33971);
#1906=VERTEX_POINT('',#33975);
#1907=VERTEX_POINT('',#33979);
#1908=VERTEX_POINT('',#33983);
#1909=VERTEX_POINT('',#33987);
#1910=VERTEX_POINT('',#33993);
#1911=VERTEX_POINT('',#33995);
#1912=VERTEX_POINT('',#33997);
#1913=VERTEX_POINT('',#33999);
#1914=VERTEX_POINT('',#34001);
#1915=VERTEX_POINT('',#34003);
#1916=VERTEX_POINT('',#34005);
#1917=VERTEX_POINT('',#34007);
#1918=VERTEX_POINT('',#34009);
#1919=VERTEX_POINT('',#34012);
#1920=VERTEX_POINT('',#34013);
#1921=VERTEX_POINT('',#34015);
#1922=VERTEX_POINT('',#34017);
#1923=VERTEX_POINT('',#34021);
#1924=VERTEX_POINT('',#34026);
#1925=VERTEX_POINT('',#34030);
#1926=VERTEX_POINT('',#34034);
#1927=VERTEX_POINT('',#34038);
#1928=VERTEX_POINT('',#34042);
#1929=VERTEX_POINT('',#34046);
#1930=VERTEX_POINT('',#34050);
#1931=VERTEX_POINT('',#34054);
#1932=VERTEX_POINT('',#34058);
#1933=VERTEX_POINT('',#34062);
#1934=VERTEX_POINT('',#34066);
#1935=VERTEX_POINT('',#34070);
#1936=VERTEX_POINT('',#34074);
#1937=VERTEX_POINT('',#34078);
#1938=VERTEX_POINT('',#34082);
#1939=VERTEX_POINT('',#34086);
#1940=VERTEX_POINT('',#34090);
#1941=VERTEX_POINT('',#34095);
#1942=VERTEX_POINT('',#34099);
#1943=VERTEX_POINT('',#34103);
#1944=VERTEX_POINT('',#34104);
#1945=VERTEX_POINT('',#34109);
#1946=VERTEX_POINT('',#34110);
#1947=VERTEX_POINT('',#34115);
#1948=VERTEX_POINT('',#34116);
#1949=VERTEX_POINT('',#34121);
#1950=VERTEX_POINT('',#34122);
#1951=VERTEX_POINT('',#34127);
#1952=VERTEX_POINT('',#34128);
#1953=VERTEX_POINT('',#34133);
#1954=VERTEX_POINT('',#34134);
#1955=VERTEX_POINT('',#34139);
#1956=VERTEX_POINT('',#34140);
#1957=VERTEX_POINT('',#34145);
#1958=VERTEX_POINT('',#34146);
#1959=VERTEX_POINT('',#34151);
#1960=VERTEX_POINT('',#34152);
#1961=VERTEX_POINT('',#34157);
#1962=VERTEX_POINT('',#34158);
#1963=VERTEX_POINT('',#34193);
#1964=VERTEX_POINT('',#34195);
#1965=VERTEX_POINT('',#34197);
#1966=VERTEX_POINT('',#34199);
#1967=VERTEX_POINT('',#34201);
#1968=VERTEX_POINT('',#34203);
#1969=VERTEX_POINT('',#34205);
#1970=VERTEX_POINT('',#34207);
#1971=VERTEX_POINT('',#34209);
#1972=VERTEX_POINT('',#34212);
#1973=VERTEX_POINT('',#34214);
#1974=VERTEX_POINT('',#34218);
#1975=VERTEX_POINT('',#34220);
#2289=EDGE_CURVE('',#1757,#1758,#1068,.T.);
#2290=EDGE_CURVE('',#1758,#1759,#1470,.T.);
#2291=EDGE_CURVE('',#1760,#1759,#207,.T.);
#2292=EDGE_CURVE('',#1757,#1760,#1471,.T.);
#2293=EDGE_CURVE('',#1761,#1762,#1069,.T.);
#2294=EDGE_CURVE('',#1762,#1763,#1472,.T.);
#2295=EDGE_CURVE('',#1763,#1758,#1473,.T.);
#2296=EDGE_CURVE('',#1764,#1757,#1474,.T.);
#2297=EDGE_CURVE('',#1761,#1764,#1475,.T.);
#2298=EDGE_CURVE('',#1765,#1766,#1070,.T.);
#2299=EDGE_CURVE('',#1766,#1767,#1476,.T.);
#2300=EDGE_CURVE('',#1767,#1762,#1477,.T.);
#2301=EDGE_CURVE('',#1768,#1761,#1478,.T.);
#2302=EDGE_CURVE('',#1765,#1768,#1479,.T.);
#2303=EDGE_CURVE('',#1769,#1770,#1071,.T.);
#2304=EDGE_CURVE('',#1770,#1771,#1480,.T.);
#2305=EDGE_CURVE('',#1771,#1766,#1481,.T.);
#2306=EDGE_CURVE('',#1772,#1765,#1482,.T.);
#2307=EDGE_CURVE('',#1769,#1772,#1483,.T.);
#2308=EDGE_CURVE('',#1773,#1774,#1072,.T.);
#2309=EDGE_CURVE('',#1774,#1775,#1484,.T.);
#2310=EDGE_CURVE('',#1775,#1770,#1485,.T.);
#2311=EDGE_CURVE('',#1776,#1769,#1486,.T.);
#2312=EDGE_CURVE('',#1773,#1776,#1487,.T.);
#2313=EDGE_CURVE('',#1777,#1778,#1073,.T.);
#2314=EDGE_CURVE('',#1778,#1779,#1488,.T.);
#2315=EDGE_CURVE('',#1779,#1774,#1489,.T.);
#2316=EDGE_CURVE('',#1780,#1773,#1490,.T.);
#2317=EDGE_CURVE('',#1777,#1780,#1491,.T.);
#2318=EDGE_CURVE('',#1781,#1782,#1074,.T.);
#2319=EDGE_CURVE('',#1782,#1783,#1492,.T.);
#2320=EDGE_CURVE('',#1783,#1778,#1493,.T.);
#2321=EDGE_CURVE('',#1784,#1777,#1494,.T.);
#2322=EDGE_CURVE('',#1781,#1784,#1495,.T.);
#2323=EDGE_CURVE('',#1785,#1786,#1075,.T.);
#2324=EDGE_CURVE('',#1786,#1787,#1496,.T.);
#2325=EDGE_CURVE('',#1787,#1782,#1497,.T.);
#2326=EDGE_CURVE('',#1788,#1781,#1498,.T.);
#2327=EDGE_CURVE('',#1785,#1788,#1499,.T.);
#2328=EDGE_CURVE('',#1789,#1790,#1076,.T.);
#2329=EDGE_CURVE('',#1791,#1789,#1500,.T.);
#2330=EDGE_CURVE('',#1792,#1791,#1501,.T.);
#2331=EDGE_CURVE('',#1793,#1792,#208,.T.);
#2332=EDGE_CURVE('',#1793,#1794,#1502,.T.);
#2333=EDGE_CURVE('',#1794,#1790,#1503,.T.);
#2334=EDGE_CURVE('',#1795,#1796,#209,.T.);
#2335=EDGE_CURVE('',#1795,#1797,#1504,.T.);
#2336=EDGE_CURVE('',#1797,#1798,#1505,.T.);
#2337=EDGE_CURVE('',#1798,#1799,#1506,.T.);
#2338=EDGE_CURVE('',#1799,#1800,#1507,.T.);
#2339=EDGE_CURVE('',#1800,#1801,#1508,.T.);
#2340=EDGE_CURVE('',#1801,#1802,#1509,.T.);
#2341=EDGE_CURVE('',#1802,#1803,#1510,.T.);
#2342=EDGE_CURVE('',#1803,#1804,#210,.T.);
#2343=EDGE_CURVE('',#1804,#1805,#1511,.T.);
#2344=EDGE_CURVE('',#1805,#1806,#1512,.T.);
#2345=EDGE_CURVE('',#1806,#1807,#1513,.T.);
#2346=EDGE_CURVE('',#1807,#1808,#1514,.T.);
#2347=EDGE_CURVE('',#1808,#1809,#1515,.T.);
#2348=EDGE_CURVE('',#1809,#1796,#1516,.T.);
#2349=EDGE_CURVE('',#1790,#1810,#1517,.T.);
#2350=EDGE_CURVE('',#1810,#1786,#1518,.T.);
#2351=EDGE_CURVE('',#1811,#1785,#1519,.T.);
#2352=EDGE_CURVE('',#1789,#1811,#1520,.T.);
#2353=EDGE_CURVE('',#1759,#1795,#1521,.T.);
#2354=EDGE_CURVE('',#1803,#1793,#1522,.T.);
#2355=EDGE_CURVE('',#1796,#1760,#1523,.T.);
#2356=EDGE_CURVE('',#1792,#1804,#1524,.T.);
#2357=EDGE_CURVE('',#1812,#1813,#211,.T.);
#2358=EDGE_CURVE('',#1813,#1812,#212,.T.);
#2359=EDGE_CURVE('',#1814,#1814,#213,.T.);
#2360=EDGE_CURVE('',#1814,#1815,#1077,.T.);
#2361=EDGE_CURVE('',#1816,#1815,#1525,.T.);
#2362=EDGE_CURVE('',#1817,#1816,#1526,.T.);
#2363=EDGE_CURVE('',#1818,#1817,#1527,.T.);
#2364=EDGE_CURVE('',#1819,#1818,#1528,.T.);
#2365=EDGE_CURVE('',#1815,#1819,#1529,.T.);
#2366=EDGE_CURVE('',#1813,#1812,#1530,.T.);
#2367=EDGE_CURVE('',#1812,#1813,#1531,.F.);
#2368=EDGE_CURVE('',#1820,#1820,#1532,.T.);
#2369=EDGE_CURVE('',#1820,#1821,#1078,.T.);
#2370=EDGE_CURVE('',#1822,#1821,#1533,.T.);
#2371=EDGE_CURVE('',#1823,#1822,#1534,.T.);
#2372=EDGE_CURVE('',#1824,#1823,#1535,.T.);
#2373=EDGE_CURVE('',#1825,#1824,#1536,.T.);
#2374=EDGE_CURVE('',#1821,#1825,#1537,.T.);
#2375=EDGE_CURVE('',#1825,#1826,#1079,.T.);
#2376=EDGE_CURVE('',#1827,#1826,#214,.T.);
#2377=EDGE_CURVE('',#1827,#1828,#1080,.T.);
#2378=EDGE_CURVE('',#1829,#1828,#215,.T.);
#2379=EDGE_CURVE('',#1829,#1822,#1081,.T.);
#2380=EDGE_CURVE('',#1830,#1824,#1082,.T.);
#2381=EDGE_CURVE('',#1826,#1830,#216,.T.);
#2382=EDGE_CURVE('',#1819,#1831,#1083,.T.);
#2383=EDGE_CURVE('',#1832,#1831,#217,.T.);
#2384=EDGE_CURVE('',#1832,#1833,#1084,.T.);
#2385=EDGE_CURVE('',#1834,#1833,#218,.T.);
#2386=EDGE_CURVE('',#1834,#1816,#1085,.T.);
#2387=EDGE_CURVE('',#1835,#1818,#1086,.T.);
#2388=EDGE_CURVE('',#1831,#1835,#219,.T.);
#2389=EDGE_CURVE('',#1826,#1836,#220,.T.);
#2390=EDGE_CURVE('',#1836,#1837,#221,.T.);
#2391=EDGE_CURVE('',#1837,#1827,#222,.T.);
#2392=EDGE_CURVE('',#1838,#1839,#223,.T.);
#2393=EDGE_CURVE('',#1839,#1827,#224,.T.);
#2394=EDGE_CURVE('',#1837,#1838,#225,.T.);
#2395=EDGE_CURVE('',#1840,#1841,#226,.T.);
#2396=EDGE_CURVE('',#1841,#1839,#227,.T.);
#2397=EDGE_CURVE('',#1838,#1840,#228,.T.);
#2398=EDGE_CURVE('',#1842,#1843,#229,.T.);
#2399=EDGE_CURVE('',#1843,#1841,#230,.T.);
#2400=EDGE_CURVE('',#1840,#1842,#231,.T.);
#2401=EDGE_CURVE('',#1844,#1845,#232,.T.);
#2402=EDGE_CURVE('',#1845,#1843,#233,.T.);
#2403=EDGE_CURVE('',#1842,#1844,#234,.T.);
#2404=EDGE_CURVE('',#1846,#1847,#235,.T.);
#2405=EDGE_CURVE('',#1847,#1845,#236,.T.);
#2406=EDGE_CURVE('',#1844,#1846,#237,.T.);
#2407=EDGE_CURVE('',#1848,#1849,#238,.T.);
#2408=EDGE_CURVE('',#1849,#1847,#239,.T.);
#2409=EDGE_CURVE('',#1846,#1848,#240,.T.);
#2410=EDGE_CURVE('',#1850,#1851,#241,.T.);
#2411=EDGE_CURVE('',#1851,#1849,#242,.T.);
#2412=EDGE_CURVE('',#1848,#1850,#243,.T.);
#2413=EDGE_CURVE('',#1852,#1853,#244,.T.);
#2414=EDGE_CURVE('',#1853,#1851,#245,.T.);
#2415=EDGE_CURVE('',#1850,#1852,#246,.T.);
#2416=EDGE_CURVE('',#1854,#1855,#247,.T.);
#2417=EDGE_CURVE('',#1855,#1853,#248,.T.);
#2418=EDGE_CURVE('',#1852,#1854,#249,.T.);
#2419=EDGE_CURVE('',#1856,#1857,#250,.T.);
#2420=EDGE_CURVE('',#1857,#1855,#251,.T.);
#2421=EDGE_CURVE('',#1854,#1856,#252,.T.);
#2422=EDGE_CURVE('',#1858,#1859,#253,.T.);
#2423=EDGE_CURVE('',#1859,#1857,#254,.T.);
#2424=EDGE_CURVE('',#1856,#1858,#255,.T.);
#2425=EDGE_CURVE('',#1860,#1861,#256,.T.);
#2426=EDGE_CURVE('',#1861,#1859,#257,.T.);
#2427=EDGE_CURVE('',#1858,#1860,#258,.T.);
#2428=EDGE_CURVE('',#1862,#1833,#259,.T.);
#2429=EDGE_CURVE('',#1833,#1861,#260,.T.);
#2430=EDGE_CURVE('',#1860,#1862,#261,.T.);
#2431=EDGE_CURVE('',#1863,#1834,#262,.T.);
#2432=EDGE_CURVE('',#1862,#1863,#263,.T.);
#2433=EDGE_CURVE('',#1864,#1865,#264,.T.);
#2434=EDGE_CURVE('',#1865,#1834,#265,.T.);
#2435=EDGE_CURVE('',#1863,#1864,#266,.T.);
#2436=EDGE_CURVE('',#1866,#1867,#267,.T.);
#2437=EDGE_CURVE('',#1867,#1865,#268,.T.);
#2438=EDGE_CURVE('',#1864,#1866,#269,.T.);
#2439=EDGE_CURVE('',#1868,#1869,#270,.T.);
#2440=EDGE_CURVE('',#1869,#1867,#271,.T.);
#2441=EDGE_CURVE('',#1866,#1868,#272,.T.);
#2442=EDGE_CURVE('',#1870,#1871,#273,.T.);
#2443=EDGE_CURVE('',#1871,#1869,#274,.T.);
#2444=EDGE_CURVE('',#1868,#1870,#275,.T.);
#2445=EDGE_CURVE('',#1872,#1873,#276,.T.);
#2446=EDGE_CURVE('',#1873,#1871,#277,.T.);
#2447=EDGE_CURVE('',#1870,#1872,#278,.T.);
#2448=EDGE_CURVE('',#1874,#1875,#279,.T.);
#2449=EDGE_CURVE('',#1875,#1873,#280,.T.);
#2450=EDGE_CURVE('',#1872,#1874,#281,.T.);
#2451=EDGE_CURVE('',#1876,#1877,#282,.T.);
#2452=EDGE_CURVE('',#1877,#1875,#283,.T.);
#2453=EDGE_CURVE('',#1874,#1876,#284,.T.);
#2454=EDGE_CURVE('',#1878,#1879,#285,.T.);
#2455=EDGE_CURVE('',#1879,#1877,#286,.T.);
#2456=EDGE_CURVE('',#1876,#1878,#287,.T.);
#2457=EDGE_CURVE('',#1880,#1881,#288,.T.);
#2458=EDGE_CURVE('',#1881,#1879,#289,.T.);
#2459=EDGE_CURVE('',#1878,#1880,#290,.T.);
#2460=EDGE_CURVE('',#1882,#1883,#291,.T.);
#2461=EDGE_CURVE('',#1883,#1881,#292,.T.);
#2462=EDGE_CURVE('',#1880,#1882,#293,.T.);
#2463=EDGE_CURVE('',#1884,#1885,#294,.T.);
#2464=EDGE_CURVE('',#1885,#1883,#295,.T.);
#2465=EDGE_CURVE('',#1882,#1884,#296,.T.);
#2466=EDGE_CURVE('',#1886,#1887,#297,.T.);
#2467=EDGE_CURVE('',#1887,#1885,#298,.T.);
#2468=EDGE_CURVE('',#1884,#1886,#299,.T.);
#2469=EDGE_CURVE('',#1888,#1889,#300,.T.);
#2470=EDGE_CURVE('',#1889,#1887,#301,.T.);
#2471=EDGE_CURVE('',#1886,#1888,#302,.T.);
#2472=EDGE_CURVE('',#1890,#1891,#303,.T.);
#2473=EDGE_CURVE('',#1891,#1889,#304,.T.);
#2474=EDGE_CURVE('',#1888,#1890,#305,.T.);
#2475=EDGE_CURVE('',#1892,#1893,#306,.T.);
#2476=EDGE_CURVE('',#1893,#1891,#307,.T.);
#2477=EDGE_CURVE('',#1890,#1892,#308,.T.);
#2478=EDGE_CURVE('',#1894,#1830,#309,.T.);
#2479=EDGE_CURVE('',#1830,#1893,#310,.T.);
#2480=EDGE_CURVE('',#1892,#1894,#311,.T.);
#2481=EDGE_CURVE('',#1894,#1836,#312,.T.);
#2482=EDGE_CURVE('',#1895,#1869,#1087,.T.);
#2483=EDGE_CURVE('',#1896,#1895,#313,.T.);
#2484=EDGE_CURVE('',#1867,#1896,#1088,.T.);
#2485=EDGE_CURVE('',#1871,#1897,#1089,.T.);
#2486=EDGE_CURVE('',#1895,#1897,#314,.T.);
#2487=EDGE_CURVE('',#1898,#1873,#1090,.T.);
#2488=EDGE_CURVE('',#1897,#1898,#315,.T.);
#2489=EDGE_CURVE('',#1875,#1899,#1091,.T.);
#2490=EDGE_CURVE('',#1898,#1899,#316,.T.);
#2491=EDGE_CURVE('',#1900,#1877,#1092,.T.);
#2492=EDGE_CURVE('',#1899,#1900,#317,.T.);
#2493=EDGE_CURVE('',#1879,#1901,#1093,.T.);
#2494=EDGE_CURVE('',#1900,#1901,#318,.T.);
#2495=EDGE_CURVE('',#1902,#1881,#1094,.T.);
#2496=EDGE_CURVE('',#1901,#1902,#319,.T.);
#2497=EDGE_CURVE('',#1883,#1903,#1095,.T.);
#2498=EDGE_CURVE('',#1902,#1903,#320,.T.);
#2499=EDGE_CURVE('',#1904,#1885,#1096,.T.);
#2500=EDGE_CURVE('',#1903,#1904,#321,.T.);
#2501=EDGE_CURVE('',#1887,#1905,#1097,.T.);
#2502=EDGE_CURVE('',#1904,#1905,#322,.T.);
#2503=EDGE_CURVE('',#1906,#1889,#1098,.T.);
#2504=EDGE_CURVE('',#1905,#1906,#323,.T.);
#2505=EDGE_CURVE('',#1891,#1907,#1099,.T.);
#2506=EDGE_CURVE('',#1906,#1907,#324,.T.);
#2507=EDGE_CURVE('',#1908,#1893,#1100,.T.);
#2508=EDGE_CURVE('',#1907,#1908,#325,.T.);
#2509=EDGE_CURVE('',#1823,#1909,#1101,.T.);
#2510=EDGE_CURVE('',#1908,#1909,#326,.T.);
#2511=EDGE_CURVE('',#1909,#1829,#327,.T.);
#2512=EDGE_CURVE('',#1910,#1910,#328,.T.);
#2513=EDGE_CURVE('',#1911,#1911,#329,.T.);
#2514=EDGE_CURVE('',#1912,#1912,#330,.T.);
#2515=EDGE_CURVE('',#1913,#1913,#331,.T.);
#2516=EDGE_CURVE('',#1914,#1914,#332,.T.);
#2517=EDGE_CURVE('',#1915,#1915,#333,.T.);
#2518=EDGE_CURVE('',#1916,#1916,#334,.T.);
#2519=EDGE_CURVE('',#1917,#1917,#335,.T.);
#2520=EDGE_CURVE('',#1918,#1918,#336,.T.);
#2521=EDGE_CURVE('',#1919,#1920,#337,.T.);
#2522=EDGE_CURVE('',#1920,#1921,#338,.T.);
#2523=EDGE_CURVE('',#1921,#1922,#339,.T.);
#2524=EDGE_CURVE('',#1922,#1919,#340,.T.);
#2525=EDGE_CURVE('',#1923,#1828,#341,.T.);
#2526=EDGE_CURVE('',#1828,#1922,#342,.T.);
#2527=EDGE_CURVE('',#1921,#1923,#343,.T.);
#2528=EDGE_CURVE('',#1924,#1829,#344,.T.);
#2529=EDGE_CURVE('',#1923,#1924,#345,.T.);
#2530=EDGE_CURVE('',#1925,#1909,#346,.T.);
#2531=EDGE_CURVE('',#1924,#1925,#347,.T.);
#2532=EDGE_CURVE('',#1926,#1908,#348,.T.);
#2533=EDGE_CURVE('',#1925,#1926,#349,.T.);
#2534=EDGE_CURVE('',#1927,#1907,#350,.T.);
#2535=EDGE_CURVE('',#1926,#1927,#351,.T.);
#2536=EDGE_CURVE('',#1928,#1906,#352,.T.);
#2537=EDGE_CURVE('',#1927,#1928,#353,.T.);
#2538=EDGE_CURVE('',#1929,#1905,#354,.T.);
#2539=EDGE_CURVE('',#1928,#1929,#355,.T.);
#2540=EDGE_CURVE('',#1930,#1904,#356,.T.);
#2541=EDGE_CURVE('',#1929,#1930,#357,.T.);
#2542=EDGE_CURVE('',#1931,#1903,#358,.T.);
#2543=EDGE_CURVE('',#1930,#1931,#359,.T.);
#2544=EDGE_CURVE('',#1932,#1902,#360,.T.);
#2545=EDGE_CURVE('',#1931,#1932,#361,.T.);
#2546=EDGE_CURVE('',#1933,#1901,#362,.T.);
#2547=EDGE_CURVE('',#1932,#1933,#363,.T.);
#2548=EDGE_CURVE('',#1934,#1900,#364,.T.);
#2549=EDGE_CURVE('',#1933,#1934,#365,.T.);
#2550=EDGE_CURVE('',#1935,#1899,#366,.T.);
#2551=EDGE_CURVE('',#1934,#1935,#367,.T.);
#2552=EDGE_CURVE('',#1936,#1898,#368,.T.);
#2553=EDGE_CURVE('',#1935,#1936,#369,.T.);
#2554=EDGE_CURVE('',#1937,#1897,#370,.T.);
#2555=EDGE_CURVE('',#1936,#1937,#371,.T.);
#2556=EDGE_CURVE('',#1938,#1895,#372,.T.);
#2557=EDGE_CURVE('',#1937,#1938,#373,.T.);
#2558=EDGE_CURVE('',#1939,#1896,#374,.T.);
#2559=EDGE_CURVE('',#1938,#1939,#375,.T.);
#2560=EDGE_CURVE('',#1940,#1835,#376,.T.);
#2561=EDGE_CURVE('',#1835,#1896,#377,.T.);
#2562=EDGE_CURVE('',#1939,#1940,#378,.T.);
#2563=EDGE_CURVE('',#1941,#1831,#379,.T.);
#2564=EDGE_CURVE('',#1940,#1941,#380,.T.);
#2565=EDGE_CURVE('',#1942,#1832,#381,.T.);
#2566=EDGE_CURVE('',#1941,#1942,#382,.T.);
#2567=EDGE_CURVE('',#1943,#1944,#383,.T.);
#2568=EDGE_CURVE('',#1944,#1832,#384,.T.);
#2569=EDGE_CURVE('',#1942,#1943,#385,.T.);
#2570=EDGE_CURVE('',#1945,#1946,#386,.T.);
#2571=EDGE_CURVE('',#1946,#1944,#387,.T.);
#2572=EDGE_CURVE('',#1943,#1945,#388,.T.);
#2573=EDGE_CURVE('',#1947,#1948,#389,.T.);
#2574=EDGE_CURVE('',#1948,#1946,#390,.T.);
#2575=EDGE_CURVE('',#1945,#1947,#391,.T.);
#2576=EDGE_CURVE('',#1949,#1950,#392,.T.);
#2577=EDGE_CURVE('',#1950,#1948,#393,.T.);
#2578=EDGE_CURVE('',#1947,#1949,#394,.T.);
#2579=EDGE_CURVE('',#1951,#1952,#395,.T.);
#2580=EDGE_CURVE('',#1952,#1950,#396,.T.);
#2581=EDGE_CURVE('',#1949,#1951,#397,.T.);
#2582=EDGE_CURVE('',#1953,#1954,#398,.T.);
#2583=EDGE_CURVE('',#1954,#1952,#399,.T.);
#2584=EDGE_CURVE('',#1951,#1953,#400,.T.);
#2585=EDGE_CURVE('',#1955,#1956,#401,.T.);
#2586=EDGE_CURVE('',#1956,#1954,#402,.T.);
#2587=EDGE_CURVE('',#1953,#1955,#403,.T.);
#2588=EDGE_CURVE('',#1957,#1958,#404,.T.);
#2589=EDGE_CURVE('',#1958,#1956,#405,.T.);
#2590=EDGE_CURVE('',#1955,#1957,#406,.T.);
#2591=EDGE_CURVE('',#1959,#1960,#407,.T.);
#2592=EDGE_CURVE('',#1960,#1958,#408,.T.);
#2593=EDGE_CURVE('',#1957,#1959,#409,.T.);
#2594=EDGE_CURVE('',#1961,#1962,#410,.T.);
#2595=EDGE_CURVE('',#1962,#1960,#411,.T.);
#2596=EDGE_CURVE('',#1959,#1961,#412,.T.);
#2597=EDGE_CURVE('',#1961,#1920,#413,.T.);
#2598=EDGE_CURVE('',#1919,#1962,#414,.T.);
#2599=EDGE_CURVE('',#1817,#1865,#1102,.T.);
#2600=EDGE_CURVE('',#1861,#1944,#1103,.T.);
#2601=EDGE_CURVE('',#1946,#1859,#1104,.T.);
#2602=EDGE_CURVE('',#1857,#1948,#1105,.T.);
#2603=EDGE_CURVE('',#1950,#1855,#1106,.T.);
#2604=EDGE_CURVE('',#1853,#1952,#1107,.T.);
#2605=EDGE_CURVE('',#1954,#1851,#1108,.T.);
#2606=EDGE_CURVE('',#1849,#1956,#1109,.T.);
#2607=EDGE_CURVE('',#1958,#1847,#1110,.T.);
#2608=EDGE_CURVE('',#1845,#1960,#1111,.T.);
#2609=EDGE_CURVE('',#1962,#1843,#1112,.T.);
#2610=EDGE_CURVE('',#1841,#1919,#1113,.T.);
#2611=EDGE_CURVE('',#1922,#1839,#1114,.T.);
#2612=EDGE_CURVE('',#1963,#1963,#415,.T.);
#2613=EDGE_CURVE('',#1964,#1964,#416,.T.);
#2614=EDGE_CURVE('',#1965,#1965,#417,.T.);
#2615=EDGE_CURVE('',#1966,#1966,#418,.T.);
#2616=EDGE_CURVE('',#1967,#1967,#419,.T.);
#2617=EDGE_CURVE('',#1968,#1968,#420,.T.);
#2618=EDGE_CURVE('',#1969,#1969,#421,.T.);
#2619=EDGE_CURVE('',#1970,#1970,#422,.T.);
#2620=EDGE_CURVE('',#1971,#1971,#423,.T.);
#2621=EDGE_CURVE('',#1910,#1972,#424,.T.);
#2622=EDGE_CURVE('',#1972,#1973,#425,.T.);
#2623=EDGE_CURVE('',#1973,#1972,#426,.T.);
#2624=EDGE_CURVE('',#1973,#1974,#1115,.T.);
#2625=EDGE_CURVE('',#1975,#1974,#427,.T.);
#2626=EDGE_CURVE('',#1974,#1975,#428,.T.);
#2627=EDGE_CURVE('',#1963,#1975,#429,.T.);
#2628=EDGE_CURVE('',#1964,#1911,#1116,.T.);
#2629=EDGE_CURVE('',#1971,#1918,#1117,.T.);
#2630=EDGE_CURVE('',#1970,#1912,#1118,.T.);
#2631=EDGE_CURVE('',#1969,#1917,#1119,.T.);
#2632=EDGE_CURVE('',#1968,#1913,#1120,.T.);
#2633=EDGE_CURVE('',#1967,#1916,#1121,.T.);
#2634=EDGE_CURVE('',#1966,#1914,#1122,.T.);
#2635=EDGE_CURVE('',#1965,#1915,#1123,.T.);
#3249=ORIENTED_EDGE('',*,*,#2289,.T.);
#3250=ORIENTED_EDGE('',*,*,#2290,.T.);
#3251=ORIENTED_EDGE('',*,*,#2291,.F.);
#3252=ORIENTED_EDGE('',*,*,#2292,.F.);
#3253=ORIENTED_EDGE('',*,*,#2293,.T.);
#3254=ORIENTED_EDGE('',*,*,#2294,.T.);
#3255=ORIENTED_EDGE('',*,*,#2295,.T.);
#3256=ORIENTED_EDGE('',*,*,#2289,.F.);
#3257=ORIENTED_EDGE('',*,*,#2296,.F.);
#3258=ORIENTED_EDGE('',*,*,#2297,.F.);
#3259=ORIENTED_EDGE('',*,*,#2298,.T.);
#3260=ORIENTED_EDGE('',*,*,#2299,.T.);
#3261=ORIENTED_EDGE('',*,*,#2300,.T.);
#3262=ORIENTED_EDGE('',*,*,#2293,.F.);
#3263=ORIENTED_EDGE('',*,*,#2301,.F.);
#3264=ORIENTED_EDGE('',*,*,#2302,.F.);
#3265=ORIENTED_EDGE('',*,*,#2303,.T.);
#3266=ORIENTED_EDGE('',*,*,#2304,.T.);
#3267=ORIENTED_EDGE('',*,*,#2305,.T.);
#3268=ORIENTED_EDGE('',*,*,#2298,.F.);
#3269=ORIENTED_EDGE('',*,*,#2306,.F.);
#3270=ORIENTED_EDGE('',*,*,#2307,.F.);
#3271=ORIENTED_EDGE('',*,*,#2308,.T.);
#3272=ORIENTED_EDGE('',*,*,#2309,.T.);
#3273=ORIENTED_EDGE('',*,*,#2310,.T.);
#3274=ORIENTED_EDGE('',*,*,#2303,.F.);
#3275=ORIENTED_EDGE('',*,*,#2311,.F.);
#3276=ORIENTED_EDGE('',*,*,#2312,.F.);
#3277=ORIENTED_EDGE('',*,*,#2313,.T.);
#3278=ORIENTED_EDGE('',*,*,#2314,.T.);
#3279=ORIENTED_EDGE('',*,*,#2315,.T.);
#3280=ORIENTED_EDGE('',*,*,#2308,.F.);
#3281=ORIENTED_EDGE('',*,*,#2316,.F.);
#3282=ORIENTED_EDGE('',*,*,#2317,.F.);
#3283=ORIENTED_EDGE('',*,*,#2318,.T.);
#3284=ORIENTED_EDGE('',*,*,#2319,.T.);
#3285=ORIENTED_EDGE('',*,*,#2320,.T.);
#3286=ORIENTED_EDGE('',*,*,#2313,.F.);
#3287=ORIENTED_EDGE('',*,*,#2321,.F.);
#3288=ORIENTED_EDGE('',*,*,#2322,.F.);
#3289=ORIENTED_EDGE('',*,*,#2323,.T.);
#3290=ORIENTED_EDGE('',*,*,#2324,.T.);
#3291=ORIENTED_EDGE('',*,*,#2325,.T.);
#3292=ORIENTED_EDGE('',*,*,#2318,.F.);
#3293=ORIENTED_EDGE('',*,*,#2326,.F.);
#3294=ORIENTED_EDGE('',*,*,#2327,.F.);
#3295=ORIENTED_EDGE('',*,*,#2328,.F.);
#3296=ORIENTED_EDGE('',*,*,#2329,.F.);
#3297=ORIENTED_EDGE('',*,*,#2330,.F.);
#3298=ORIENTED_EDGE('',*,*,#2331,.F.);
#3299=ORIENTED_EDGE('',*,*,#2332,.T.);
#3300=ORIENTED_EDGE('',*,*,#2333,.T.);
#3301=ORIENTED_EDGE('',*,*,#2334,.F.);
#3302=ORIENTED_EDGE('',*,*,#2335,.T.);
#3303=ORIENTED_EDGE('',*,*,#2336,.T.);
#3304=ORIENTED_EDGE('',*,*,#2337,.T.);
#3305=ORIENTED_EDGE('',*,*,#2338,.T.);
#3306=ORIENTED_EDGE('',*,*,#2339,.T.);
#3307=ORIENTED_EDGE('',*,*,#2340,.T.);
#3308=ORIENTED_EDGE('',*,*,#2341,.T.);
#3309=ORIENTED_EDGE('',*,*,#2342,.T.);
#3310=ORIENTED_EDGE('',*,*,#2343,.T.);
#3311=ORIENTED_EDGE('',*,*,#2344,.T.);
#3312=ORIENTED_EDGE('',*,*,#2345,.T.);
#3313=ORIENTED_EDGE('',*,*,#2346,.T.);
#3314=ORIENTED_EDGE('',*,*,#2347,.T.);
#3315=ORIENTED_EDGE('',*,*,#2348,.T.);
#3316=ORIENTED_EDGE('',*,*,#2328,.T.);
#3317=ORIENTED_EDGE('',*,*,#2349,.T.);
#3318=ORIENTED_EDGE('',*,*,#2350,.T.);
#3319=ORIENTED_EDGE('',*,*,#2323,.F.);
#3320=ORIENTED_EDGE('',*,*,#2351,.F.);
#3321=ORIENTED_EDGE('',*,*,#2352,.F.);
#3322=ORIENTED_EDGE('',*,*,#2353,.F.);
#3323=ORIENTED_EDGE('',*,*,#2290,.F.);
#3324=ORIENTED_EDGE('',*,*,#2295,.F.);
#3325=ORIENTED_EDGE('',*,*,#2294,.F.);
#3326=ORIENTED_EDGE('',*,*,#2300,.F.);
#3327=ORIENTED_EDGE('',*,*,#2299,.F.);
#3328=ORIENTED_EDGE('',*,*,#2305,.F.);
#3329=ORIENTED_EDGE('',*,*,#2304,.F.);
#3330=ORIENTED_EDGE('',*,*,#2310,.F.);
#3331=ORIENTED_EDGE('',*,*,#2309,.F.);
#3332=ORIENTED_EDGE('',*,*,#2315,.F.);
#3333=ORIENTED_EDGE('',*,*,#2314,.F.);
#3334=ORIENTED_EDGE('',*,*,#2320,.F.);
#3335=ORIENTED_EDGE('',*,*,#2319,.F.);
#3336=ORIENTED_EDGE('',*,*,#2325,.F.);
#3337=ORIENTED_EDGE('',*,*,#2324,.F.);
#3338=ORIENTED_EDGE('',*,*,#2350,.F.);
#3339=ORIENTED_EDGE('',*,*,#2349,.F.);
#3340=ORIENTED_EDGE('',*,*,#2333,.F.);
#3341=ORIENTED_EDGE('',*,*,#2332,.F.);
#3342=ORIENTED_EDGE('',*,*,#2354,.F.);
#3343=ORIENTED_EDGE('',*,*,#2341,.F.);
#3344=ORIENTED_EDGE('',*,*,#2340,.F.);
#3345=ORIENTED_EDGE('',*,*,#2339,.F.);
#3346=ORIENTED_EDGE('',*,*,#2338,.F.);
#3347=ORIENTED_EDGE('',*,*,#2337,.F.);
#3348=ORIENTED_EDGE('',*,*,#2336,.F.);
#3349=ORIENTED_EDGE('',*,*,#2335,.F.);
#3350=ORIENTED_EDGE('',*,*,#2355,.F.);
#3351=ORIENTED_EDGE('',*,*,#2348,.F.);
#3352=ORIENTED_EDGE('',*,*,#2347,.F.);
#3353=ORIENTED_EDGE('',*,*,#2346,.F.);
#3354=ORIENTED_EDGE('',*,*,#2345,.F.);
#3355=ORIENTED_EDGE('',*,*,#2344,.F.);
#3356=ORIENTED_EDGE('',*,*,#2343,.F.);
#3357=ORIENTED_EDGE('',*,*,#2356,.F.);
#3358=ORIENTED_EDGE('',*,*,#2330,.T.);
#3359=ORIENTED_EDGE('',*,*,#2329,.T.);
#3360=ORIENTED_EDGE('',*,*,#2352,.T.);
#3361=ORIENTED_EDGE('',*,*,#2351,.T.);
#3362=ORIENTED_EDGE('',*,*,#2327,.T.);
#3363=ORIENTED_EDGE('',*,*,#2326,.T.);
#3364=ORIENTED_EDGE('',*,*,#2322,.T.);
#3365=ORIENTED_EDGE('',*,*,#2321,.T.);
#3366=ORIENTED_EDGE('',*,*,#2317,.T.);
#3367=ORIENTED_EDGE('',*,*,#2316,.T.);
#3368=ORIENTED_EDGE('',*,*,#2312,.T.);
#3369=ORIENTED_EDGE('',*,*,#2311,.T.);
#3370=ORIENTED_EDGE('',*,*,#2307,.T.);
#3371=ORIENTED_EDGE('',*,*,#2306,.T.);
#3372=ORIENTED_EDGE('',*,*,#2302,.T.);
#3373=ORIENTED_EDGE('',*,*,#2301,.T.);
#3374=ORIENTED_EDGE('',*,*,#2297,.T.);
#3375=ORIENTED_EDGE('',*,*,#2296,.T.);
#3376=ORIENTED_EDGE('',*,*,#2292,.T.);
#3377=ORIENTED_EDGE('',*,*,#2357,.F.);
#3378=ORIENTED_EDGE('',*,*,#2358,.F.);
#3379=ORIENTED_EDGE('',*,*,#2354,.T.);
#3380=ORIENTED_EDGE('',*,*,#2331,.T.);
#3381=ORIENTED_EDGE('',*,*,#2356,.T.);
#3382=ORIENTED_EDGE('',*,*,#2342,.F.);
#3383=ORIENTED_EDGE('',*,*,#2359,.F.);
#3384=ORIENTED_EDGE('',*,*,#2360,.T.);
#3385=ORIENTED_EDGE('',*,*,#2361,.F.);
#3386=ORIENTED_EDGE('',*,*,#2362,.F.);
#3387=ORIENTED_EDGE('',*,*,#2363,.F.);
#3388=ORIENTED_EDGE('',*,*,#2364,.F.);
#3389=ORIENTED_EDGE('',*,*,#2365,.F.);
#3390=ORIENTED_EDGE('',*,*,#2360,.F.);
#3391=ORIENTED_EDGE('',*,*,#2359,.T.);
#3392=ORIENTED_EDGE('',*,*,#2353,.T.);
#3393=ORIENTED_EDGE('',*,*,#2334,.T.);
#3394=ORIENTED_EDGE('',*,*,#2355,.T.);
#3395=ORIENTED_EDGE('',*,*,#2291,.T.);
#3396=ORIENTED_EDGE('',*,*,#2358,.T.);
#3397=ORIENTED_EDGE('',*,*,#2366,.F.);
#3398=ORIENTED_EDGE('',*,*,#2357,.T.);
#3399=ORIENTED_EDGE('',*,*,#2367,.F.);
#3400=ORIENTED_EDGE('',*,*,#2368,.F.);
#3401=ORIENTED_EDGE('',*,*,#2369,.T.);
#3402=ORIENTED_EDGE('',*,*,#2370,.F.);
#3403=ORIENTED_EDGE('',*,*,#2371,.F.);
#3404=ORIENTED_EDGE('',*,*,#2372,.F.);
#3405=ORIENTED_EDGE('',*,*,#2373,.F.);
#3406=ORIENTED_EDGE('',*,*,#2374,.F.);
#3407=ORIENTED_EDGE('',*,*,#2369,.F.);
#3408=ORIENTED_EDGE('',*,*,#2370,.T.);
#3409=ORIENTED_EDGE('',*,*,#2374,.T.);
#3410=ORIENTED_EDGE('',*,*,#2375,.T.);
#3411=ORIENTED_EDGE('',*,*,#2376,.F.);
#3412=ORIENTED_EDGE('',*,*,#2377,.T.);
#3413=ORIENTED_EDGE('',*,*,#2378,.F.);
#3414=ORIENTED_EDGE('',*,*,#2379,.T.);
#3415=ORIENTED_EDGE('',*,*,#2373,.T.);
#3416=ORIENTED_EDGE('',*,*,#2380,.F.);
#3417=ORIENTED_EDGE('',*,*,#2381,.F.);
#3418=ORIENTED_EDGE('',*,*,#2375,.F.);
#3419=ORIENTED_EDGE('',*,*,#2361,.T.);
#3420=ORIENTED_EDGE('',*,*,#2365,.T.);
#3421=ORIENTED_EDGE('',*,*,#2382,.T.);
#3422=ORIENTED_EDGE('',*,*,#2383,.F.);
#3423=ORIENTED_EDGE('',*,*,#2384,.T.);
#3424=ORIENTED_EDGE('',*,*,#2385,.F.);
#3425=ORIENTED_EDGE('',*,*,#2386,.T.);
#3426=ORIENTED_EDGE('',*,*,#2364,.T.);
#3427=ORIENTED_EDGE('',*,*,#2387,.F.);
#3428=ORIENTED_EDGE('',*,*,#2388,.F.);
#3429=ORIENTED_EDGE('',*,*,#2382,.F.);
#3430=ORIENTED_EDGE('',*,*,#2389,.T.);
#3431=ORIENTED_EDGE('',*,*,#2390,.T.);
#3432=ORIENTED_EDGE('',*,*,#2391,.T.);
#3433=ORIENTED_EDGE('',*,*,#2376,.T.);
#3434=ORIENTED_EDGE('',*,*,#2392,.T.);
#3435=ORIENTED_EDGE('',*,*,#2393,.T.);
#3436=ORIENTED_EDGE('',*,*,#2391,.F.);
#3437=ORIENTED_EDGE('',*,*,#2394,.T.);
#3438=ORIENTED_EDGE('',*,*,#2395,.T.);
#3439=ORIENTED_EDGE('',*,*,#2396,.T.);
#3440=ORIENTED_EDGE('',*,*,#2392,.F.);
#3441=ORIENTED_EDGE('',*,*,#2397,.T.);
#3442=ORIENTED_EDGE('',*,*,#2398,.T.);
#3443=ORIENTED_EDGE('',*,*,#2399,.T.);
#3444=ORIENTED_EDGE('',*,*,#2395,.F.);
#3445=ORIENTED_EDGE('',*,*,#2400,.T.);
#3446=ORIENTED_EDGE('',*,*,#2401,.T.);
#3447=ORIENTED_EDGE('',*,*,#2402,.T.);
#3448=ORIENTED_EDGE('',*,*,#2398,.F.);
#3449=ORIENTED_EDGE('',*,*,#2403,.T.);
#3450=ORIENTED_EDGE('',*,*,#2404,.T.);
#3451=ORIENTED_EDGE('',*,*,#2405,.T.);
#3452=ORIENTED_EDGE('',*,*,#2401,.F.);
#3453=ORIENTED_EDGE('',*,*,#2406,.T.);
#3454=ORIENTED_EDGE('',*,*,#2407,.T.);
#3455=ORIENTED_EDGE('',*,*,#2408,.T.);
#3456=ORIENTED_EDGE('',*,*,#2404,.F.);
#3457=ORIENTED_EDGE('',*,*,#2409,.T.);
#3458=ORIENTED_EDGE('',*,*,#2410,.T.);
#3459=ORIENTED_EDGE('',*,*,#2411,.T.);
#3460=ORIENTED_EDGE('',*,*,#2407,.F.);
#3461=ORIENTED_EDGE('',*,*,#2412,.T.);
#3462=ORIENTED_EDGE('',*,*,#2413,.T.);
#3463=ORIENTED_EDGE('',*,*,#2414,.T.);
#3464=ORIENTED_EDGE('',*,*,#2410,.F.);
#3465=ORIENTED_EDGE('',*,*,#2415,.T.);
#3466=ORIENTED_EDGE('',*,*,#2416,.T.);
#3467=ORIENTED_EDGE('',*,*,#2417,.T.);
#3468=ORIENTED_EDGE('',*,*,#2413,.F.);
#3469=ORIENTED_EDGE('',*,*,#2418,.T.);
#3470=ORIENTED_EDGE('',*,*,#2419,.T.);
#3471=ORIENTED_EDGE('',*,*,#2420,.T.);
#3472=ORIENTED_EDGE('',*,*,#2416,.F.);
#3473=ORIENTED_EDGE('',*,*,#2421,.T.);
#3474=ORIENTED_EDGE('',*,*,#2422,.T.);
#3475=ORIENTED_EDGE('',*,*,#2423,.T.);
#3476=ORIENTED_EDGE('',*,*,#2419,.F.);
#3477=ORIENTED_EDGE('',*,*,#2424,.T.);
#3478=ORIENTED_EDGE('',*,*,#2425,.T.);
#3479=ORIENTED_EDGE('',*,*,#2426,.T.);
#3480=ORIENTED_EDGE('',*,*,#2422,.F.);
#3481=ORIENTED_EDGE('',*,*,#2427,.T.);
#3482=ORIENTED_EDGE('',*,*,#2428,.T.);
#3483=ORIENTED_EDGE('',*,*,#2429,.T.);
#3484=ORIENTED_EDGE('',*,*,#2425,.F.);
#3485=ORIENTED_EDGE('',*,*,#2430,.T.);
#3486=ORIENTED_EDGE('',*,*,#2431,.T.);
#3487=ORIENTED_EDGE('',*,*,#2385,.T.);
#3488=ORIENTED_EDGE('',*,*,#2428,.F.);
#3489=ORIENTED_EDGE('',*,*,#2432,.T.);
#3490=ORIENTED_EDGE('',*,*,#2433,.T.);
#3491=ORIENTED_EDGE('',*,*,#2434,.T.);
#3492=ORIENTED_EDGE('',*,*,#2431,.F.);
#3493=ORIENTED_EDGE('',*,*,#2435,.T.);
#3494=ORIENTED_EDGE('',*,*,#2436,.T.);
#3495=ORIENTED_EDGE('',*,*,#2437,.T.);
#3496=ORIENTED_EDGE('',*,*,#2433,.F.);
#3497=ORIENTED_EDGE('',*,*,#2438,.T.);
#3498=ORIENTED_EDGE('',*,*,#2439,.T.);
#3499=ORIENTED_EDGE('',*,*,#2440,.T.);
#3500=ORIENTED_EDGE('',*,*,#2436,.F.);
#3501=ORIENTED_EDGE('',*,*,#2441,.T.);
#3502=ORIENTED_EDGE('',*,*,#2442,.T.);
#3503=ORIENTED_EDGE('',*,*,#2443,.T.);
#3504=ORIENTED_EDGE('',*,*,#2439,.F.);
#3505=ORIENTED_EDGE('',*,*,#2444,.T.);
#3506=ORIENTED_EDGE('',*,*,#2445,.T.);
#3507=ORIENTED_EDGE('',*,*,#2446,.T.);
#3508=ORIENTED_EDGE('',*,*,#2442,.F.);
#3509=ORIENTED_EDGE('',*,*,#2447,.T.);
#3510=ORIENTED_EDGE('',*,*,#2448,.T.);
#3511=ORIENTED_EDGE('',*,*,#2449,.T.);
#3512=ORIENTED_EDGE('',*,*,#2445,.F.);
#3513=ORIENTED_EDGE('',*,*,#2450,.T.);
#3514=ORIENTED_EDGE('',*,*,#2451,.T.);
#3515=ORIENTED_EDGE('',*,*,#2452,.T.);
#3516=ORIENTED_EDGE('',*,*,#2448,.F.);
#3517=ORIENTED_EDGE('',*,*,#2453,.T.);
#3518=ORIENTED_EDGE('',*,*,#2454,.T.);
#3519=ORIENTED_EDGE('',*,*,#2455,.T.);
#3520=ORIENTED_EDGE('',*,*,#2451,.F.);
#3521=ORIENTED_EDGE('',*,*,#2456,.T.);
#3522=ORIENTED_EDGE('',*,*,#2457,.T.);
#3523=ORIENTED_EDGE('',*,*,#2458,.T.);
#3524=ORIENTED_EDGE('',*,*,#2454,.F.);
#3525=ORIENTED_EDGE('',*,*,#2459,.T.);
#3526=ORIENTED_EDGE('',*,*,#2460,.T.);
#3527=ORIENTED_EDGE('',*,*,#2461,.T.);
#3528=ORIENTED_EDGE('',*,*,#2457,.F.);
#3529=ORIENTED_EDGE('',*,*,#2462,.T.);
#3530=ORIENTED_EDGE('',*,*,#2463,.T.);
#3531=ORIENTED_EDGE('',*,*,#2464,.T.);
#3532=ORIENTED_EDGE('',*,*,#2460,.F.);
#3533=ORIENTED_EDGE('',*,*,#2465,.T.);
#3534=ORIENTED_EDGE('',*,*,#2466,.T.);
#3535=ORIENTED_EDGE('',*,*,#2467,.T.);
#3536=ORIENTED_EDGE('',*,*,#2463,.F.);
#3537=ORIENTED_EDGE('',*,*,#2468,.T.);
#3538=ORIENTED_EDGE('',*,*,#2469,.T.);
#3539=ORIENTED_EDGE('',*,*,#2470,.T.);
#3540=ORIENTED_EDGE('',*,*,#2466,.F.);
#3541=ORIENTED_EDGE('',*,*,#2471,.T.);
#3542=ORIENTED_EDGE('',*,*,#2472,.T.);
#3543=ORIENTED_EDGE('',*,*,#2473,.T.);
#3544=ORIENTED_EDGE('',*,*,#2469,.F.);
#3545=ORIENTED_EDGE('',*,*,#2474,.T.);
#3546=ORIENTED_EDGE('',*,*,#2475,.T.);
#3547=ORIENTED_EDGE('',*,*,#2476,.T.);
#3548=ORIENTED_EDGE('',*,*,#2472,.F.);
#3549=ORIENTED_EDGE('',*,*,#2477,.T.);
#3550=ORIENTED_EDGE('',*,*,#2478,.T.);
#3551=ORIENTED_EDGE('',*,*,#2479,.T.);
#3552=ORIENTED_EDGE('',*,*,#2475,.F.);
#3553=ORIENTED_EDGE('',*,*,#2480,.T.);
#3554=ORIENTED_EDGE('',*,*,#2478,.F.);
#3555=ORIENTED_EDGE('',*,*,#2481,.T.);
#3556=ORIENTED_EDGE('',*,*,#2389,.F.);
#3557=ORIENTED_EDGE('',*,*,#2381,.T.);
#3558=ORIENTED_EDGE('',*,*,#2440,.F.);
#3559=ORIENTED_EDGE('',*,*,#2482,.F.);
#3560=ORIENTED_EDGE('',*,*,#2483,.F.);
#3561=ORIENTED_EDGE('',*,*,#2484,.F.);
#3562=ORIENTED_EDGE('',*,*,#2443,.F.);
#3563=ORIENTED_EDGE('',*,*,#2485,.T.);
#3564=ORIENTED_EDGE('',*,*,#2486,.F.);
#3565=ORIENTED_EDGE('',*,*,#2482,.T.);
#3566=ORIENTED_EDGE('',*,*,#2446,.F.);
#3567=ORIENTED_EDGE('',*,*,#2487,.F.);
#3568=ORIENTED_EDGE('',*,*,#2488,.F.);
#3569=ORIENTED_EDGE('',*,*,#2485,.F.);
#3570=ORIENTED_EDGE('',*,*,#2449,.F.);
#3571=ORIENTED_EDGE('',*,*,#2489,.T.);
#3572=ORIENTED_EDGE('',*,*,#2490,.F.);
#3573=ORIENTED_EDGE('',*,*,#2487,.T.);
#3574=ORIENTED_EDGE('',*,*,#2452,.F.);
#3575=ORIENTED_EDGE('',*,*,#2491,.F.);
#3576=ORIENTED_EDGE('',*,*,#2492,.F.);
#3577=ORIENTED_EDGE('',*,*,#2489,.F.);
#3578=ORIENTED_EDGE('',*,*,#2455,.F.);
#3579=ORIENTED_EDGE('',*,*,#2493,.T.);
#3580=ORIENTED_EDGE('',*,*,#2494,.F.);
#3581=ORIENTED_EDGE('',*,*,#2491,.T.);
#3582=ORIENTED_EDGE('',*,*,#2458,.F.);
#3583=ORIENTED_EDGE('',*,*,#2495,.F.);
#3584=ORIENTED_EDGE('',*,*,#2496,.F.);
#3585=ORIENTED_EDGE('',*,*,#2493,.F.);
#3586=ORIENTED_EDGE('',*,*,#2461,.F.);
#3587=ORIENTED_EDGE('',*,*,#2497,.T.);
#3588=ORIENTED_EDGE('',*,*,#2498,.F.);
#3589=ORIENTED_EDGE('',*,*,#2495,.T.);
#3590=ORIENTED_EDGE('',*,*,#2464,.F.);
#3591=ORIENTED_EDGE('',*,*,#2499,.F.);
#3592=ORIENTED_EDGE('',*,*,#2500,.F.);
#3593=ORIENTED_EDGE('',*,*,#2497,.F.);
#3594=ORIENTED_EDGE('',*,*,#2467,.F.);
#3595=ORIENTED_EDGE('',*,*,#2501,.T.);
#3596=ORIENTED_EDGE('',*,*,#2502,.F.);
#3597=ORIENTED_EDGE('',*,*,#2499,.T.);
#3598=ORIENTED_EDGE('',*,*,#2470,.F.);
#3599=ORIENTED_EDGE('',*,*,#2503,.F.);
#3600=ORIENTED_EDGE('',*,*,#2504,.F.);
#3601=ORIENTED_EDGE('',*,*,#2501,.F.);
#3602=ORIENTED_EDGE('',*,*,#2473,.F.);
#3603=ORIENTED_EDGE('',*,*,#2505,.T.);
#3604=ORIENTED_EDGE('',*,*,#2506,.F.);
#3605=ORIENTED_EDGE('',*,*,#2503,.T.);
#3606=ORIENTED_EDGE('',*,*,#2476,.F.);
#3607=ORIENTED_EDGE('',*,*,#2507,.F.);
#3608=ORIENTED_EDGE('',*,*,#2508,.F.);
#3609=ORIENTED_EDGE('',*,*,#2505,.F.);
#3610=ORIENTED_EDGE('',*,*,#2372,.T.);
#3611=ORIENTED_EDGE('',*,*,#2509,.T.);
#3612=ORIENTED_EDGE('',*,*,#2510,.F.);
#3613=ORIENTED_EDGE('',*,*,#2507,.T.);
#3614=ORIENTED_EDGE('',*,*,#2479,.F.);
#3615=ORIENTED_EDGE('',*,*,#2380,.T.);
#3616=ORIENTED_EDGE('',*,*,#2371,.T.);
#3617=ORIENTED_EDGE('',*,*,#2379,.F.);
#3618=ORIENTED_EDGE('',*,*,#2511,.F.);
#3619=ORIENTED_EDGE('',*,*,#2509,.F.);
#3620=ORIENTED_EDGE('',*,*,#2390,.F.);
#3621=ORIENTED_EDGE('',*,*,#2481,.F.);
#3622=ORIENTED_EDGE('',*,*,#2480,.F.);
#3623=ORIENTED_EDGE('',*,*,#2477,.F.);
#3624=ORIENTED_EDGE('',*,*,#2474,.F.);
#3625=ORIENTED_EDGE('',*,*,#2471,.F.);
#3626=ORIENTED_EDGE('',*,*,#2468,.F.);
#3627=ORIENTED_EDGE('',*,*,#2465,.F.);
#3628=ORIENTED_EDGE('',*,*,#2462,.F.);
#3629=ORIENTED_EDGE('',*,*,#2459,.F.);
#3630=ORIENTED_EDGE('',*,*,#2456,.F.);
#3631=ORIENTED_EDGE('',*,*,#2453,.F.);
#3632=ORIENTED_EDGE('',*,*,#2450,.F.);
#3633=ORIENTED_EDGE('',*,*,#2447,.F.);
#3634=ORIENTED_EDGE('',*,*,#2444,.F.);
#3635=ORIENTED_EDGE('',*,*,#2441,.F.);
#3636=ORIENTED_EDGE('',*,*,#2438,.F.);
#3637=ORIENTED_EDGE('',*,*,#2435,.F.);
#3638=ORIENTED_EDGE('',*,*,#2432,.F.);
#3639=ORIENTED_EDGE('',*,*,#2430,.F.);
#3640=ORIENTED_EDGE('',*,*,#2427,.F.);
#3641=ORIENTED_EDGE('',*,*,#2424,.F.);
#3642=ORIENTED_EDGE('',*,*,#2421,.F.);
#3643=ORIENTED_EDGE('',*,*,#2418,.F.);
#3644=ORIENTED_EDGE('',*,*,#2415,.F.);
#3645=ORIENTED_EDGE('',*,*,#2412,.F.);
#3646=ORIENTED_EDGE('',*,*,#2409,.F.);
#3647=ORIENTED_EDGE('',*,*,#2406,.F.);
#3648=ORIENTED_EDGE('',*,*,#2403,.F.);
#3649=ORIENTED_EDGE('',*,*,#2400,.F.);
#3650=ORIENTED_EDGE('',*,*,#2397,.F.);
#3651=ORIENTED_EDGE('',*,*,#2394,.F.);
#3652=ORIENTED_EDGE('',*,*,#2512,.F.);
#3653=ORIENTED_EDGE('',*,*,#2513,.T.);
#3654=ORIENTED_EDGE('',*,*,#2514,.T.);
#3655=ORIENTED_EDGE('',*,*,#2515,.T.);
#3656=ORIENTED_EDGE('',*,*,#2516,.T.);
#3657=ORIENTED_EDGE('',*,*,#2517,.T.);
#3658=ORIENTED_EDGE('',*,*,#2518,.T.);
#3659=ORIENTED_EDGE('',*,*,#2519,.T.);
#3660=ORIENTED_EDGE('',*,*,#2520,.T.);
#3661=ORIENTED_EDGE('',*,*,#2521,.T.);
#3662=ORIENTED_EDGE('',*,*,#2522,.T.);
#3663=ORIENTED_EDGE('',*,*,#2523,.T.);
#3664=ORIENTED_EDGE('',*,*,#2524,.T.);
#3665=ORIENTED_EDGE('',*,*,#2525,.T.);
#3666=ORIENTED_EDGE('',*,*,#2526,.T.);
#3667=ORIENTED_EDGE('',*,*,#2523,.F.);
#3668=ORIENTED_EDGE('',*,*,#2527,.T.);
#3669=ORIENTED_EDGE('',*,*,#2528,.T.);
#3670=ORIENTED_EDGE('',*,*,#2378,.T.);
#3671=ORIENTED_EDGE('',*,*,#2525,.F.);
#3672=ORIENTED_EDGE('',*,*,#2529,.T.);
#3673=ORIENTED_EDGE('',*,*,#2530,.T.);
#3674=ORIENTED_EDGE('',*,*,#2511,.T.);
#3675=ORIENTED_EDGE('',*,*,#2528,.F.);
#3676=ORIENTED_EDGE('',*,*,#2531,.T.);
#3677=ORIENTED_EDGE('',*,*,#2532,.T.);
#3678=ORIENTED_EDGE('',*,*,#2510,.T.);
#3679=ORIENTED_EDGE('',*,*,#2530,.F.);
#3680=ORIENTED_EDGE('',*,*,#2533,.T.);
#3681=ORIENTED_EDGE('',*,*,#2534,.T.);
#3682=ORIENTED_EDGE('',*,*,#2508,.T.);
#3683=ORIENTED_EDGE('',*,*,#2532,.F.);
#3684=ORIENTED_EDGE('',*,*,#2535,.T.);
#3685=ORIENTED_EDGE('',*,*,#2536,.T.);
#3686=ORIENTED_EDGE('',*,*,#2506,.T.);
#3687=ORIENTED_EDGE('',*,*,#2534,.F.);
#3688=ORIENTED_EDGE('',*,*,#2537,.T.);
#3689=ORIENTED_EDGE('',*,*,#2538,.T.);
#3690=ORIENTED_EDGE('',*,*,#2504,.T.);
#3691=ORIENTED_EDGE('',*,*,#2536,.F.);
#3692=ORIENTED_EDGE('',*,*,#2539,.T.);
#3693=ORIENTED_EDGE('',*,*,#2540,.T.);
#3694=ORIENTED_EDGE('',*,*,#2502,.T.);
#3695=ORIENTED_EDGE('',*,*,#2538,.F.);
#3696=ORIENTED_EDGE('',*,*,#2541,.T.);
#3697=ORIENTED_EDGE('',*,*,#2542,.T.);
#3698=ORIENTED_EDGE('',*,*,#2500,.T.);
#3699=ORIENTED_EDGE('',*,*,#2540,.F.);
#3700=ORIENTED_EDGE('',*,*,#2543,.T.);
#3701=ORIENTED_EDGE('',*,*,#2544,.T.);
#3702=ORIENTED_EDGE('',*,*,#2498,.T.);
#3703=ORIENTED_EDGE('',*,*,#2542,.F.);
#3704=ORIENTED_EDGE('',*,*,#2545,.T.);
#3705=ORIENTED_EDGE('',*,*,#2546,.T.);
#3706=ORIENTED_EDGE('',*,*,#2496,.T.);
#3707=ORIENTED_EDGE('',*,*,#2544,.F.);
#3708=ORIENTED_EDGE('',*,*,#2547,.T.);
#3709=ORIENTED_EDGE('',*,*,#2548,.T.);
#3710=ORIENTED_EDGE('',*,*,#2494,.T.);
#3711=ORIENTED_EDGE('',*,*,#2546,.F.);
#3712=ORIENTED_EDGE('',*,*,#2549,.T.);
#3713=ORIENTED_EDGE('',*,*,#2550,.T.);
#3714=ORIENTED_EDGE('',*,*,#2492,.T.);
#3715=ORIENTED_EDGE('',*,*,#2548,.F.);
#3716=ORIENTED_EDGE('',*,*,#2551,.T.);
#3717=ORIENTED_EDGE('',*,*,#2552,.T.);
#3718=ORIENTED_EDGE('',*,*,#2490,.T.);
#3719=ORIENTED_EDGE('',*,*,#2550,.F.);
#3720=ORIENTED_EDGE('',*,*,#2553,.T.);
#3721=ORIENTED_EDGE('',*,*,#2554,.T.);
#3722=ORIENTED_EDGE('',*,*,#2488,.T.);
#3723=ORIENTED_EDGE('',*,*,#2552,.F.);
#3724=ORIENTED_EDGE('',*,*,#2555,.T.);
#3725=ORIENTED_EDGE('',*,*,#2556,.T.);
#3726=ORIENTED_EDGE('',*,*,#2486,.T.);
#3727=ORIENTED_EDGE('',*,*,#2554,.F.);
#3728=ORIENTED_EDGE('',*,*,#2557,.T.);
#3729=ORIENTED_EDGE('',*,*,#2558,.T.);
#3730=ORIENTED_EDGE('',*,*,#2483,.T.);
#3731=ORIENTED_EDGE('',*,*,#2556,.F.);
#3732=ORIENTED_EDGE('',*,*,#2559,.T.);
#3733=ORIENTED_EDGE('',*,*,#2560,.T.);
#3734=ORIENTED_EDGE('',*,*,#2561,.T.);
#3735=ORIENTED_EDGE('',*,*,#2558,.F.);
#3736=ORIENTED_EDGE('',*,*,#2562,.T.);
#3737=ORIENTED_EDGE('',*,*,#2563,.T.);
#3738=ORIENTED_EDGE('',*,*,#2388,.T.);
#3739=ORIENTED_EDGE('',*,*,#2560,.F.);
#3740=ORIENTED_EDGE('',*,*,#2564,.T.);
#3741=ORIENTED_EDGE('',*,*,#2565,.T.);
#3742=ORIENTED_EDGE('',*,*,#2383,.T.);
#3743=ORIENTED_EDGE('',*,*,#2563,.F.);
#3744=ORIENTED_EDGE('',*,*,#2566,.T.);
#3745=ORIENTED_EDGE('',*,*,#2567,.T.);
#3746=ORIENTED_EDGE('',*,*,#2568,.T.);
#3747=ORIENTED_EDGE('',*,*,#2565,.F.);
#3748=ORIENTED_EDGE('',*,*,#2569,.T.);
#3749=ORIENTED_EDGE('',*,*,#2570,.T.);
#3750=ORIENTED_EDGE('',*,*,#2571,.T.);
#3751=ORIENTED_EDGE('',*,*,#2567,.F.);
#3752=ORIENTED_EDGE('',*,*,#2572,.T.);
#3753=ORIENTED_EDGE('',*,*,#2573,.T.);
#3754=ORIENTED_EDGE('',*,*,#2574,.T.);
#3755=ORIENTED_EDGE('',*,*,#2570,.F.);
#3756=ORIENTED_EDGE('',*,*,#2575,.T.);
#3757=ORIENTED_EDGE('',*,*,#2576,.T.);
#3758=ORIENTED_EDGE('',*,*,#2577,.T.);
#3759=ORIENTED_EDGE('',*,*,#2573,.F.);
#3760=ORIENTED_EDGE('',*,*,#2578,.T.);
#3761=ORIENTED_EDGE('',*,*,#2579,.T.);
#3762=ORIENTED_EDGE('',*,*,#2580,.T.);
#3763=ORIENTED_EDGE('',*,*,#2576,.F.);
#3764=ORIENTED_EDGE('',*,*,#2581,.T.);
#3765=ORIENTED_EDGE('',*,*,#2582,.T.);
#3766=ORIENTED_EDGE('',*,*,#2583,.T.);
#3767=ORIENTED_EDGE('',*,*,#2579,.F.);
#3768=ORIENTED_EDGE('',*,*,#2584,.T.);
#3769=ORIENTED_EDGE('',*,*,#2585,.T.);
#3770=ORIENTED_EDGE('',*,*,#2586,.T.);
#3771=ORIENTED_EDGE('',*,*,#2582,.F.);
#3772=ORIENTED_EDGE('',*,*,#2587,.T.);
#3773=ORIENTED_EDGE('',*,*,#2588,.T.);
#3774=ORIENTED_EDGE('',*,*,#2589,.T.);
#3775=ORIENTED_EDGE('',*,*,#2585,.F.);
#3776=ORIENTED_EDGE('',*,*,#2590,.T.);
#3777=ORIENTED_EDGE('',*,*,#2591,.T.);
#3778=ORIENTED_EDGE('',*,*,#2592,.T.);
#3779=ORIENTED_EDGE('',*,*,#2588,.F.);
#3780=ORIENTED_EDGE('',*,*,#2593,.T.);
#3781=ORIENTED_EDGE('',*,*,#2594,.T.);
#3782=ORIENTED_EDGE('',*,*,#2595,.T.);
#3783=ORIENTED_EDGE('',*,*,#2591,.F.);
#3784=ORIENTED_EDGE('',*,*,#2596,.T.);
#3785=ORIENTED_EDGE('',*,*,#2594,.F.);
#3786=ORIENTED_EDGE('',*,*,#2597,.T.);
#3787=ORIENTED_EDGE('',*,*,#2521,.F.);
#3788=ORIENTED_EDGE('',*,*,#2598,.T.);
#3789=ORIENTED_EDGE('',*,*,#2363,.T.);
#3790=ORIENTED_EDGE('',*,*,#2599,.T.);
#3791=ORIENTED_EDGE('',*,*,#2437,.F.);
#3792=ORIENTED_EDGE('',*,*,#2484,.T.);
#3793=ORIENTED_EDGE('',*,*,#2561,.F.);
#3794=ORIENTED_EDGE('',*,*,#2387,.T.);
#3795=ORIENTED_EDGE('',*,*,#2362,.T.);
#3796=ORIENTED_EDGE('',*,*,#2386,.F.);
#3797=ORIENTED_EDGE('',*,*,#2434,.F.);
#3798=ORIENTED_EDGE('',*,*,#2599,.F.);
#3799=ORIENTED_EDGE('',*,*,#2429,.F.);
#3800=ORIENTED_EDGE('',*,*,#2384,.F.);
#3801=ORIENTED_EDGE('',*,*,#2568,.F.);
#3802=ORIENTED_EDGE('',*,*,#2600,.F.);
#3803=ORIENTED_EDGE('',*,*,#2426,.F.);
#3804=ORIENTED_EDGE('',*,*,#2600,.T.);
#3805=ORIENTED_EDGE('',*,*,#2571,.F.);
#3806=ORIENTED_EDGE('',*,*,#2601,.T.);
#3807=ORIENTED_EDGE('',*,*,#2423,.F.);
#3808=ORIENTED_EDGE('',*,*,#2601,.F.);
#3809=ORIENTED_EDGE('',*,*,#2574,.F.);
#3810=ORIENTED_EDGE('',*,*,#2602,.F.);
#3811=ORIENTED_EDGE('',*,*,#2420,.F.);
#3812=ORIENTED_EDGE('',*,*,#2602,.T.);
#3813=ORIENTED_EDGE('',*,*,#2577,.F.);
#3814=ORIENTED_EDGE('',*,*,#2603,.T.);
#3815=ORIENTED_EDGE('',*,*,#2417,.F.);
#3816=ORIENTED_EDGE('',*,*,#2603,.F.);
#3817=ORIENTED_EDGE('',*,*,#2580,.F.);
#3818=ORIENTED_EDGE('',*,*,#2604,.F.);
#3819=ORIENTED_EDGE('',*,*,#2414,.F.);
#3820=ORIENTED_EDGE('',*,*,#2604,.T.);
#3821=ORIENTED_EDGE('',*,*,#2583,.F.);
#3822=ORIENTED_EDGE('',*,*,#2605,.T.);
#3823=ORIENTED_EDGE('',*,*,#2411,.F.);
#3824=ORIENTED_EDGE('',*,*,#2605,.F.);
#3825=ORIENTED_EDGE('',*,*,#2586,.F.);
#3826=ORIENTED_EDGE('',*,*,#2606,.F.);
#3827=ORIENTED_EDGE('',*,*,#2408,.F.);
#3828=ORIENTED_EDGE('',*,*,#2606,.T.);
#3829=ORIENTED_EDGE('',*,*,#2589,.F.);
#3830=ORIENTED_EDGE('',*,*,#2607,.T.);
#3831=ORIENTED_EDGE('',*,*,#2405,.F.);
#3832=ORIENTED_EDGE('',*,*,#2607,.F.);
#3833=ORIENTED_EDGE('',*,*,#2592,.F.);
#3834=ORIENTED_EDGE('',*,*,#2608,.F.);
#3835=ORIENTED_EDGE('',*,*,#2402,.F.);
#3836=ORIENTED_EDGE('',*,*,#2608,.T.);
#3837=ORIENTED_EDGE('',*,*,#2595,.F.);
#3838=ORIENTED_EDGE('',*,*,#2609,.T.);
#3839=ORIENTED_EDGE('',*,*,#2399,.F.);
#3840=ORIENTED_EDGE('',*,*,#2609,.F.);
#3841=ORIENTED_EDGE('',*,*,#2598,.F.);
#3842=ORIENTED_EDGE('',*,*,#2610,.F.);
#3843=ORIENTED_EDGE('',*,*,#2396,.F.);
#3844=ORIENTED_EDGE('',*,*,#2610,.T.);
#3845=ORIENTED_EDGE('',*,*,#2524,.F.);
#3846=ORIENTED_EDGE('',*,*,#2611,.T.);
#3847=ORIENTED_EDGE('',*,*,#2522,.F.);
#3848=ORIENTED_EDGE('',*,*,#2597,.F.);
#3849=ORIENTED_EDGE('',*,*,#2596,.F.);
#3850=ORIENTED_EDGE('',*,*,#2593,.F.);
#3851=ORIENTED_EDGE('',*,*,#2590,.F.);
#3852=ORIENTED_EDGE('',*,*,#2587,.F.);
#3853=ORIENTED_EDGE('',*,*,#2584,.F.);
#3854=ORIENTED_EDGE('',*,*,#2581,.F.);
#3855=ORIENTED_EDGE('',*,*,#2578,.F.);
#3856=ORIENTED_EDGE('',*,*,#2575,.F.);
#3857=ORIENTED_EDGE('',*,*,#2572,.F.);
#3858=ORIENTED_EDGE('',*,*,#2569,.F.);
#3859=ORIENTED_EDGE('',*,*,#2566,.F.);
#3860=ORIENTED_EDGE('',*,*,#2564,.F.);
#3861=ORIENTED_EDGE('',*,*,#2562,.F.);
#3862=ORIENTED_EDGE('',*,*,#2559,.F.);
#3863=ORIENTED_EDGE('',*,*,#2557,.F.);
#3864=ORIENTED_EDGE('',*,*,#2555,.F.);
#3865=ORIENTED_EDGE('',*,*,#2553,.F.);
#3866=ORIENTED_EDGE('',*,*,#2551,.F.);
#3867=ORIENTED_EDGE('',*,*,#2549,.F.);
#3868=ORIENTED_EDGE('',*,*,#2547,.F.);
#3869=ORIENTED_EDGE('',*,*,#2545,.F.);
#3870=ORIENTED_EDGE('',*,*,#2543,.F.);
#3871=ORIENTED_EDGE('',*,*,#2541,.F.);
#3872=ORIENTED_EDGE('',*,*,#2539,.F.);
#3873=ORIENTED_EDGE('',*,*,#2537,.F.);
#3874=ORIENTED_EDGE('',*,*,#2535,.F.);
#3875=ORIENTED_EDGE('',*,*,#2533,.F.);
#3876=ORIENTED_EDGE('',*,*,#2531,.F.);
#3877=ORIENTED_EDGE('',*,*,#2529,.F.);
#3878=ORIENTED_EDGE('',*,*,#2527,.F.);
#3879=ORIENTED_EDGE('',*,*,#2612,.F.);
#3880=ORIENTED_EDGE('',*,*,#2613,.T.);
#3881=ORIENTED_EDGE('',*,*,#2614,.T.);
#3882=ORIENTED_EDGE('',*,*,#2615,.T.);
#3883=ORIENTED_EDGE('',*,*,#2616,.T.);
#3884=ORIENTED_EDGE('',*,*,#2617,.T.);
#3885=ORIENTED_EDGE('',*,*,#2618,.T.);
#3886=ORIENTED_EDGE('',*,*,#2619,.T.);
#3887=ORIENTED_EDGE('',*,*,#2620,.T.);
#3888=ORIENTED_EDGE('',*,*,#2512,.T.);
#3889=ORIENTED_EDGE('',*,*,#2621,.T.);
#3890=ORIENTED_EDGE('',*,*,#2622,.T.);
#3891=ORIENTED_EDGE('',*,*,#2623,.T.);
#3892=ORIENTED_EDGE('',*,*,#2621,.F.);
#3893=ORIENTED_EDGE('',*,*,#2623,.F.);
#3894=ORIENTED_EDGE('',*,*,#2624,.T.);
#3895=ORIENTED_EDGE('',*,*,#2625,.F.);
#3896=ORIENTED_EDGE('',*,*,#2626,.F.);
#3897=ORIENTED_EDGE('',*,*,#2624,.F.);
#3898=ORIENTED_EDGE('',*,*,#2622,.F.);
#3899=ORIENTED_EDGE('',*,*,#2368,.T.);
#3900=ORIENTED_EDGE('',*,*,#2367,.T.);
#3901=ORIENTED_EDGE('',*,*,#2366,.T.);
#3902=ORIENTED_EDGE('',*,*,#2612,.T.);
#3903=ORIENTED_EDGE('',*,*,#2627,.T.);
#3904=ORIENTED_EDGE('',*,*,#2625,.T.);
#3905=ORIENTED_EDGE('',*,*,#2626,.T.);
#3906=ORIENTED_EDGE('',*,*,#2627,.F.);
#3907=ORIENTED_EDGE('',*,*,#2393,.F.);
#3908=ORIENTED_EDGE('',*,*,#2611,.F.);
#3909=ORIENTED_EDGE('',*,*,#2526,.F.);
#3910=ORIENTED_EDGE('',*,*,#2377,.F.);
#3911=ORIENTED_EDGE('',*,*,#2613,.F.);
#3912=ORIENTED_EDGE('',*,*,#2628,.T.);
#3913=ORIENTED_EDGE('',*,*,#2513,.F.);
#3914=ORIENTED_EDGE('',*,*,#2628,.F.);
#3915=ORIENTED_EDGE('',*,*,#2620,.F.);
#3916=ORIENTED_EDGE('',*,*,#2629,.T.);
#3917=ORIENTED_EDGE('',*,*,#2520,.F.);
#3918=ORIENTED_EDGE('',*,*,#2629,.F.);
#3919=ORIENTED_EDGE('',*,*,#2619,.F.);
#3920=ORIENTED_EDGE('',*,*,#2630,.T.);
#3921=ORIENTED_EDGE('',*,*,#2514,.F.);
#3922=ORIENTED_EDGE('',*,*,#2630,.F.);
#3923=ORIENTED_EDGE('',*,*,#2618,.F.);
#3924=ORIENTED_EDGE('',*,*,#2631,.T.);
#3925=ORIENTED_EDGE('',*,*,#2519,.F.);
#3926=ORIENTED_EDGE('',*,*,#2631,.F.);
#3927=ORIENTED_EDGE('',*,*,#2617,.F.);
#3928=ORIENTED_EDGE('',*,*,#2632,.T.);
#3929=ORIENTED_EDGE('',*,*,#2515,.F.);
#3930=ORIENTED_EDGE('',*,*,#2632,.F.);
#3931=ORIENTED_EDGE('',*,*,#2616,.F.);
#3932=ORIENTED_EDGE('',*,*,#2633,.T.);
#3933=ORIENTED_EDGE('',*,*,#2518,.F.);
#3934=ORIENTED_EDGE('',*,*,#2633,.F.);
#3935=ORIENTED_EDGE('',*,*,#2615,.F.);
#3936=ORIENTED_EDGE('',*,*,#2634,.T.);
#3937=ORIENTED_EDGE('',*,*,#2516,.F.);
#3938=ORIENTED_EDGE('',*,*,#2634,.F.);
#3939=ORIENTED_EDGE('',*,*,#2614,.F.);
#3940=ORIENTED_EDGE('',*,*,#2635,.T.);
#3941=ORIENTED_EDGE('',*,*,#2517,.F.);
#3942=ORIENTED_EDGE('',*,*,#2635,.F.);
#4086=CYLINDRICAL_SURFACE('',#4605,4.085);
#4087=CYLINDRICAL_SURFACE('',#4607,4.085);
#4088=CYLINDRICAL_SURFACE('',#4608,4.085);
#4089=CYLINDRICAL_SURFACE('',#4609,4.085);
#4090=CYLINDRICAL_SURFACE('',#4610,4.085);
#4091=CYLINDRICAL_SURFACE('',#4611,4.085);
#4092=CYLINDRICAL_SURFACE('',#4612,4.085);
#4093=CYLINDRICAL_SURFACE('',#4613,4.085);
#4094=CYLINDRICAL_SURFACE('',#4614,4.085);
#4095=CYLINDRICAL_SURFACE('',#4616,3.38975);
#4096=CYLINDRICAL_SURFACE('',#4619,4.085);
#4097=CYLINDRICAL_SURFACE('',#4623,5.);
#4098=CYLINDRICAL_SURFACE('',#4626,5.);
#4099=CYLINDRICAL_SURFACE('',#4627,5.);
#4100=CYLINDRICAL_SURFACE('',#4628,5.);
#4101=CYLINDRICAL_SURFACE('',#4629,4.);
#4102=CYLINDRICAL_SURFACE('',#4632,31.);
#4103=CYLINDRICAL_SURFACE('',#4634,4.);
#4104=CYLINDRICAL_SURFACE('',#4637,31.);
#4105=CYLINDRICAL_SURFACE('',#4764,6.5);
#4106=CYLINDRICAL_SURFACE('',#4766,4.);
#4107=CYLINDRICAL_SURFACE('',#4768,31.);
#4108=CYLINDRICAL_SURFACE('',#4770,4.);
#4109=CYLINDRICAL_SURFACE('',#4772,6.5);
#4110=CYLINDRICAL_SURFACE('',#4774,4.);
#4111=CYLINDRICAL_SURFACE('',#4776,31.);
#4112=CYLINDRICAL_SURFACE('',#4778,4.);
#4113=CYLINDRICAL_SURFACE('',#4780,6.5);
#4114=CYLINDRICAL_SURFACE('',#4782,4.);
#4115=CYLINDRICAL_SURFACE('',#4784,31.);
#4116=CYLINDRICAL_SURFACE('',#4786,4.);
#4117=CYLINDRICAL_SURFACE('',#4788,6.5);
#4118=CYLINDRICAL_SURFACE('',#4790,4.);
#4119=CYLINDRICAL_SURFACE('',#4792,31.);
#4120=CYLINDRICAL_SURFACE('',#4914,4.);
#4121=CYLINDRICAL_SURFACE('',#4915,31.);
#4122=CYLINDRICAL_SURFACE('',#4916,6.5);
#4123=CYLINDRICAL_SURFACE('',#4917,4.);
#4124=CYLINDRICAL_SURFACE('',#4918,31.);
#4125=CYLINDRICAL_SURFACE('',#4919,4.);
#4126=CYLINDRICAL_SURFACE('',#4920,6.5);
#4127=CYLINDRICAL_SURFACE('',#4921,4.);
#4128=CYLINDRICAL_SURFACE('',#4922,31.);
#4129=CYLINDRICAL_SURFACE('',#4923,4.);
#4130=CYLINDRICAL_SURFACE('',#4924,6.5);
#4131=CYLINDRICAL_SURFACE('',#4925,4.);
#4132=CYLINDRICAL_SURFACE('',#4926,31.);
#4133=CYLINDRICAL_SURFACE('',#4927,4.);
#4134=CYLINDRICAL_SURFACE('',#4942,28.);
#4135=CYLINDRICAL_SURFACE('',#4947,6.5);
#4136=CYLINDRICAL_SURFACE('',#4948,1.5);
#4137=CYLINDRICAL_SURFACE('',#4949,1.5);
#4138=CYLINDRICAL_SURFACE('',#4950,1.5);
#4139=CYLINDRICAL_SURFACE('',#4951,1.5);
#4140=CYLINDRICAL_SURFACE('',#4952,1.5);
#4141=CYLINDRICAL_SURFACE('',#4953,1.5);
#4142=CYLINDRICAL_SURFACE('',#4954,1.5);
#4143=CYLINDRICAL_SURFACE('',#4955,1.5);
#4232=ADVANCED_FACE('',(#597),#4086,.F.);
#4233=ADVANCED_FACE('',(#598),#4087,.F.);
#4234=ADVANCED_FACE('',(#599),#4088,.F.);
#4235=ADVANCED_FACE('',(#600),#4089,.F.);
#4236=ADVANCED_FACE('',(#601),#4090,.F.);
#4237=ADVANCED_FACE('',(#602),#4091,.F.);
#4238=ADVANCED_FACE('',(#603),#4092,.F.);
#4239=ADVANCED_FACE('',(#604),#4093,.F.);
#4240=ADVANCED_FACE('',(#605),#4094,.F.);
#4241=ADVANCED_FACE('',(#606),#4095,.F.);
#4242=ADVANCED_FACE('',(#607),#4096,.F.);
#4243=ADVANCED_FACE('',(#608),#55,.F.);
#4244=ADVANCED_FACE('',(#609),#56,.F.);
#4245=ADVANCED_FACE('',(#610,#102),#143,.T.);
#4246=ADVANCED_FACE('',(#611),#4097,.T.);
#4247=ADVANCED_FACE('',(#612,#103),#144,.F.);
#4248=ADVANCED_FACE('',(#613),#4098,.F.);
#4249=ADVANCED_FACE('',(#614),#4099,.F.);
#4250=ADVANCED_FACE('',(#615),#4100,.F.);
#4251=ADVANCED_FACE('',(#616),#4101,.F.);
#4252=ADVANCED_FACE('',(#617),#4102,.T.);
#4253=ADVANCED_FACE('',(#618),#4103,.F.);
#4254=ADVANCED_FACE('',(#619),#4104,.T.);
#4255=ADVANCED_FACE('',(#620),#450,.T.);
#4256=ADVANCED_FACE('',(#621),#451,.T.);
#4257=ADVANCED_FACE('',(#622),#452,.T.);
#4258=ADVANCED_FACE('',(#623),#453,.T.);
#4259=ADVANCED_FACE('',(#624),#454,.T.);
#4260=ADVANCED_FACE('',(#625),#455,.T.);
#4261=ADVANCED_FACE('',(#626),#456,.T.);
#4262=ADVANCED_FACE('',(#627),#457,.T.);
#4263=ADVANCED_FACE('',(#628),#458,.T.);
#4264=ADVANCED_FACE('',(#629),#459,.T.);
#4265=ADVANCED_FACE('',(#630),#460,.T.);
#4266=ADVANCED_FACE('',(#631),#461,.T.);
#4267=ADVANCED_FACE('',(#632),#462,.T.);
#4268=ADVANCED_FACE('',(#633),#463,.T.);
#4269=ADVANCED_FACE('',(#634),#464,.T.);
#4270=ADVANCED_FACE('',(#635),#465,.T.);
#4271=ADVANCED_FACE('',(#636),#466,.T.);
#4272=ADVANCED_FACE('',(#637),#467,.T.);
#4273=ADVANCED_FACE('',(#638),#468,.T.);
#4274=ADVANCED_FACE('',(#639),#469,.T.);
#4275=ADVANCED_FACE('',(#640),#470,.T.);
#4276=ADVANCED_FACE('',(#641),#471,.T.);
#4277=ADVANCED_FACE('',(#642),#472,.T.);
#4278=ADVANCED_FACE('',(#643),#473,.T.);
#4279=ADVANCED_FACE('',(#644),#474,.T.);
#4280=ADVANCED_FACE('',(#645),#475,.T.);
#4281=ADVANCED_FACE('',(#646),#476,.T.);
#4282=ADVANCED_FACE('',(#647),#477,.T.);
#4283=ADVANCED_FACE('',(#648),#478,.T.);
#4284=ADVANCED_FACE('',(#649),#479,.T.);
#4285=ADVANCED_FACE('',(#650),#480,.T.);
#4286=ADVANCED_FACE('',(#651),#481,.T.);
#4287=ADVANCED_FACE('',(#652),#4105,.T.);
#4288=ADVANCED_FACE('',(#653),#4106,.F.);
#4289=ADVANCED_FACE('',(#654),#4107,.T.);
#4290=ADVANCED_FACE('',(#655),#4108,.F.);
#4291=ADVANCED_FACE('',(#656),#4109,.T.);
#4292=ADVANCED_FACE('',(#657),#4110,.F.);
#4293=ADVANCED_FACE('',(#658),#4111,.T.);
#4294=ADVANCED_FACE('',(#659),#4112,.F.);
#4295=ADVANCED_FACE('',(#660),#4113,.T.);
#4296=ADVANCED_FACE('',(#661),#4114,.F.);
#4297=ADVANCED_FACE('',(#662),#4115,.T.);
#4298=ADVANCED_FACE('',(#663),#4116,.F.);
#4299=ADVANCED_FACE('',(#664),#4117,.T.);
#4300=ADVANCED_FACE('',(#665),#4118,.F.);
#4301=ADVANCED_FACE('',(#666),#4119,.T.);
#4302=ADVANCED_FACE('',(#667,#104,#105,#106,#107,#108,#109,#110,#111,#112),
#145,.T.);
#4303=ADVANCED_FACE('',(#668),#482,.T.);
#4304=ADVANCED_FACE('',(#669),#483,.T.);
#4305=ADVANCED_FACE('',(#670),#484,.T.);
#4306=ADVANCED_FACE('',(#671),#485,.T.);
#4307=ADVANCED_FACE('',(#672),#486,.T.);
#4308=ADVANCED_FACE('',(#673),#487,.T.);
#4309=ADVANCED_FACE('',(#674),#488,.T.);
#4310=ADVANCED_FACE('',(#675),#489,.T.);
#4311=ADVANCED_FACE('',(#676),#490,.T.);
#4312=ADVANCED_FACE('',(#677),#491,.T.);
#4313=ADVANCED_FACE('',(#678),#492,.T.);
#4314=ADVANCED_FACE('',(#679),#493,.T.);
#4315=ADVANCED_FACE('',(#680),#494,.T.);
#4316=ADVANCED_FACE('',(#681),#495,.T.);
#4317=ADVANCED_FACE('',(#682),#496,.T.);
#4318=ADVANCED_FACE('',(#683),#497,.T.);
#4319=ADVANCED_FACE('',(#684),#498,.T.);
#4320=ADVANCED_FACE('',(#685),#499,.T.);
#4321=ADVANCED_FACE('',(#686),#500,.T.);
#4322=ADVANCED_FACE('',(#687),#501,.T.);
#4323=ADVANCED_FACE('',(#688),#502,.T.);
#4324=ADVANCED_FACE('',(#689),#503,.T.);
#4325=ADVANCED_FACE('',(#690),#504,.T.);
#4326=ADVANCED_FACE('',(#691),#505,.T.);
#4327=ADVANCED_FACE('',(#692),#506,.T.);
#4328=ADVANCED_FACE('',(#693),#507,.T.);
#4329=ADVANCED_FACE('',(#694),#508,.T.);
#4330=ADVANCED_FACE('',(#695),#509,.T.);
#4331=ADVANCED_FACE('',(#696),#510,.T.);
#4332=ADVANCED_FACE('',(#697),#511,.T.);
#4333=ADVANCED_FACE('',(#698),#512,.T.);
#4334=ADVANCED_FACE('',(#699),#513,.T.);
#4335=ADVANCED_FACE('',(#700),#4120,.F.);
#4336=ADVANCED_FACE('',(#701),#4121,.T.);
#4337=ADVANCED_FACE('',(#702),#4122,.T.);
#4338=ADVANCED_FACE('',(#703),#4123,.F.);
#4339=ADVANCED_FACE('',(#704),#4124,.T.);
#4340=ADVANCED_FACE('',(#705),#4125,.F.);
#4341=ADVANCED_FACE('',(#706),#4126,.T.);
#4342=ADVANCED_FACE('',(#707),#4127,.F.);
#4343=ADVANCED_FACE('',(#708),#4128,.T.);
#4344=ADVANCED_FACE('',(#709),#4129,.F.);
#4345=ADVANCED_FACE('',(#710),#4130,.T.);
#4346=ADVANCED_FACE('',(#711),#4131,.F.);
#4347=ADVANCED_FACE('',(#712),#4132,.T.);
#4348=ADVANCED_FACE('',(#713),#4133,.F.);
#4349=ADVANCED_FACE('',(#714,#113,#114,#115,#116,#117,#118,#119,#120,#121),
#146,.F.);
#4350=ADVANCED_FACE('',(#715),#514,.T.);
#4351=ADVANCED_FACE('',(#716,#122,#123),#4134,.F.);
#4352=ADVANCED_FACE('',(#717),#515,.T.);
#4353=ADVANCED_FACE('',(#718),#4135,.T.);
#4354=ADVANCED_FACE('',(#719),#4136,.F.);
#4355=ADVANCED_FACE('',(#720),#4137,.F.);
#4356=ADVANCED_FACE('',(#721),#4138,.F.);
#4357=ADVANCED_FACE('',(#722),#4139,.F.);
#4358=ADVANCED_FACE('',(#723),#4140,.F.);
#4359=ADVANCED_FACE('',(#724),#4141,.F.);
#4360=ADVANCED_FACE('',(#725),#4142,.F.);
#4361=ADVANCED_FACE('',(#726),#4143,.F.);
#4388=CLOSED_SHELL('',(#4232,#4233,#4234,#4235,#4236,#4237,#4238,#4239,
#4240,#4241,#4242,#4243,#4244,#4245,#4246,#4247,#4248,#4249,#4250,#4251,
#4252,#4253,#4254,#4255,#4256,#4257,#4258,#4259,#4260,#4261,#4262,#4263,
#4264,#4265,#4266,#4267,#4268,#4269,#4270,#4271,#4272,#4273,#4274,#4275,
#4276,#4277,#4278,#4279,#4280,#4281,#4282,#4283,#4284,#4285,#4286,#4287,
#4288,#4289,#4290,#4291,#4292,#4293,#4294,#4295,#4296,#4297,#4298,#4299,
#4300,#4301,#4302,#4303,#4304,#4305,#4306,#4307,#4308,#4309,#4310,#4311,
#4312,#4313,#4314,#4315,#4316,#4317,#4318,#4319,#4320,#4321,#4322,#4323,
#4324,#4325,#4326,#4327,#4328,#4329,#4330,#4331,#4332,#4333,#4334,#4335,
#4336,#4337,#4338,#4339,#4340,#4341,#4342,#4343,#4344,#4345,#4346,#4347,
#4348,#4349,#4350,#4351,#4352,#4353,#4354,#4355,#4356,#4357,#4358,#4359,
#4360,#4361));
#4604=AXIS2_PLACEMENT_3D('',#26042,#5307,#5308);
#4605=AXIS2_PLACEMENT_3D('',#26043,#5309,#5310);
#4606=AXIS2_PLACEMENT_3D('',#26053,#5312,#5313);
#4607=AXIS2_PLACEMENT_3D('',#26109,#5314,#5315);
#4608=AXIS2_PLACEMENT_3D('',#26500,#5317,#5318);
#4609=AXIS2_PLACEMENT_3D('',#26966,#5320,#5321);
#4610=AXIS2_PLACEMENT_3D('',#27432,#5323,#5324);
#4611=AXIS2_PLACEMENT_3D('',#27752,#5326,#5327);
#4612=AXIS2_PLACEMENT_3D('',#28142,#5329,#5330);
#4613=AXIS2_PLACEMENT_3D('',#28608,#5332,#5333);
#4614=AXIS2_PLACEMENT_3D('',#29074,#5335,#5336);
#4615=AXIS2_PLACEMENT_3D('',#29168,#5338,#5339);
#4616=AXIS2_PLACEMENT_3D('',#29319,#5340,#5341);
#4617=AXIS2_PLACEMENT_3D('',#29322,#5342,#5343);
#4618=AXIS2_PLACEMENT_3D('',#30766,#5344,#5345);
#4619=AXIS2_PLACEMENT_3D('',#32200,#5346,#5347);
#4620=AXIS2_PLACEMENT_3D('',#33524,#5348,#5349);
#4621=AXIS2_PLACEMENT_3D('',#33527,#5350,#5351);
#4622=AXIS2_PLACEMENT_3D('',#33528,#5352,#5353);
#4623=AXIS2_PLACEMENT_3D('',#33529,#5354,#5355);
#4624=AXIS2_PLACEMENT_3D('',#33531,#5356,#5357);
#4625=AXIS2_PLACEMENT_3D('',#33588,#5359,#5360);
#4626=AXIS2_PLACEMENT_3D('',#33589,#5361,#5362);
#4627=AXIS2_PLACEMENT_3D('',#33608,#5363,#5364);
#4628=AXIS2_PLACEMENT_3D('',#33628,#5365,#5366);
#4629=AXIS2_PLACEMENT_3D('',#33720,#5368,#5369);
#4630=AXIS2_PLACEMENT_3D('',#33724,#5371,#5372);
#4631=AXIS2_PLACEMENT_3D('',#33728,#5374,#5375);
#4632=AXIS2_PLACEMENT_3D('',#33730,#5377,#5378);
#4633=AXIS2_PLACEMENT_3D('',#33733,#5380,#5381);
#4634=AXIS2_PLACEMENT_3D('',#33734,#5382,#5383);
#4635=AXIS2_PLACEMENT_3D('',#33738,#5385,#5386);
#4636=AXIS2_PLACEMENT_3D('',#33742,#5388,#5389);
#4637=AXIS2_PLACEMENT_3D('',#33744,#5391,#5392);
#4638=AXIS2_PLACEMENT_3D('',#33747,#5394,#5395);
#4639=AXIS2_PLACEMENT_3D('',#33748,#5396,#5397);
#4640=AXIS2_PLACEMENT_3D('',#33750,#5398,#5399);
#4641=AXIS2_PLACEMENT_3D('',#33752,#5400,#5401);
#4642=AXIS2_PLACEMENT_3D('',#33753,#5402,#5403);
#4643=AXIS2_PLACEMENT_3D('',#33754,#5404,#5405);
#4644=AXIS2_PLACEMENT_3D('',#33757,#5406,#5407);
#4645=AXIS2_PLACEMENT_3D('',#33758,#5408,#5409);
#4646=AXIS2_PLACEMENT_3D('',#33759,#5410,#5411);
#4647=AXIS2_PLACEMENT_3D('',#33760,#5412,#5413);
#4648=AXIS2_PLACEMENT_3D('',#33763,#5414,#5415);
#4649=AXIS2_PLACEMENT_3D('',#33764,#5416,#5417);
#4650=AXIS2_PLACEMENT_3D('',#33765,#5418,#5419);
#4651=AXIS2_PLACEMENT_3D('',#33766,#5420,#5421);
#4652=AXIS2_PLACEMENT_3D('',#33769,#5422,#5423);
#4653=AXIS2_PLACEMENT_3D('',#33770,#5424,#5425);
#4654=AXIS2_PLACEMENT_3D('',#33771,#5426,#5427);
#4655=AXIS2_PLACEMENT_3D('',#33772,#5428,#5429);
#4656=AXIS2_PLACEMENT_3D('',#33775,#5430,#5431);
#4657=AXIS2_PLACEMENT_3D('',#33776,#5432,#5433);
#4658=AXIS2_PLACEMENT_3D('',#33777,#5434,#5435);
#4659=AXIS2_PLACEMENT_3D('',#33778,#5436,#5437);
#4660=AXIS2_PLACEMENT_3D('',#33781,#5438,#5439);
#4661=AXIS2_PLACEMENT_3D('',#33782,#5440,#5441);
#4662=AXIS2_PLACEMENT_3D('',#33783,#5442,#5443);
#4663=AXIS2_PLACEMENT_3D('',#33784,#5444,#5445);
#4664=AXIS2_PLACEMENT_3D('',#33787,#5446,#5447);
#4665=AXIS2_PLACEMENT_3D('',#33788,#5448,#5449);
#4666=AXIS2_PLACEMENT_3D('',#33789,#5450,#5451);
#4667=AXIS2_PLACEMENT_3D('',#33790,#5452,#5453);
#4668=AXIS2_PLACEMENT_3D('',#33793,#5454,#5455);
#4669=AXIS2_PLACEMENT_3D('',#33794,#5456,#5457);
#4670=AXIS2_PLACEMENT_3D('',#33795,#5458,#5459);
#4671=AXIS2_PLACEMENT_3D('',#33796,#5460,#5461);
#4672=AXIS2_PLACEMENT_3D('',#33799,#5462,#5463);
#4673=AXIS2_PLACEMENT_3D('',#33800,#5464,#5465);
#4674=AXIS2_PLACEMENT_3D('',#33801,#5466,#5467);
#4675=AXIS2_PLACEMENT_3D('',#33802,#5468,#5469);
#4676=AXIS2_PLACEMENT_3D('',#33805,#5470,#5471);
#4677=AXIS2_PLACEMENT_3D('',#33806,#5472,#5473);
#4678=AXIS2_PLACEMENT_3D('',#33807,#5474,#5475);
#4679=AXIS2_PLACEMENT_3D('',#33808,#5476,#5477);
#4680=AXIS2_PLACEMENT_3D('',#33811,#5478,#5479);
#4681=AXIS2_PLACEMENT_3D('',#33812,#5480,#5481);
#4682=AXIS2_PLACEMENT_3D('',#33813,#5482,#5483);
#4683=AXIS2_PLACEMENT_3D('',#33814,#5484,#5485);
#4684=AXIS2_PLACEMENT_3D('',#33817,#5486,#5487);
#4685=AXIS2_PLACEMENT_3D('',#33818,#5488,#5489);
#4686=AXIS2_PLACEMENT_3D('',#33819,#5490,#5491);
#4687=AXIS2_PLACEMENT_3D('',#33820,#5492,#5493);
#4688=AXIS2_PLACEMENT_3D('',#33823,#5494,#5495);
#4689=AXIS2_PLACEMENT_3D('',#33824,#5496,#5497);
#4690=AXIS2_PLACEMENT_3D('',#33825,#5498,#5499);
#4691=AXIS2_PLACEMENT_3D('',#33826,#5500,#5501);
#4692=AXIS2_PLACEMENT_3D('',#33828,#5502,#5503);
#4693=AXIS2_PLACEMENT_3D('',#33829,#5504,#5505);
#4694=AXIS2_PLACEMENT_3D('',#33830,#5506,#5507);
#4695=AXIS2_PLACEMENT_3D('',#33831,#5508,#5509);
#4696=AXIS2_PLACEMENT_3D('',#33833,#5510,#5511);
#4697=AXIS2_PLACEMENT_3D('',#33834,#5512,#5513);
#4698=AXIS2_PLACEMENT_3D('',#33835,#5514,#5515);
#4699=AXIS2_PLACEMENT_3D('',#33838,#5516,#5517);
#4700=AXIS2_PLACEMENT_3D('',#33839,#5518,#5519);
#4701=AXIS2_PLACEMENT_3D('',#33840,#5520,#5521);
#4702=AXIS2_PLACEMENT_3D('',#33841,#5522,#5523);
#4703=AXIS2_PLACEMENT_3D('',#33844,#5524,#5525);
#4704=AXIS2_PLACEMENT_3D('',#33845,#5526,#5527);
#4705=AXIS2_PLACEMENT_3D('',#33846,#5528,#5529);
#4706=AXIS2_PLACEMENT_3D('',#33847,#5530,#5531);
#4707=AXIS2_PLACEMENT_3D('',#33850,#5532,#5533);
#4708=AXIS2_PLACEMENT_3D('',#33851,#5534,#5535);
#4709=AXIS2_PLACEMENT_3D('',#33852,#5536,#5537);
#4710=AXIS2_PLACEMENT_3D('',#33853,#5538,#5539);
#4711=AXIS2_PLACEMENT_3D('',#33856,#5540,#5541);
#4712=AXIS2_PLACEMENT_3D('',#33857,#5542,#5543);
#4713=AXIS2_PLACEMENT_3D('',#33858,#5544,#5545);
#4714=AXIS2_PLACEMENT_3D('',#33859,#5546,#5547);
#4715=AXIS2_PLACEMENT_3D('',#33862,#5548,#5549);
#4716=AXIS2_PLACEMENT_3D('',#33863,#5550,#5551);
#4717=AXIS2_PLACEMENT_3D('',#33864,#5552,#5553);
#4718=AXIS2_PLACEMENT_3D('',#33865,#5554,#5555);
#4719=AXIS2_PLACEMENT_3D('',#33868,#5556,#5557);
#4720=AXIS2_PLACEMENT_3D('',#33869,#5558,#5559);
#4721=AXIS2_PLACEMENT_3D('',#33870,#5560,#5561);
#4722=AXIS2_PLACEMENT_3D('',#33871,#5562,#5563);
#4723=AXIS2_PLACEMENT_3D('',#33874,#5564,#5565);
#4724=AXIS2_PLACEMENT_3D('',#33875,#5566,#5567);
#4725=AXIS2_PLACEMENT_3D('',#33876,#5568,#5569);
#4726=AXIS2_PLACEMENT_3D('',#33877,#5570,#5571);
#4727=AXIS2_PLACEMENT_3D('',#33880,#5572,#5573);
#4728=AXIS2_PLACEMENT_3D('',#33881,#5574,#5575);
#4729=AXIS2_PLACEMENT_3D('',#33882,#5576,#5577);
#4730=AXIS2_PLACEMENT_3D('',#33883,#5578,#5579);
#4731=AXIS2_PLACEMENT_3D('',#33886,#5580,#5581);
#4732=AXIS2_PLACEMENT_3D('',#33887,#5582,#5583);
#4733=AXIS2_PLACEMENT_3D('',#33888,#5584,#5585);
#4734=AXIS2_PLACEMENT_3D('',#33889,#5586,#5587);
#4735=AXIS2_PLACEMENT_3D('',#33892,#5588,#5589);
#4736=AXIS2_PLACEMENT_3D('',#33893,#5590,#5591);
#4737=AXIS2_PLACEMENT_3D('',#33894,#5592,#5593);
#4738=AXIS2_PLACEMENT_3D('',#33895,#5594,#5595);
#4739=AXIS2_PLACEMENT_3D('',#33898,#5596,#5597);
#4740=AXIS2_PLACEMENT_3D('',#33899,#5598,#5599);
#4741=AXIS2_PLACEMENT_3D('',#33900,#5600,#5601);
#4742=AXIS2_PLACEMENT_3D('',#33901,#5602,#5603);
#4743=AXIS2_PLACEMENT_3D('',#33904,#5604,#5605);
#4744=AXIS2_PLACEMENT_3D('',#33905,#5606,#5607);
#4745=AXIS2_PLACEMENT_3D('',#33906,#5608,#5609);
#4746=AXIS2_PLACEMENT_3D('',#33907,#5610,#5611);
#4747=AXIS2_PLACEMENT_3D('',#33910,#5612,#5613);
#4748=AXIS2_PLACEMENT_3D('',#33911,#5614,#5615);
#4749=AXIS2_PLACEMENT_3D('',#33912,#5616,#5617);
#4750=AXIS2_PLACEMENT_3D('',#33913,#5618,#5619);
#4751=AXIS2_PLACEMENT_3D('',#33916,#5620,#5621);
#4752=AXIS2_PLACEMENT_3D('',#33917,#5622,#5623);
#4753=AXIS2_PLACEMENT_3D('',#33918,#5624,#5625);
#4754=AXIS2_PLACEMENT_3D('',#33919,#5626,#5627);
#4755=AXIS2_PLACEMENT_3D('',#33922,#5628,#5629);
#4756=AXIS2_PLACEMENT_3D('',#33923,#5630,#5631);
#4757=AXIS2_PLACEMENT_3D('',#33924,#5632,#5633);
#4758=AXIS2_PLACEMENT_3D('',#33925,#5634,#5635);
#4759=AXIS2_PLACEMENT_3D('',#33927,#5636,#5637);
#4760=AXIS2_PLACEMENT_3D('',#33928,#5638,#5639);
#4761=AXIS2_PLACEMENT_3D('',#33929,#5640,#5641);
#4762=AXIS2_PLACEMENT_3D('',#33930,#5642,#5643);
#4763=AXIS2_PLACEMENT_3D('',#33931,#5644,#5645);
#4764=AXIS2_PLACEMENT_3D('',#33932,#5646,#5647);
#4765=AXIS2_PLACEMENT_3D('',#33936,#5649,#5650);
#4766=AXIS2_PLACEMENT_3D('',#33938,#5652,#5653);
#4767=AXIS2_PLACEMENT_3D('',#33941,#5655,#5656);
#4768=AXIS2_PLACEMENT_3D('',#33942,#5657,#5658);
#4769=AXIS2_PLACEMENT_3D('',#33945,#5660,#5661);
#4770=AXIS2_PLACEMENT_3D('',#33946,#5662,#5663);
#4771=AXIS2_PLACEMENT_3D('',#33949,#5665,#5666);
#4772=AXIS2_PLACEMENT_3D('',#33950,#5667,#5668);
#4773=AXIS2_PLACEMENT_3D('',#33953,#5670,#5671);
#4774=AXIS2_PLACEMENT_3D('',#33954,#5672,#5673);
#4775=AXIS2_PLACEMENT_3D('',#33957,#5675,#5676);
#4776=AXIS2_PLACEMENT_3D('',#33958,#5677,#5678);
#4777=AXIS2_PLACEMENT_3D('',#33961,#5680,#5681);
#4778=AXIS2_PLACEMENT_3D('',#33962,#5682,#5683);
#4779=AXIS2_PLACEMENT_3D('',#33965,#5685,#5686);
#4780=AXIS2_PLACEMENT_3D('',#33966,#5687,#5688);
#4781=AXIS2_PLACEMENT_3D('',#33969,#5690,#5691);
#4782=AXIS2_PLACEMENT_3D('',#33970,#5692,#5693);
#4783=AXIS2_PLACEMENT_3D('',#33973,#5695,#5696);
#4784=AXIS2_PLACEMENT_3D('',#33974,#5697,#5698);
#4785=AXIS2_PLACEMENT_3D('',#33977,#5700,#5701);
#4786=AXIS2_PLACEMENT_3D('',#33978,#5702,#5703);
#4787=AXIS2_PLACEMENT_3D('',#33981,#5705,#5706);
#4788=AXIS2_PLACEMENT_3D('',#33982,#5707,#5708);
#4789=AXIS2_PLACEMENT_3D('',#33985,#5710,#5711);
#4790=AXIS2_PLACEMENT_3D('',#33986,#5712,#5713);
#4791=AXIS2_PLACEMENT_3D('',#33989,#5715,#5716);
#4792=AXIS2_PLACEMENT_3D('',#33990,#5717,#5718);
#4793=AXIS2_PLACEMENT_3D('',#33991,#5719,#5720);
#4794=AXIS2_PLACEMENT_3D('',#33992,#5721,#5722);
#4795=AXIS2_PLACEMENT_3D('',#33994,#5723,#5724);
#4796=AXIS2_PLACEMENT_3D('',#33996,#5725,#5726);
#4797=AXIS2_PLACEMENT_3D('',#33998,#5727,#5728);
#4798=AXIS2_PLACEMENT_3D('',#34000,#5729,#5730);
#4799=AXIS2_PLACEMENT_3D('',#34002,#5731,#5732);
#4800=AXIS2_PLACEMENT_3D('',#34004,#5733,#5734);
#4801=AXIS2_PLACEMENT_3D('',#34006,#5735,#5736);
#4802=AXIS2_PLACEMENT_3D('',#34008,#5737,#5738);
#4803=AXIS2_PLACEMENT_3D('',#34010,#5739,#5740);
#4804=AXIS2_PLACEMENT_3D('',#34011,#5741,#5742);
#4805=AXIS2_PLACEMENT_3D('',#34014,#5743,#5744);
#4806=AXIS2_PLACEMENT_3D('',#34016,#5745,#5746);
#4807=AXIS2_PLACEMENT_3D('',#34018,#5747,#5748);
#4808=AXIS2_PLACEMENT_3D('',#34019,#5749,#5750);
#4809=AXIS2_PLACEMENT_3D('',#34020,#5751,#5752);
#4810=AXIS2_PLACEMENT_3D('',#34022,#5753,#5754);
#4811=AXIS2_PLACEMENT_3D('',#34023,#5755,#5756);
#4812=AXIS2_PLACEMENT_3D('',#34024,#5757,#5758);
#4813=AXIS2_PLACEMENT_3D('',#34025,#5759,#5760);
#4814=AXIS2_PLACEMENT_3D('',#34027,#5761,#5762);
#4815=AXIS2_PLACEMENT_3D('',#34028,#5763,#5764);
#4816=AXIS2_PLACEMENT_3D('',#34029,#5765,#5766);
#4817=AXIS2_PLACEMENT_3D('',#34031,#5767,#5768);
#4818=AXIS2_PLACEMENT_3D('',#34032,#5769,#5770);
#4819=AXIS2_PLACEMENT_3D('',#34033,#5771,#5772);
#4820=AXIS2_PLACEMENT_3D('',#34035,#5773,#5774);
#4821=AXIS2_PLACEMENT_3D('',#34036,#5775,#5776);
#4822=AXIS2_PLACEMENT_3D('',#34037,#5777,#5778);
#4823=AXIS2_PLACEMENT_3D('',#34039,#5779,#5780);
#4824=AXIS2_PLACEMENT_3D('',#34040,#5781,#5782);
#4825=AXIS2_PLACEMENT_3D('',#34041,#5783,#5784);
#4826=AXIS2_PLACEMENT_3D('',#34043,#5785,#5786);
#4827=AXIS2_PLACEMENT_3D('',#34044,#5787,#5788);
#4828=AXIS2_PLACEMENT_3D('',#34045,#5789,#5790);
#4829=AXIS2_PLACEMENT_3D('',#34047,#5791,#5792);
#4830=AXIS2_PLACEMENT_3D('',#34048,#5793,#5794);
#4831=AXIS2_PLACEMENT_3D('',#34049,#5795,#5796);
#4832=AXIS2_PLACEMENT_3D('',#34051,#5797,#5798);
#4833=AXIS2_PLACEMENT_3D('',#34052,#5799,#5800);
#4834=AXIS2_PLACEMENT_3D('',#34053,#5801,#5802);
#4835=AXIS2_PLACEMENT_3D('',#34055,#5803,#5804);
#4836=AXIS2_PLACEMENT_3D('',#34056,#5805,#5806);
#4837=AXIS2_PLACEMENT_3D('',#34057,#5807,#5808);
#4838=AXIS2_PLACEMENT_3D('',#34059,#5809,#5810);
#4839=AXIS2_PLACEMENT_3D('',#34060,#5811,#5812);
#4840=AXIS2_PLACEMENT_3D('',#34061,#5813,#5814);
#4841=AXIS2_PLACEMENT_3D('',#34063,#5815,#5816);
#4842=AXIS2_PLACEMENT_3D('',#34064,#5817,#5818);
#4843=AXIS2_PLACEMENT_3D('',#34065,#5819,#5820);
#4844=AXIS2_PLACEMENT_3D('',#34067,#5821,#5822);
#4845=AXIS2_PLACEMENT_3D('',#34068,#5823,#5824);
#4846=AXIS2_PLACEMENT_3D('',#34069,#5825,#5826);
#4847=AXIS2_PLACEMENT_3D('',#34071,#5827,#5828);
#4848=AXIS2_PLACEMENT_3D('',#34072,#5829,#5830);
#4849=AXIS2_PLACEMENT_3D('',#34073,#5831,#5832);
#4850=AXIS2_PLACEMENT_3D('',#34075,#5833,#5834);
#4851=AXIS2_PLACEMENT_3D('',#34076,#5835,#5836);
#4852=AXIS2_PLACEMENT_3D('',#34077,#5837,#5838);
#4853=AXIS2_PLACEMENT_3D('',#34079,#5839,#5840);
#4854=AXIS2_PLACEMENT_3D('',#34080,#5841,#5842);
#4855=AXIS2_PLACEMENT_3D('',#34081,#5843,#5844);
#4856=AXIS2_PLACEMENT_3D('',#34083,#5845,#5846);
#4857=AXIS2_PLACEMENT_3D('',#34084,#5847,#5848);
#4858=AXIS2_PLACEMENT_3D('',#34085,#5849,#5850);
#4859=AXIS2_PLACEMENT_3D('',#34087,#5851,#5852);
#4860=AXIS2_PLACEMENT_3D('',#34088,#5853,#5854);
#4861=AXIS2_PLACEMENT_3D('',#34089,#5855,#5856);
#4862=AXIS2_PLACEMENT_3D('',#34091,#5857,#5858);
#4863=AXIS2_PLACEMENT_3D('',#34092,#5859,#5860);
#4864=AXIS2_PLACEMENT_3D('',#34093,#5861,#5862);
#4865=AXIS2_PLACEMENT_3D('',#34094,#5863,#5864);
#4866=AXIS2_PLACEMENT_3D('',#34096,#5865,#5866);
#4867=AXIS2_PLACEMENT_3D('',#34097,#5867,#5868);
#4868=AXIS2_PLACEMENT_3D('',#34098,#5869,#5870);
#4869=AXIS2_PLACEMENT_3D('',#34100,#5871,#5872);
#4870=AXIS2_PLACEMENT_3D('',#34101,#5873,#5874);
#4871=AXIS2_PLACEMENT_3D('',#34102,#5875,#5876);
#4872=AXIS2_PLACEMENT_3D('',#34105,#5877,#5878);
#4873=AXIS2_PLACEMENT_3D('',#34106,#5879,#5880);
#4874=AXIS2_PLACEMENT_3D('',#34107,#5881,#5882);
#4875=AXIS2_PLACEMENT_3D('',#34108,#5883,#5884);
#4876=AXIS2_PLACEMENT_3D('',#34111,#5885,#5886);
#4877=AXIS2_PLACEMENT_3D('',#34112,#5887,#5888);
#4878=AXIS2_PLACEMENT_3D('',#34113,#5889,#5890);
#4879=AXIS2_PLACEMENT_3D('',#34114,#5891,#5892);
#4880=AXIS2_PLACEMENT_3D('',#34117,#5893,#5894);
#4881=AXIS2_PLACEMENT_3D('',#34118,#5895,#5896);
#4882=AXIS2_PLACEMENT_3D('',#34119,#5897,#5898);
#4883=AXIS2_PLACEMENT_3D('',#34120,#5899,#5900);
#4884=AXIS2_PLACEMENT_3D('',#34123,#5901,#5902);
#4885=AXIS2_PLACEMENT_3D('',#34124,#5903,#5904);
#4886=AXIS2_PLACEMENT_3D('',#34125,#5905,#5906);
#4887=AXIS2_PLACEMENT_3D('',#34126,#5907,#5908);
#4888=AXIS2_PLACEMENT_3D('',#34129,#5909,#5910);
#4889=AXIS2_PLACEMENT_3D('',#34130,#5911,#5912);
#4890=AXIS2_PLACEMENT_3D('',#34131,#5913,#5914);
#4891=AXIS2_PLACEMENT_3D('',#34132,#5915,#5916);
#4892=AXIS2_PLACEMENT_3D('',#34135,#5917,#5918);
#4893=AXIS2_PLACEMENT_3D('',#34136,#5919,#5920);
#4894=AXIS2_PLACEMENT_3D('',#34137,#5921,#5922);
#4895=AXIS2_PLACEMENT_3D('',#34138,#5923,#5924);
#4896=AXIS2_PLACEMENT_3D('',#34141,#5925,#5926);
#4897=AXIS2_PLACEMENT_3D('',#34142,#5927,#5928);
#4898=AXIS2_PLACEMENT_3D('',#34143,#5929,#5930);
#4899=AXIS2_PLACEMENT_3D('',#34144,#5931,#5932);
#4900=AXIS2_PLACEMENT_3D('',#34147,#5933,#5934);
#4901=AXIS2_PLACEMENT_3D('',#34148,#5935,#5936);
#4902=AXIS2_PLACEMENT_3D('',#34149,#5937,#5938);
#4903=AXIS2_PLACEMENT_3D('',#34150,#5939,#5940);
#4904=AXIS2_PLACEMENT_3D('',#34153,#5941,#5942);
#4905=AXIS2_PLACEMENT_3D('',#34154,#5943,#5944);
#4906=AXIS2_PLACEMENT_3D('',#34155,#5945,#5946);
#4907=AXIS2_PLACEMENT_3D('',#34156,#5947,#5948);
#4908=AXIS2_PLACEMENT_3D('',#34159,#5949,#5950);
#4909=AXIS2_PLACEMENT_3D('',#34160,#5951,#5952);
#4910=AXIS2_PLACEMENT_3D('',#34161,#5953,#5954);
#4911=AXIS2_PLACEMENT_3D('',#34162,#5955,#5956);
#4912=AXIS2_PLACEMENT_3D('',#34163,#5957,#5958);
#4913=AXIS2_PLACEMENT_3D('',#34164,#5959,#5960);
#4914=AXIS2_PLACEMENT_3D('',#34165,#5961,#5962);
#4915=AXIS2_PLACEMENT_3D('',#34167,#5964,#5965);
#4916=AXIS2_PLACEMENT_3D('',#34168,#5966,#5967);
#4917=AXIS2_PLACEMENT_3D('',#34170,#5969,#5970);
#4918=AXIS2_PLACEMENT_3D('',#34172,#5972,#5973);
#4919=AXIS2_PLACEMENT_3D('',#34174,#5975,#5976);
#4920=AXIS2_PLACEMENT_3D('',#34176,#5978,#5979);
#4921=AXIS2_PLACEMENT_3D('',#34178,#5981,#5982);
#4922=AXIS2_PLACEMENT_3D('',#34180,#5984,#5985);
#4923=AXIS2_PLACEMENT_3D('',#34182,#5987,#5988);
#4924=AXIS2_PLACEMENT_3D('',#34184,#5990,#5991);
#4925=AXIS2_PLACEMENT_3D('',#34186,#5993,#5994);
#4926=AXIS2_PLACEMENT_3D('',#34188,#5996,#5997);
#4927=AXIS2_PLACEMENT_3D('',#34190,#5999,#6000);
#4928=AXIS2_PLACEMENT_3D('',#34192,#6002,#6003);
#4929=AXIS2_PLACEMENT_3D('',#34194,#6004,#6005);
#4930=AXIS2_PLACEMENT_3D('',#34196,#6006,#6007);
#4931=AXIS2_PLACEMENT_3D('',#34198,#6008,#6009);
#4932=AXIS2_PLACEMENT_3D('',#34200,#6010,#6011);
#4933=AXIS2_PLACEMENT_3D('',#34202,#6012,#6013);
#4934=AXIS2_PLACEMENT_3D('',#34204,#6014,#6015);
#4935=AXIS2_PLACEMENT_3D('',#34206,#6016,#6017);
#4936=AXIS2_PLACEMENT_3D('',#34208,#6018,#6019);
#4937=AXIS2_PLACEMENT_3D('',#34210,#6020,#6021);
#4938=AXIS2_PLACEMENT_3D('',#34211,#6022,#6023);
#4939=AXIS2_PLACEMENT_3D('',#34213,#6024,#6025);
#4940=AXIS2_PLACEMENT_3D('',#34215,#6026,#6027);
#4941=AXIS2_PLACEMENT_3D('',#34216,#6028,#6029);
#4942=AXIS2_PLACEMENT_3D('',#34217,#6030,#6031);
#4943=AXIS2_PLACEMENT_3D('',#34221,#6033,#6034);
#4944=AXIS2_PLACEMENT_3D('',#34222,#6035,#6036);
#4945=AXIS2_PLACEMENT_3D('',#34223,#6037,#6038);
#4946=AXIS2_PLACEMENT_3D('',#34224,#6039,#6040);
#4947=AXIS2_PLACEMENT_3D('',#34225,#6041,#6042);
#4948=AXIS2_PLACEMENT_3D('',#34226,#6043,#6044);
#4949=AXIS2_PLACEMENT_3D('',#34228,#6046,#6047);
#4950=AXIS2_PLACEMENT_3D('',#34230,#6049,#6050);
#4951=AXIS2_PLACEMENT_3D('',#34232,#6052,#6053);
#4952=AXIS2_PLACEMENT_3D('',#34234,#6055,#6056);
#4953=AXIS2_PLACEMENT_3D('',#34236,#6058,#6059);
#4954=AXIS2_PLACEMENT_3D('',#34238,#6061,#6062);
#4955=AXIS2_PLACEMENT_3D('',#34240,#6064,#6065);
#5307=DIRECTION('axis',(0.,0.,1.));
#5308=DIRECTION('refdir',(1.,0.,0.));
#5309=DIRECTION('center_axis',(0.,0.,-1.));
#5310=DIRECTION('ref_axis',(-0.608826750567588,-0.793303213023439,0.));
#5311=DIRECTION('',(0.,0.,-1.));
#5312=DIRECTION('center_axis',(0.,0.,1.));
#5313=DIRECTION('ref_axis',(1.,-1.81309624337467E-14,0.));
#5314=DIRECTION('center_axis',(0.,0.,-1.));
#5315=DIRECTION('ref_axis',(-0.608826750567588,-0.793303213023439,0.));
#5316=DIRECTION('',(0.,0.,-1.));
#5317=DIRECTION('center_axis',(0.,0.,-1.));
#5318=DIRECTION('ref_axis',(-0.608826750567588,-0.793303213023439,0.));
#5319=DIRECTION('',(0.,0.,-1.));
#5320=DIRECTION('center_axis',(0.,0.,-1.));
#5321=DIRECTION('ref_axis',(-0.608826750567588,-0.793303213023439,0.));
#5322=DIRECTION('',(0.,0.,-1.));
#5323=DIRECTION('center_axis',(0.,0.,-1.));
#5324=DIRECTION('ref_axis',(-0.608826750567588,-0.793303213023439,0.));
#5325=DIRECTION('',(0.,0.,-1.));
#5326=DIRECTION('center_axis',(0.,0.,-1.));
#5327=DIRECTION('ref_axis',(-0.608826750567588,-0.793303213023439,0.));
#5328=DIRECTION('',(0.,0.,-1.));
#5329=DIRECTION('center_axis',(0.,0.,-1.));
#5330=DIRECTION('ref_axis',(-0.608826750567588,-0.793303213023439,0.));
#5331=DIRECTION('',(0.,0.,-1.));
#5332=DIRECTION('center_axis',(0.,0.,-1.));
#5333=DIRECTION('ref_axis',(-0.608826750567588,-0.793303213023439,0.));
#5334=DIRECTION('',(0.,0.,-1.));
#5335=DIRECTION('center_axis',(0.,0.,-1.));
#5336=DIRECTION('ref_axis',(-0.608826750567588,-0.793303213023439,0.));
#5337=DIRECTION('',(0.,0.,-1.));
#5338=DIRECTION('center_axis',(0.,0.,-1.));
#5339=DIRECTION('ref_axis',(1.,-1.81309624337467E-14,0.));
#5340=DIRECTION('center_axis',(0.,0.,-1.));
#5341=DIRECTION('ref_axis',(1.,0.,0.));
#5342=DIRECTION('center_axis',(0.,0.,1.));
#5343=DIRECTION('ref_axis',(1.,0.,0.));
#5344=DIRECTION('center_axis',(0.,0.,1.));
#5345=DIRECTION('ref_axis',(1.,0.,0.));
#5346=DIRECTION('center_axis',(0.,0.,-1.));
#5347=DIRECTION('ref_axis',(-0.608826750567588,-0.793303213023439,0.));
#5348=DIRECTION('center_axis',(0.,0.,1.));
#5349=DIRECTION('ref_axis',(1.,0.,0.));
#5350=DIRECTION('center_axis',(0.,0.,-1.));
#5351=DIRECTION('ref_axis',(1.,0.,0.));
#5352=DIRECTION('center_axis',(0.,0.,-1.));
#5353=DIRECTION('ref_axis',(1.,0.,0.));
#5354=DIRECTION('center_axis',(0.,0.,-1.));
#5355=DIRECTION('ref_axis',(1.,0.,0.));
#5356=DIRECTION('center_axis',(0.,0.,-1.));
#5357=DIRECTION('ref_axis',(1.,0.,0.));
#5358=DIRECTION('',(0.,0.,1.));
#5359=DIRECTION('center_axis',(0.,0.,1.));
#5360=DIRECTION('ref_axis',(1.,0.,0.));
#5361=DIRECTION('center_axis',(0.,0.,1.));
#5362=DIRECTION('ref_axis',(1.,0.,0.));
#5363=DIRECTION('center_axis',(0.,0.,1.));
#5364=DIRECTION('ref_axis',(-1.,1.22464679914735E-16,0.));
#5365=DIRECTION('center_axis',(0.,0.,1.));
#5366=DIRECTION('ref_axis',(1.,0.,0.));
#5367=DIRECTION('',(0.,0.,1.));
#5368=DIRECTION('center_axis',(0.,-1.,0.));
#5369=DIRECTION('ref_axis',(-0.523000124799862,0.,-0.852332604949106));
#5370=DIRECTION('',(0.,1.,0.));
#5371=DIRECTION('center_axis',(0.,-1.,0.));
#5372=DIRECTION('ref_axis',(-0.523000124799863,0.,-0.852332604949106));
#5373=DIRECTION('',(0.,-1.,0.));
#5374=DIRECTION('center_axis',(0.,1.,0.));
#5375=DIRECTION('ref_axis',(-0.523000124799863,0.,-0.852332604949106));
#5376=DIRECTION('',(0.,1.,0.));
#5377=DIRECTION('center_axis',(0.,-1.,0.));
#5378=DIRECTION('ref_axis',(1.,0.,0.));
#5379=DIRECTION('',(0.,-1.,0.));
#5380=DIRECTION('center_axis',(0.,1.,0.));
#5381=DIRECTION('ref_axis',(6.12323399573677E-17,0.,1.));
#5382=DIRECTION('center_axis',(0.,1.,0.));
#5383=DIRECTION('ref_axis',(-0.523000124799863,0.,0.852332604949106));
#5384=DIRECTION('',(0.,-1.,0.));
#5385=DIRECTION('center_axis',(0.,1.,0.));
#5386=DIRECTION('ref_axis',(-0.523000124799863,0.,0.852332604949105));
#5387=DIRECTION('',(0.,1.,0.));
#5388=DIRECTION('center_axis',(0.,-1.,0.));
#5389=DIRECTION('ref_axis',(-0.523000124799863,0.,0.852332604949105));
#5390=DIRECTION('',(0.,-1.,0.));
#5391=DIRECTION('center_axis',(0.,-1.,0.));
#5392=DIRECTION('ref_axis',(1.,0.,0.));
#5393=DIRECTION('',(0.,1.,0.));
#5394=DIRECTION('center_axis',(0.,-1.,0.));
#5395=DIRECTION('ref_axis',(-1.60812264967664E-16,0.,-1.));
#5396=DIRECTION('center_axis',(0.,1.,0.));
#5397=DIRECTION('ref_axis',(-0.523000124799863,0.,-0.852332604949105));
#5398=DIRECTION('center_axis',(-0.996128362168068,0.,-0.0879106710494425));
#5399=DIRECTION('ref_axis',(-0.0879106710494425,0.,0.996128362168068));
#5400=DIRECTION('center_axis',(0.,1.,0.));
#5401=DIRECTION('ref_axis',(-0.523000124799863,0.,-0.852332604949106));
#5402=DIRECTION('center_axis',(0.372812222548027,0.,-0.927906809285717));
#5403=DIRECTION('ref_axis',(0.,1.,0.));
#5404=DIRECTION('center_axis',(0.,1.,0.));
#5405=DIRECTION('ref_axis',(0.,0.,1.));
#5406=DIRECTION('center_axis',(-0.392511146482165,0.,0.919747247828041));
#5407=DIRECTION('ref_axis',(0.,1.,0.));
#5408=DIRECTION('center_axis',(0.,1.,0.));
#5409=DIRECTION('ref_axis',(-0.382683432365091,0.,0.923879532511286));
#5410=DIRECTION('center_axis',(0.,-1.,0.));
#5411=DIRECTION('ref_axis',(-0.382683432365091,0.,0.923879532511286));
#5412=DIRECTION('center_axis',(0.,1.,0.));
#5413=DIRECTION('ref_axis',(0.,0.,1.));
#5414=DIRECTION('center_axis',(0.766531351459009,0.,0.642206888183571));
#5415=DIRECTION('ref_axis',(0.,1.,0.));
#5416=DIRECTION('center_axis',(0.,-1.,0.));
#5417=DIRECTION('ref_axis',(0.972507099593301,0.,-0.232873229978514));
#5418=DIRECTION('center_axis',(0.,1.,0.));
#5419=DIRECTION('ref_axis',(0.972507099593301,0.,-0.232873229978514));
#5420=DIRECTION('center_axis',(0.,1.,0.));
#5421=DIRECTION('ref_axis',(0.,0.,1.));
#5422=DIRECTION('center_axis',(0.642206888183567,0.,0.766531351459012));
#5423=DIRECTION('ref_axis',(0.,1.,0.));
#5424=DIRECTION('center_axis',(0.,1.,0.));
#5425=DIRECTION('ref_axis',(-0.707106781186547,0.,0.707106781186548));
#5426=DIRECTION('center_axis',(0.,-1.,0.));
#5427=DIRECTION('ref_axis',(-0.707106781186547,0.,0.707106781186548));
#5428=DIRECTION('center_axis',(0.,1.,0.));
#5429=DIRECTION('ref_axis',(0.232873229978514,0.,-0.972507099593301));
#5430=DIRECTION('center_axis',(0.919747247828041,0.,-0.392511146482166));
#5431=DIRECTION('ref_axis',(0.,1.,0.));
#5432=DIRECTION('center_axis',(0.,-1.,0.));
#5433=DIRECTION('ref_axis',(0.232873229978513,0.,-0.972507099593301));
#5434=DIRECTION('center_axis',(0.,1.,0.));
#5435=DIRECTION('ref_axis',(0.232873229978513,0.,-0.972507099593301));
#5436=DIRECTION('center_axis',(0.,1.,0.));
#5437=DIRECTION('ref_axis',(0.,0.,1.));
#5438=DIRECTION('center_axis',(-0.927906809285719,0.,0.372812222548022));
#5439=DIRECTION('ref_axis',(0.,1.,0.));
#5440=DIRECTION('center_axis',(0.,1.,0.));
#5441=DIRECTION('ref_axis',(-0.923879532511287,0.,0.382683432365089));
#5442=DIRECTION('center_axis',(0.,-1.,0.));
#5443=DIRECTION('ref_axis',(-0.923879532511287,0.,0.382683432365089));
#5444=DIRECTION('center_axis',(0.,1.,0.));
#5445=DIRECTION('ref_axis',(0.,0.,1.));
#5446=DIRECTION('center_axis',(0.087910671049441,0.,0.996128362168068));
#5447=DIRECTION('ref_axis',(0.,1.,0.));
#5448=DIRECTION('center_axis',(0.,-1.,0.));
#5449=DIRECTION('ref_axis',(0.852332604949105,0.,0.523000124799863));
#5450=DIRECTION('center_axis',(0.,1.,0.));
#5451=DIRECTION('ref_axis',(0.852332604949105,0.,0.523000124799863));
#5452=DIRECTION('center_axis',(0.,1.,0.));
#5453=DIRECTION('ref_axis',(0.,0.,1.));
#5454=DIRECTION('center_axis',(-0.087910671049441,0.,0.996128362168068));
#5455=DIRECTION('ref_axis',(0.,1.,0.));
#5456=DIRECTION('center_axis',(0.,1.,0.));
#5457=DIRECTION('ref_axis',(-1.,0.,1.22464679914735E-16));
#5458=DIRECTION('center_axis',(0.,-1.,0.));
#5459=DIRECTION('ref_axis',(-1.,0.,1.22464679914735E-16));
#5460=DIRECTION('center_axis',(0.,1.,0.));
#5461=DIRECTION('ref_axis',(0.,0.,1.));
#5462=DIRECTION('center_axis',(0.927906809285718,0.,0.372812222548024));
#5463=DIRECTION('ref_axis',(0.,1.,0.));
#5464=DIRECTION('center_axis',(0.,-1.,0.));
#5465=DIRECTION('ref_axis',(0.852332604949105,0.,-0.523000124799863));
#5466=DIRECTION('center_axis',(0.,1.,0.));
#5467=DIRECTION('ref_axis',(0.852332604949105,0.,-0.523000124799863));
#5468=DIRECTION('center_axis',(0.,1.,0.));
#5469=DIRECTION('ref_axis',(-0.923879532511287,0.,-0.38268343236509));
#5470=DIRECTION('center_axis',(-0.919747247828042,0.,-0.392511146482165));
#5471=DIRECTION('ref_axis',(0.,1.,0.));
#5472=DIRECTION('center_axis',(0.,1.,0.));
#5473=DIRECTION('ref_axis',(-0.923879532511287,0.,-0.38268343236509));
#5474=DIRECTION('center_axis',(0.,-1.,0.));
#5475=DIRECTION('ref_axis',(-0.923879532511287,0.,-0.38268343236509));
#5476=DIRECTION('center_axis',(0.,1.,0.));
#5477=DIRECTION('ref_axis',(0.,0.,1.));
#5478=DIRECTION('center_axis',(-0.642206888183571,0.,0.766531351459009));
#5479=DIRECTION('ref_axis',(0.,1.,0.));
#5480=DIRECTION('center_axis',(0.,-1.,0.));
#5481=DIRECTION('ref_axis',(0.232873229978512,0.,0.972507099593301));
#5482=DIRECTION('center_axis',(0.,1.,0.));
#5483=DIRECTION('ref_axis',(0.232873229978512,0.,0.972507099593301));
#5484=DIRECTION('center_axis',(0.,1.,0.));
#5485=DIRECTION('ref_axis',(0.,0.,1.));
#5486=DIRECTION('center_axis',(-0.766531351459001,0.,0.642206888183581));
#5487=DIRECTION('ref_axis',(0.,1.,0.));
#5488=DIRECTION('center_axis',(0.,1.,0.));
#5489=DIRECTION('ref_axis',(-0.707106781186548,0.,-0.707106781186547));
#5490=DIRECTION('center_axis',(0.,-1.,0.));
#5491=DIRECTION('ref_axis',(-0.707106781186548,0.,-0.707106781186547));
#5492=DIRECTION('center_axis',(0.,1.,0.));
#5493=DIRECTION('ref_axis',(0.,0.,1.));
#5494=DIRECTION('center_axis',(0.392511146482166,0.,0.919747247828041));
#5495=DIRECTION('ref_axis',(0.,1.,0.));
#5496=DIRECTION('center_axis',(0.,-1.,0.));
#5497=DIRECTION('ref_axis',(0.972507099593301,0.,0.232873229978512));
#5498=DIRECTION('center_axis',(0.,1.,0.));
#5499=DIRECTION('ref_axis',(0.972507099593301,0.,0.232873229978512));
#5500=DIRECTION('center_axis',(0.,1.,0.));
#5501=DIRECTION('ref_axis',(-0.38268343236509,0.,-0.923879532511287));
#5502=DIRECTION('center_axis',(-0.372812222548024,0.,-0.927906809285718));
#5503=DIRECTION('ref_axis',(0.,1.,0.));
#5504=DIRECTION('center_axis',(0.,1.,0.));
#5505=DIRECTION('ref_axis',(-0.38268343236509,0.,-0.923879532511287));
#5506=DIRECTION('center_axis',(0.,-1.,0.));
#5507=DIRECTION('ref_axis',(-0.38268343236509,0.,-0.923879532511287));
#5508=DIRECTION('center_axis',(0.,1.,0.));
#5509=DIRECTION('ref_axis',(0.,0.,1.));
#5510=DIRECTION('center_axis',(-0.996128362168068,0.,0.087910671049441));
#5511=DIRECTION('ref_axis',(0.,1.,0.));
#5512=DIRECTION('center_axis',(0.,1.,0.));
#5513=DIRECTION('ref_axis',(-0.523000124799863,0.,0.852332604949105));
#5514=DIRECTION('center_axis',(0.,1.,0.));
#5515=DIRECTION('ref_axis',(1.22464679914735E-16,0.,-1.));
#5516=DIRECTION('center_axis',(-0.996128362168068,0.,-0.0879106710494399));
#5517=DIRECTION('ref_axis',(0.,1.,0.));
#5518=DIRECTION('center_axis',(0.,1.,0.));
#5519=DIRECTION('ref_axis',(-1.83697019872103E-16,0.,-1.));
#5520=DIRECTION('center_axis',(0.,-1.,0.));
#5521=DIRECTION('ref_axis',(-1.83697019872103E-16,0.,-1.));
#5522=DIRECTION('center_axis',(0.,1.,0.));
#5523=DIRECTION('ref_axis',(0.,0.,1.));
#5524=DIRECTION('center_axis',(-0.372812222548024,0.,0.927906809285718));
#5525=DIRECTION('ref_axis',(0.,1.,0.));
#5526=DIRECTION('center_axis',(0.,-1.,0.));
#5527=DIRECTION('ref_axis',(0.523000124799863,0.,0.852332604949105));
#5528=DIRECTION('center_axis',(0.,1.,0.));
#5529=DIRECTION('ref_axis',(0.523000124799863,0.,0.852332604949105));
#5530=DIRECTION('center_axis',(0.,1.,0.));
#5531=DIRECTION('ref_axis',(0.38268343236509,0.,-0.923879532511287));
#5532=DIRECTION('center_axis',(0.392511146482165,0.,-0.919747247828041));
#5533=DIRECTION('ref_axis',(0.,1.,0.));
#5534=DIRECTION('center_axis',(0.,1.,0.));
#5535=DIRECTION('ref_axis',(0.38268343236509,0.,-0.923879532511287));
#5536=DIRECTION('center_axis',(0.,-1.,0.));
#5537=DIRECTION('ref_axis',(0.38268343236509,0.,-0.923879532511287));
#5538=DIRECTION('center_axis',(0.,1.,0.));
#5539=DIRECTION('ref_axis',(0.,0.,1.));
#5540=DIRECTION('center_axis',(-0.766531351459009,0.,-0.642206888183571));
#5541=DIRECTION('ref_axis',(0.,1.,0.));
#5542=DIRECTION('center_axis',(0.,-1.,0.));
#5543=DIRECTION('ref_axis',(-0.972507099593301,0.,0.232873229978513));
#5544=DIRECTION('center_axis',(0.,1.,0.));
#5545=DIRECTION('ref_axis',(-0.972507099593301,0.,0.232873229978513));
#5546=DIRECTION('center_axis',(0.,1.,0.));
#5547=DIRECTION('ref_axis',(0.,0.,1.));
#5548=DIRECTION('center_axis',(-0.642206888183576,0.,-0.766531351459005));
#5549=DIRECTION('ref_axis',(0.,1.,0.));
#5550=DIRECTION('center_axis',(0.,1.,0.));
#5551=DIRECTION('ref_axis',(0.707106781186547,0.,-0.707106781186548));
#5552=DIRECTION('center_axis',(0.,-1.,0.));
#5553=DIRECTION('ref_axis',(0.707106781186547,0.,-0.707106781186548));
#5554=DIRECTION('center_axis',(0.,1.,0.));
#5555=DIRECTION('ref_axis',(0.,0.,1.));
#5556=DIRECTION('center_axis',(-0.919747247828041,0.,0.392511146482166));
#5557=DIRECTION('ref_axis',(0.,1.,0.));
#5558=DIRECTION('center_axis',(0.,-1.,0.));
#5559=DIRECTION('ref_axis',(-0.232873229978512,0.,0.972507099593301));
#5560=DIRECTION('center_axis',(0.,1.,0.));
#5561=DIRECTION('ref_axis',(-0.232873229978512,0.,0.972507099593301));
#5562=DIRECTION('center_axis',(0.,1.,0.));
#5563=DIRECTION('ref_axis',(0.923879532511287,0.,-0.38268343236509));
#5564=DIRECTION('center_axis',(0.927906809285716,0.,-0.37281222254803));
#5565=DIRECTION('ref_axis',(0.,1.,0.));
#5566=DIRECTION('center_axis',(0.,1.,0.));
#5567=DIRECTION('ref_axis',(0.923879532511287,0.,-0.382683432365089));
#5568=DIRECTION('center_axis',(0.,-1.,0.));
#5569=DIRECTION('ref_axis',(0.923879532511287,0.,-0.382683432365089));
#5570=DIRECTION('center_axis',(0.,1.,0.));
#5571=DIRECTION('ref_axis',(0.,0.,1.));
#5572=DIRECTION('center_axis',(-0.0879106710494421,0.,-0.996128362168068));
#5573=DIRECTION('ref_axis',(0.,1.,0.));
#5574=DIRECTION('center_axis',(0.,-1.,0.));
#5575=DIRECTION('ref_axis',(-0.852332604949105,0.,-0.523000124799863));
#5576=DIRECTION('center_axis',(0.,1.,0.));
#5577=DIRECTION('ref_axis',(-0.852332604949105,0.,-0.523000124799863));
#5578=DIRECTION('center_axis',(0.,1.,0.));
#5579=DIRECTION('ref_axis',(0.,0.,1.));
#5580=DIRECTION('center_axis',(0.0879106710494428,0.,-0.996128362168068));
#5581=DIRECTION('ref_axis',(0.,1.,0.));
#5582=DIRECTION('center_axis',(0.,1.,0.));
#5583=DIRECTION('ref_axis',(1.,0.,-2.44929359829471E-16));
#5584=DIRECTION('center_axis',(0.,-1.,0.));
#5585=DIRECTION('ref_axis',(1.,0.,-2.44929359829471E-16));
#5586=DIRECTION('center_axis',(0.,1.,0.));
#5587=DIRECTION('ref_axis',(0.,0.,1.));
#5588=DIRECTION('center_axis',(-0.927906809285717,0.,-0.372812222548027));
#5589=DIRECTION('ref_axis',(0.,1.,0.));
#5590=DIRECTION('center_axis',(0.,-1.,0.));
#5591=DIRECTION('ref_axis',(-0.852332604949106,0.,0.523000124799863));
#5592=DIRECTION('center_axis',(0.,1.,0.));
#5593=DIRECTION('ref_axis',(-0.852332604949106,0.,0.523000124799863));
#5594=DIRECTION('center_axis',(0.,1.,0.));
#5595=DIRECTION('ref_axis',(0.,0.,1.));
#5596=DIRECTION('center_axis',(0.919747247828042,0.,0.392511146482165));
#5597=DIRECTION('ref_axis',(0.,1.,0.));
#5598=DIRECTION('center_axis',(0.,1.,0.));
#5599=DIRECTION('ref_axis',(0.923879532511286,0.,0.382683432365091));
#5600=DIRECTION('center_axis',(0.,-1.,0.));
#5601=DIRECTION('ref_axis',(0.923879532511286,0.,0.382683432365091));
#5602=DIRECTION('center_axis',(0.,1.,0.));
#5603=DIRECTION('ref_axis',(-0.232873229978513,0.,-0.972507099593301));
#5604=DIRECTION('center_axis',(0.642206888183571,0.,-0.766531351459009));
#5605=DIRECTION('ref_axis',(0.,1.,0.));
#5606=DIRECTION('center_axis',(0.,-1.,0.));
#5607=DIRECTION('ref_axis',(-0.232873229978514,0.,-0.972507099593301));
#5608=DIRECTION('center_axis',(0.,1.,0.));
#5609=DIRECTION('ref_axis',(-0.232873229978514,0.,-0.972507099593301));
#5610=DIRECTION('center_axis',(0.,1.,0.));
#5611=DIRECTION('ref_axis',(0.,0.,1.));
#5612=DIRECTION('center_axis',(0.766531351459006,0.,-0.642206888183574));
#5613=DIRECTION('ref_axis',(0.,1.,0.));
#5614=DIRECTION('center_axis',(0.,1.,0.));
#5615=DIRECTION('ref_axis',(0.707106781186547,0.,0.707106781186547));
#5616=DIRECTION('center_axis',(0.,-1.,0.));
#5617=DIRECTION('ref_axis',(0.707106781186547,0.,0.707106781186547));
#5618=DIRECTION('center_axis',(0.,1.,0.));
#5619=DIRECTION('ref_axis',(0.,0.,1.));
#5620=DIRECTION('center_axis',(-0.392511146482166,0.,-0.919747247828041));
#5621=DIRECTION('ref_axis',(0.,1.,0.));
#5622=DIRECTION('center_axis',(0.,-1.,0.));
#5623=DIRECTION('ref_axis',(-0.972507099593301,0.,-0.232873229978513));
#5624=DIRECTION('center_axis',(0.,1.,0.));
#5625=DIRECTION('ref_axis',(-0.972507099593301,0.,-0.232873229978513));
#5626=DIRECTION('center_axis',(0.,1.,0.));
#5627=DIRECTION('ref_axis',(0.,0.,1.));
#5628=DIRECTION('center_axis',(0.37281222254803,0.,0.927906809285716));
#5629=DIRECTION('ref_axis',(0.,1.,0.));
#5630=DIRECTION('center_axis',(0.,1.,0.));
#5631=DIRECTION('ref_axis',(0.382683432365089,0.,0.923879532511287));
#5632=DIRECTION('center_axis',(0.,-1.,0.));
#5633=DIRECTION('ref_axis',(0.382683432365089,0.,0.923879532511287));
#5634=DIRECTION('center_axis',(0.,1.,0.));
#5635=DIRECTION('ref_axis',(0.523000124799863,0.,-0.852332604949105));
#5636=DIRECTION('center_axis',(0.996128362168068,0.,-0.0879106710494421));
#5637=DIRECTION('ref_axis',(0.,1.,0.));
#5638=DIRECTION('center_axis',(0.,-1.,0.));
#5639=DIRECTION('ref_axis',(0.523000124799863,0.,-0.852332604949105));
#5640=DIRECTION('center_axis',(0.,1.,0.));
#5641=DIRECTION('ref_axis',(0.523000124799863,0.,-0.852332604949105));
#5642=DIRECTION('center_axis',(0.,1.,0.));
#5643=DIRECTION('ref_axis',(0.,0.,1.));
#5644=DIRECTION('center_axis',(0.,-1.,0.));
#5645=DIRECTION('ref_axis',(6.12323399573677E-17,0.,1.));
#5646=DIRECTION('center_axis',(0.,1.,0.));
#5647=DIRECTION('ref_axis',(0.38268343236509,0.,-0.923879532511287));
#5648=DIRECTION('',(0.,1.,0.));
#5649=DIRECTION('center_axis',(0.,-1.,0.));
#5650=DIRECTION('ref_axis',(0.38268343236509,0.,-0.923879532511287));
#5651=DIRECTION('',(0.,-1.,0.));
#5652=DIRECTION('center_axis',(0.,1.,0.));
#5653=DIRECTION('ref_axis',(-0.972507099593301,0.,0.232873229978513));
#5654=DIRECTION('',(0.,-1.,0.));
#5655=DIRECTION('center_axis',(0.,1.,0.));
#5656=DIRECTION('ref_axis',(-0.972507099593301,0.,0.232873229978513));
#5657=DIRECTION('center_axis',(0.,-1.,0.));
#5658=DIRECTION('ref_axis',(1.,0.,0.));
#5659=DIRECTION('',(0.,1.,0.));
#5660=DIRECTION('center_axis',(0.,-1.,0.));
#5661=DIRECTION('ref_axis',(0.707106781186547,0.,-0.707106781186547));
#5662=DIRECTION('center_axis',(0.,-1.,0.));
#5663=DIRECTION('ref_axis',(-0.232873229978513,0.,0.972507099593301));
#5664=DIRECTION('',(0.,-1.,0.));
#5665=DIRECTION('center_axis',(0.,1.,0.));
#5666=DIRECTION('ref_axis',(-0.232873229978512,0.,0.972507099593301));
#5667=DIRECTION('center_axis',(0.,1.,0.));
#5668=DIRECTION('ref_axis',(0.923879532511287,0.,-0.382683432365089));
#5669=DIRECTION('',(0.,1.,0.));
#5670=DIRECTION('center_axis',(0.,-1.,0.));
#5671=DIRECTION('ref_axis',(0.923879532511287,0.,-0.382683432365089));
#5672=DIRECTION('center_axis',(0.,1.,0.));
#5673=DIRECTION('ref_axis',(-0.852332604949105,0.,-0.523000124799864));
#5674=DIRECTION('',(0.,-1.,0.));
#5675=DIRECTION('center_axis',(0.,1.,0.));
#5676=DIRECTION('ref_axis',(-0.852332604949105,0.,-0.523000124799863));
#5677=DIRECTION('center_axis',(0.,-1.,0.));
#5678=DIRECTION('ref_axis',(1.,0.,0.));
#5679=DIRECTION('',(0.,1.,0.));
#5680=DIRECTION('center_axis',(0.,-1.,0.));
#5681=DIRECTION('ref_axis',(1.,0.,1.17961196366423E-16));
#5682=DIRECTION('center_axis',(0.,-1.,0.));
#5683=DIRECTION('ref_axis',(-0.852332604949106,0.,0.523000124799862));
#5684=DIRECTION('',(0.,-1.,0.));
#5685=DIRECTION('center_axis',(0.,1.,0.));
#5686=DIRECTION('ref_axis',(-0.852332604949106,0.,0.523000124799863));
#5687=DIRECTION('center_axis',(0.,1.,0.));
#5688=DIRECTION('ref_axis',(0.923879532511287,0.,0.38268343236509));
#5689=DIRECTION('',(0.,1.,0.));
#5690=DIRECTION('center_axis',(0.,-1.,0.));
#5691=DIRECTION('ref_axis',(0.923879532511286,0.,0.382683432365091));
#5692=DIRECTION('center_axis',(0.,1.,0.));
#5693=DIRECTION('ref_axis',(-0.232873229978514,0.,-0.972507099593301));
#5694=DIRECTION('',(0.,-1.,0.));
#5695=DIRECTION('center_axis',(0.,1.,0.));
#5696=DIRECTION('ref_axis',(-0.232873229978514,0.,-0.972507099593301));
#5697=DIRECTION('center_axis',(0.,-1.,0.));
#5698=DIRECTION('ref_axis',(1.,0.,0.));
#5699=DIRECTION('',(0.,1.,0.));
#5700=DIRECTION('center_axis',(0.,-1.,0.));
#5701=DIRECTION('ref_axis',(0.707106781186547,0.,0.707106781186548));
#5702=DIRECTION('center_axis',(0.,-1.,0.));
#5703=DIRECTION('ref_axis',(-0.972507099593301,0.,-0.232873229978514));
#5704=DIRECTION('',(0.,-1.,0.));
#5705=DIRECTION('center_axis',(0.,1.,0.));
#5706=DIRECTION('ref_axis',(-0.972507099593301,0.,-0.232873229978513));
#5707=DIRECTION('center_axis',(0.,1.,0.));
#5708=DIRECTION('ref_axis',(0.382683432365089,0.,0.923879532511287));
#5709=DIRECTION('',(0.,1.,0.));
#5710=DIRECTION('center_axis',(0.,-1.,0.));
#5711=DIRECTION('ref_axis',(0.382683432365089,0.,0.923879532511287));
#5712=DIRECTION('center_axis',(0.,1.,0.));
#5713=DIRECTION('ref_axis',(0.523000124799864,0.,-0.852332604949105));
#5714=DIRECTION('',(0.,-1.,0.));
#5715=DIRECTION('center_axis',(0.,1.,0.));
#5716=DIRECTION('ref_axis',(0.523000124799863,0.,-0.852332604949105));
#5717=DIRECTION('center_axis',(0.,-1.,0.));
#5718=DIRECTION('ref_axis',(1.,0.,0.));
#5719=DIRECTION('center_axis',(0.,-1.,0.));
#5720=DIRECTION('ref_axis',(-1.83697019872103E-16,0.,1.));
#5721=DIRECTION('center_axis',(0.,1.,0.));
#5722=DIRECTION('ref_axis',(1.,0.,0.));
#5723=DIRECTION('center_axis',(0.,1.,0.));
#5724=DIRECTION('ref_axis',(1.,0.,0.));
#5725=DIRECTION('center_axis',(0.,-1.,0.));
#5726=DIRECTION('ref_axis',(-0.38268343236509,0.,-0.923879532511287));
#5727=DIRECTION('center_axis',(0.,-1.,0.));
#5728=DIRECTION('ref_axis',(-0.923879532511287,0.,0.38268343236509));
#5729=DIRECTION('center_axis',(0.,-1.,0.));
#5730=DIRECTION('ref_axis',(-0.923879532511287,0.,-0.38268343236509));
#5731=DIRECTION('center_axis',(0.,-1.,0.));
#5732=DIRECTION('ref_axis',(0.923879532511287,0.,-0.38268343236509));
#5733=DIRECTION('center_axis',(0.,-1.,0.));
#5734=DIRECTION('ref_axis',(0.923879532511287,0.,0.38268343236509));
#5735=DIRECTION('center_axis',(0.,-1.,0.));
#5736=DIRECTION('ref_axis',(0.38268343236509,0.,-0.923879532511287));
#5737=DIRECTION('center_axis',(0.,-1.,0.));
#5738=DIRECTION('ref_axis',(0.38268343236509,0.,0.923879532511287));
#5739=DIRECTION('center_axis',(0.,-1.,0.));
#5740=DIRECTION('ref_axis',(-0.38268343236509,0.,0.923879532511287));
#5741=DIRECTION('center_axis',(0.,-1.,0.));
#5742=DIRECTION('ref_axis',(0.,0.,-1.));
#5743=DIRECTION('center_axis',(0.766531351459009,0.,0.642206888183571));
#5744=DIRECTION('ref_axis',(-0.642206888183571,0.,0.766531351459009));
#5745=DIRECTION('center_axis',(0.,-1.,0.));
#5746=DIRECTION('ref_axis',(0.972507099593301,0.,-0.232873229978514));
#5747=DIRECTION('center_axis',(0.392511146482161,0.,-0.919747247828043));
#5748=DIRECTION('ref_axis',(0.,-1.,0.));
#5749=DIRECTION('center_axis',(0.,1.,0.));
#5750=DIRECTION('ref_axis',(0.972507099593301,0.,-0.232873229978514));
#5751=DIRECTION('center_axis',(0.,-1.,0.));
#5752=DIRECTION('ref_axis',(-0.38268343236509,0.,0.923879532511287));
#5753=DIRECTION('center_axis',(-0.372812222548022,0.,0.927906809285719));
#5754=DIRECTION('ref_axis',(0.,-1.,0.));
#5755=DIRECTION('center_axis',(0.,-1.,0.));
#5756=DIRECTION('ref_axis',(-0.382683432365091,0.,0.923879532511286));
#5757=DIRECTION('center_axis',(0.,1.,0.));
#5758=DIRECTION('ref_axis',(-0.382683432365091,0.,0.923879532511286));
#5759=DIRECTION('center_axis',(0.,-1.,0.));
#5760=DIRECTION('ref_axis',(0.,0.,-1.));
#5761=DIRECTION('center_axis',(-0.996128362168068,0.,-0.0879106710494425));
#5762=DIRECTION('ref_axis',(0.,-1.,0.));
#5763=DIRECTION('center_axis',(0.,-1.,0.));
#5764=DIRECTION('ref_axis',(-0.523000124799863,0.,-0.852332604949106));
#5765=DIRECTION('center_axis',(0.,-1.,0.));
#5766=DIRECTION('ref_axis',(1.22464679914735E-16,0.,1.));
#5767=DIRECTION('center_axis',(-0.996128362168068,0.,0.087910671049441));
#5768=DIRECTION('ref_axis',(0.,-1.,0.));
#5769=DIRECTION('center_axis',(0.,1.,0.));
#5770=DIRECTION('ref_axis',(-1.83697019872103E-16,0.,1.));
#5771=DIRECTION('center_axis',(0.,-1.,0.));
#5772=DIRECTION('ref_axis',(0.,0.,-1.));
#5773=DIRECTION('center_axis',(-0.372812222548023,0.,-0.927906809285719));
#5774=DIRECTION('ref_axis',(0.,-1.,0.));
#5775=DIRECTION('center_axis',(0.,-1.,0.));
#5776=DIRECTION('ref_axis',(0.523000124799863,0.,-0.852332604949105));
#5777=DIRECTION('center_axis',(0.,-1.,0.));
#5778=DIRECTION('ref_axis',(0.382683432365089,0.,0.923879532511287));
#5779=DIRECTION('center_axis',(0.392511146482171,0.,0.919747247828039));
#5780=DIRECTION('ref_axis',(0.,-1.,0.));
#5781=DIRECTION('center_axis',(0.,1.,0.));
#5782=DIRECTION('ref_axis',(0.382683432365089,0.,0.923879532511287));
#5783=DIRECTION('center_axis',(0.,-1.,0.));
#5784=DIRECTION('ref_axis',(0.,0.,-1.));
#5785=DIRECTION('center_axis',(-0.766531351459011,0.,0.642206888183568));
#5786=DIRECTION('ref_axis',(0.,-1.,0.));
#5787=DIRECTION('center_axis',(0.,-1.,0.));
#5788=DIRECTION('ref_axis',(-0.972507099593301,0.,-0.232873229978513));
#5789=DIRECTION('center_axis',(0.,-1.,0.));
#5790=DIRECTION('ref_axis',(0.,0.,-1.));
#5791=DIRECTION('center_axis',(-0.642206888183576,0.,0.766531351459005));
#5792=DIRECTION('ref_axis',(0.,-1.,0.));
#5793=DIRECTION('center_axis',(0.,1.,0.));
#5794=DIRECTION('ref_axis',(0.707106781186547,0.,0.707106781186548));
#5795=DIRECTION('center_axis',(0.,-1.,0.));
#5796=DIRECTION('ref_axis',(0.,0.,-1.));
#5797=DIRECTION('center_axis',(-0.919747247828043,0.,-0.392511146482161));
#5798=DIRECTION('ref_axis',(0.,-1.,0.));
#5799=DIRECTION('center_axis',(0.,-1.,0.));
#5800=DIRECTION('ref_axis',(-0.232873229978514,0.,-0.972507099593301));
#5801=DIRECTION('center_axis',(0.,-1.,0.));
#5802=DIRECTION('ref_axis',(0.923879532511287,0.,0.38268343236509));
#5803=DIRECTION('center_axis',(0.92790680928572,0.,0.372812222548021));
#5804=DIRECTION('ref_axis',(0.,-1.,0.));
#5805=DIRECTION('center_axis',(0.,1.,0.));
#5806=DIRECTION('ref_axis',(0.923879532511286,0.,0.382683432365091));
#5807=DIRECTION('center_axis',(0.,-1.,0.));
#5808=DIRECTION('ref_axis',(0.,0.,-1.));
#5809=DIRECTION('center_axis',(-0.0879106710494425,0.,0.996128362168068));
#5810=DIRECTION('ref_axis',(0.,-1.,0.));
#5811=DIRECTION('center_axis',(0.,-1.,0.));
#5812=DIRECTION('ref_axis',(-0.852332604949106,0.,0.523000124799863));
#5813=DIRECTION('center_axis',(0.,-1.,0.));
#5814=DIRECTION('ref_axis',(0.,0.,-1.));
#5815=DIRECTION('center_axis',(0.0879106710494399,0.,0.996128362168068));
#5816=DIRECTION('ref_axis',(0.,-1.,0.));
#5817=DIRECTION('center_axis',(0.,1.,0.));
#5818=DIRECTION('ref_axis',(1.,0.,1.17961196366423E-16));
#5819=DIRECTION('center_axis',(0.,-1.,0.));
#5820=DIRECTION('ref_axis',(0.,0.,-1.));
#5821=DIRECTION('center_axis',(-0.927906809285719,0.,0.372812222548023));
#5822=DIRECTION('ref_axis',(0.,-1.,0.));
#5823=DIRECTION('center_axis',(0.,-1.,0.));
#5824=DIRECTION('ref_axis',(-0.852332604949105,0.,-0.523000124799863));
#5825=DIRECTION('center_axis',(0.,-1.,0.));
#5826=DIRECTION('ref_axis',(0.,0.,-1.));
#5827=DIRECTION('center_axis',(0.919747247828038,0.,-0.392511146482172));
#5828=DIRECTION('ref_axis',(0.,-1.,0.));
#5829=DIRECTION('center_axis',(0.,1.,0.));
#5830=DIRECTION('ref_axis',(0.923879532511287,0.,-0.382683432365089));
#5831=DIRECTION('center_axis',(0.,-1.,0.));
#5832=DIRECTION('ref_axis',(-0.232873229978513,0.,0.972507099593301));
#5833=DIRECTION('center_axis',(0.642206888183571,0.,0.766531351459009));
#5834=DIRECTION('ref_axis',(0.,-1.,0.));
#5835=DIRECTION('center_axis',(0.,-1.,0.));
#5836=DIRECTION('ref_axis',(-0.232873229978512,0.,0.972507099593301));
#5837=DIRECTION('center_axis',(0.,-1.,0.));
#5838=DIRECTION('ref_axis',(0.,0.,-1.));
#5839=DIRECTION('center_axis',(0.766531351459006,0.,0.642206888183574));
#5840=DIRECTION('ref_axis',(0.,-1.,0.));
#5841=DIRECTION('center_axis',(0.,1.,0.));
#5842=DIRECTION('ref_axis',(0.707106781186547,0.,-0.707106781186547));
#5843=DIRECTION('center_axis',(0.,-1.,0.));
#5844=DIRECTION('ref_axis',(0.,0.,-1.));
#5845=DIRECTION('center_axis',(-0.392511146482168,0.,0.91974724782804));
#5846=DIRECTION('ref_axis',(0.,-1.,0.));
#5847=DIRECTION('center_axis',(0.,-1.,0.));
#5848=DIRECTION('ref_axis',(-0.972507099593301,0.,0.232873229978513));
#5849=DIRECTION('center_axis',(0.,-1.,0.));
#5850=DIRECTION('ref_axis',(0.,0.,-1.));
#5851=DIRECTION('center_axis',(0.372812222548023,0.,-0.927906809285719));
#5852=DIRECTION('ref_axis',(0.,-1.,0.));
#5853=DIRECTION('center_axis',(0.,1.,0.));
#5854=DIRECTION('ref_axis',(0.38268343236509,0.,-0.923879532511287));
#5855=DIRECTION('center_axis',(0.,-1.,0.));
#5856=DIRECTION('ref_axis',(0.523000124799863,0.,0.852332604949105));
#5857=DIRECTION('center_axis',(0.996128362168068,0.,0.087910671049441));
#5858=DIRECTION('ref_axis',(0.,-1.,0.));
#5859=DIRECTION('center_axis',(0.,1.,0.));
#5860=DIRECTION('ref_axis',(0.523000124799863,0.,0.852332604949105));
#5861=DIRECTION('center_axis',(0.,-1.,0.));
#5862=DIRECTION('ref_axis',(0.523000124799863,0.,0.852332604949105));
#5863=DIRECTION('center_axis',(0.,-1.,0.));
#5864=DIRECTION('ref_axis',(0.,0.,-1.));
#5865=DIRECTION('center_axis',(0.996128362168068,0.,-0.0879106710494399));
#5866=DIRECTION('ref_axis',(0.,-1.,0.));
#5867=DIRECTION('center_axis',(0.,1.,0.));
#5868=DIRECTION('ref_axis',(-1.60812264967664E-16,0.,-1.));
#5869=DIRECTION('center_axis',(0.,-1.,0.));
#5870=DIRECTION('ref_axis',(-0.523000124799863,0.,0.852332604949106));
#5871=DIRECTION('center_axis',(0.372812222548025,0.,0.927906809285718));
#5872=DIRECTION('ref_axis',(0.,-1.,0.));
#5873=DIRECTION('center_axis',(0.,-1.,0.));
#5874=DIRECTION('ref_axis',(-0.523000124799863,0.,0.852332604949105));
#5875=DIRECTION('center_axis',(0.,-1.,0.));
#5876=DIRECTION('ref_axis',(0.,0.,-1.));
#5877=DIRECTION('center_axis',(-0.392511146482174,0.,-0.919747247828038));
#5878=DIRECTION('ref_axis',(0.,-1.,0.));
#5879=DIRECTION('center_axis',(0.,-1.,0.));
#5880=DIRECTION('ref_axis',(-0.38268343236509,0.,-0.923879532511287));
#5881=DIRECTION('center_axis',(0.,1.,0.));
#5882=DIRECTION('ref_axis',(-0.38268343236509,0.,-0.923879532511287));
#5883=DIRECTION('center_axis',(0.,-1.,0.));
#5884=DIRECTION('ref_axis',(0.,0.,-1.));
#5885=DIRECTION('center_axis',(0.766531351459009,0.,-0.642206888183571));
#5886=DIRECTION('ref_axis',(0.,-1.,0.));
#5887=DIRECTION('center_axis',(0.,1.,0.));
#5888=DIRECTION('ref_axis',(0.972507099593301,0.,0.232873229978512));
#5889=DIRECTION('center_axis',(0.,-1.,0.));
#5890=DIRECTION('ref_axis',(0.972507099593301,0.,0.232873229978512));
#5891=DIRECTION('center_axis',(0.,-1.,0.));
#5892=DIRECTION('ref_axis',(0.,0.,-1.));
#5893=DIRECTION('center_axis',(0.642206888183569,0.,-0.76653135145901));
#5894=DIRECTION('ref_axis',(0.,-1.,0.));
#5895=DIRECTION('center_axis',(0.,-1.,0.));
#5896=DIRECTION('ref_axis',(-0.707106781186547,0.,-0.707106781186548));
#5897=DIRECTION('center_axis',(0.,1.,0.));
#5898=DIRECTION('ref_axis',(-0.707106781186547,0.,-0.707106781186548));
#5899=DIRECTION('center_axis',(0.,-1.,0.));
#5900=DIRECTION('ref_axis',(0.232873229978514,0.,0.972507099593301));
#5901=DIRECTION('center_axis',(0.919747247828041,0.,0.392511146482166));
#5902=DIRECTION('ref_axis',(0.,-1.,0.));
#5903=DIRECTION('center_axis',(0.,1.,0.));
#5904=DIRECTION('ref_axis',(0.232873229978512,0.,0.972507099593301));
#5905=DIRECTION('center_axis',(0.,-1.,0.));
#5906=DIRECTION('ref_axis',(0.232873229978512,0.,0.972507099593301));
#5907=DIRECTION('center_axis',(0.,-1.,0.));
#5908=DIRECTION('ref_axis',(0.,0.,-1.));
#5909=DIRECTION('center_axis',(-0.927906809285719,0.,-0.372812222548023));
#5910=DIRECTION('ref_axis',(0.,-1.,0.));
#5911=DIRECTION('center_axis',(0.,-1.,0.));
#5912=DIRECTION('ref_axis',(-0.923879532511287,0.,-0.38268343236509));
#5913=DIRECTION('center_axis',(0.,1.,0.));
#5914=DIRECTION('ref_axis',(-0.923879532511287,0.,-0.38268343236509));
#5915=DIRECTION('center_axis',(0.,-1.,0.));
#5916=DIRECTION('ref_axis',(0.,0.,-1.));
#5917=DIRECTION('center_axis',(0.0879106710494421,0.,-0.996128362168068));
#5918=DIRECTION('ref_axis',(0.,-1.,0.));
#5919=DIRECTION('center_axis',(0.,1.,0.));
#5920=DIRECTION('ref_axis',(0.852332604949105,0.,-0.523000124799863));
#5921=DIRECTION('center_axis',(0.,-1.,0.));
#5922=DIRECTION('ref_axis',(0.852332604949105,0.,-0.523000124799863));
#5923=DIRECTION('center_axis',(0.,-1.,0.));
#5924=DIRECTION('ref_axis',(0.,0.,-1.));
#5925=DIRECTION('center_axis',(-0.0879106710494421,0.,-0.996128362168068));
#5926=DIRECTION('ref_axis',(0.,-1.,0.));
#5927=DIRECTION('center_axis',(0.,-1.,0.));
#5928=DIRECTION('ref_axis',(-1.,0.,-1.22464679914735E-16));
#5929=DIRECTION('center_axis',(0.,1.,0.));
#5930=DIRECTION('ref_axis',(-1.,0.,-1.22464679914735E-16));
#5931=DIRECTION('center_axis',(0.,-1.,0.));
#5932=DIRECTION('ref_axis',(0.,0.,-1.));
#5933=DIRECTION('center_axis',(0.927906809285717,0.,-0.372812222548027));
#5934=DIRECTION('ref_axis',(0.,-1.,0.));
#5935=DIRECTION('center_axis',(0.,1.,0.));
#5936=DIRECTION('ref_axis',(0.852332604949105,0.,0.523000124799863));
#5937=DIRECTION('center_axis',(0.,-1.,0.));
#5938=DIRECTION('ref_axis',(0.852332604949105,0.,0.523000124799863));
#5939=DIRECTION('center_axis',(0.,-1.,0.));
#5940=DIRECTION('ref_axis',(-0.923879532511287,0.,0.382683432365089));
#5941=DIRECTION('center_axis',(-0.919747247828039,0.,0.392511146482171));
#5942=DIRECTION('ref_axis',(0.,-1.,0.));
#5943=DIRECTION('center_axis',(0.,-1.,0.));
#5944=DIRECTION('ref_axis',(-0.923879532511287,0.,0.382683432365089));
#5945=DIRECTION('center_axis',(0.,1.,0.));
#5946=DIRECTION('ref_axis',(-0.923879532511287,0.,0.382683432365089));
#5947=DIRECTION('center_axis',(0.,-1.,0.));
#5948=DIRECTION('ref_axis',(0.,0.,-1.));
#5949=DIRECTION('center_axis',(-0.642206888183565,0.,-0.766531351459014));
#5950=DIRECTION('ref_axis',(0.,-1.,0.));
#5951=DIRECTION('center_axis',(0.,1.,0.));
#5952=DIRECTION('ref_axis',(0.232873229978513,0.,-0.972507099593301));
#5953=DIRECTION('center_axis',(0.,-1.,0.));
#5954=DIRECTION('ref_axis',(0.232873229978513,0.,-0.972507099593301));
#5955=DIRECTION('center_axis',(0.,-1.,0.));
#5956=DIRECTION('ref_axis',(0.,0.,-1.));
#5957=DIRECTION('center_axis',(0.,1.,0.));
#5958=DIRECTION('ref_axis',(-0.707106781186548,0.,0.707106781186547));
#5959=DIRECTION('center_axis',(0.,-1.,0.));
#5960=DIRECTION('ref_axis',(-0.707106781186548,0.,0.707106781186547));
#5961=DIRECTION('center_axis',(0.,-1.,0.));
#5962=DIRECTION('ref_axis',(0.523000124799864,0.,0.852332604949105));
#5963=DIRECTION('',(0.,1.,0.));
#5964=DIRECTION('center_axis',(0.,-1.,0.));
#5965=DIRECTION('ref_axis',(1.,0.,0.));
#5966=DIRECTION('center_axis',(0.,1.,0.));
#5967=DIRECTION('ref_axis',(-0.38268343236509,0.,-0.923879532511287));
#5968=DIRECTION('',(0.,-1.,0.));
#5969=DIRECTION('center_axis',(0.,-1.,0.));
#5970=DIRECTION('ref_axis',(0.972507099593301,0.,0.232873229978513));
#5971=DIRECTION('',(0.,1.,0.));
#5972=DIRECTION('center_axis',(0.,-1.,0.));
#5973=DIRECTION('ref_axis',(1.,0.,0.));
#5974=DIRECTION('',(0.,-1.,0.));
#5975=DIRECTION('center_axis',(0.,1.,0.));
#5976=DIRECTION('ref_axis',(0.232873229978513,0.,0.972507099593301));
#5977=DIRECTION('',(0.,1.,0.));
#5978=DIRECTION('center_axis',(0.,1.,0.));
#5979=DIRECTION('ref_axis',(-0.923879532511287,0.,-0.38268343236509));
#5980=DIRECTION('',(0.,-1.,0.));
#5981=DIRECTION('center_axis',(0.,-1.,0.));
#5982=DIRECTION('ref_axis',(0.852332604949105,0.,-0.523000124799864));
#5983=DIRECTION('',(0.,1.,0.));
#5984=DIRECTION('center_axis',(0.,-1.,0.));
#5985=DIRECTION('ref_axis',(-1.,0.,1.22464679914735E-16));
#5986=DIRECTION('',(0.,-1.,0.));
#5987=DIRECTION('center_axis',(0.,1.,0.));
#5988=DIRECTION('ref_axis',(0.852332604949106,0.,0.523000124799863));
#5989=DIRECTION('',(0.,1.,0.));
#5990=DIRECTION('center_axis',(0.,1.,0.));
#5991=DIRECTION('ref_axis',(-0.923879532511287,0.,0.38268343236509));
#5992=DIRECTION('',(0.,-1.,0.));
#5993=DIRECTION('center_axis',(0.,-1.,0.));
#5994=DIRECTION('ref_axis',(0.232873229978513,0.,-0.972507099593301));
#5995=DIRECTION('',(0.,1.,0.));
#5996=DIRECTION('center_axis',(0.,-1.,0.));
#5997=DIRECTION('ref_axis',(1.,0.,0.));
#5998=DIRECTION('',(0.,-1.,0.));
#5999=DIRECTION('center_axis',(0.,1.,0.));
#6000=DIRECTION('ref_axis',(0.972507099593301,0.,-0.232873229978514));
#6001=DIRECTION('',(0.,1.,0.));
#6002=DIRECTION('center_axis',(0.,1.,0.));
#6003=DIRECTION('ref_axis',(1.,0.,0.));
#6004=DIRECTION('center_axis',(0.,-1.,0.));
#6005=DIRECTION('ref_axis',(1.,0.,0.));
#6006=DIRECTION('center_axis',(0.,1.,0.));
#6007=DIRECTION('ref_axis',(-0.38268343236509,0.,-0.923879532511287));
#6008=DIRECTION('center_axis',(0.,1.,0.));
#6009=DIRECTION('ref_axis',(0.923879532511287,0.,0.38268343236509));
#6010=DIRECTION('center_axis',(0.,1.,0.));
#6011=DIRECTION('ref_axis',(0.923879532511287,0.,-0.38268343236509));
#6012=DIRECTION('center_axis',(0.,1.,0.));
#6013=DIRECTION('ref_axis',(0.38268343236509,0.,-0.923879532511287));
#6014=DIRECTION('center_axis',(0.,1.,0.));
#6015=DIRECTION('ref_axis',(-0.923879532511287,0.,-0.38268343236509));
#6016=DIRECTION('center_axis',(0.,1.,0.));
#6017=DIRECTION('ref_axis',(0.38268343236509,0.,0.923879532511287));
#6018=DIRECTION('center_axis',(0.,1.,0.));
#6019=DIRECTION('ref_axis',(-0.923879532511287,0.,0.38268343236509));
#6020=DIRECTION('center_axis',(0.,1.,0.));
#6021=DIRECTION('ref_axis',(-0.38268343236509,0.,0.923879532511287));
#6022=DIRECTION('center_axis',(0.,-1.,0.));
#6023=DIRECTION('ref_axis',(0.,0.,-1.));
#6024=DIRECTION('center_axis',(-1.,0.,-1.22464679914735E-16));
#6025=DIRECTION('ref_axis',(-1.22464679914735E-16,0.,1.));
#6026=DIRECTION('center_axis',(0.,-1.,0.));
#6027=DIRECTION('ref_axis',(1.,0.,0.));
#6028=DIRECTION('center_axis',(0.,-1.,0.));
#6029=DIRECTION('ref_axis',(1.,0.,0.));
#6030=DIRECTION('center_axis',(0.,-1.,0.));
#6031=DIRECTION('ref_axis',(1.,0.,0.));
#6032=DIRECTION('',(0.,-1.,0.));
#6033=DIRECTION('center_axis',(0.,1.,0.));
#6034=DIRECTION('ref_axis',(1.,0.,0.));
#6035=DIRECTION('center_axis',(0.,1.,0.));
#6036=DIRECTION('ref_axis',(1.,0.,0.));
#6037=DIRECTION('center_axis',(0.,1.,0.));
#6038=DIRECTION('ref_axis',(0.,0.,1.));
#6039=DIRECTION('center_axis',(-1.,0.,1.22464679914735E-16));
#6040=DIRECTION('ref_axis',(-1.22464679914735E-16,0.,-1.));
#6041=DIRECTION('center_axis',(0.,1.,0.));
#6042=DIRECTION('ref_axis',(-0.38268343236509,0.,0.923879532511287));
#6043=DIRECTION('center_axis',(0.,1.,0.));
#6044=DIRECTION('ref_axis',(-0.38268343236509,0.,-0.923879532511287));
#6045=DIRECTION('',(0.,1.,0.));
#6046=DIRECTION('center_axis',(0.,1.,0.));
#6047=DIRECTION('ref_axis',(-0.38268343236509,0.,0.923879532511287));
#6048=DIRECTION('',(0.,1.,0.));
#6049=DIRECTION('center_axis',(0.,1.,0.));
#6050=DIRECTION('ref_axis',(-0.923879532511287,0.,0.38268343236509));
#6051=DIRECTION('',(0.,1.,0.));
#6052=DIRECTION('center_axis',(0.,1.,0.));
#6053=DIRECTION('ref_axis',(0.38268343236509,0.,0.923879532511287));
#6054=DIRECTION('',(0.,1.,0.));
#6055=DIRECTION('center_axis',(0.,1.,0.));
#6056=DIRECTION('ref_axis',(-0.923879532511287,0.,-0.38268343236509));
#6057=DIRECTION('',(0.,1.,0.));
#6058=DIRECTION('center_axis',(0.,1.,0.));
#6059=DIRECTION('ref_axis',(0.38268343236509,0.,-0.923879532511287));
#6060=DIRECTION('',(0.,1.,0.));
#6061=DIRECTION('center_axis',(0.,1.,0.));
#6062=DIRECTION('ref_axis',(0.923879532511287,0.,-0.38268343236509));
#6063=DIRECTION('',(0.,1.,0.));
#6064=DIRECTION('center_axis',(0.,1.,0.));
#6065=DIRECTION('ref_axis',(0.923879532511287,0.,0.38268343236509));
#6066=DIRECTION('',(0.,1.,0.));
#26042=CARTESIAN_POINT('',(0.,0.,0.));
#26043=CARTESIAN_POINT('Origin',(0.,0.,-25.2396150285955));
#26044=CARTESIAN_POINT('',(2.48705727606859,3.24064362520075,-38.7031482120265));
#26045=CARTESIAN_POINT('',(2.49067940755002,3.24534996886546,-38.8073295092502));
#26046=CARTESIAN_POINT('',(2.4870572760686,3.24064362520075,-25.2396150285955));
#26047=CARTESIAN_POINT('',(4.07943565862452,-0.213142457391218,-39.));
#26048=CARTESIAN_POINT('Ctrl Pts',(2.49067940755052,3.24534996886507,-38.8073295092502));
#26049=CARTESIAN_POINT('Ctrl Pts',(3.52935397857082,2.44593384313725,-38.8715530061668));
#26050=CARTESIAN_POINT('Ctrl Pts',(4.14824284080374,1.10379118401926,-38.9357765030834));
#26051=CARTESIAN_POINT('Ctrl Pts',(4.07943565862452,-0.213142457391218,
-39.));
#26052=CARTESIAN_POINT('',(3.42517145598067,-2.22607850201542,-38.9999998622677));
#26053=CARTESIAN_POINT('Origin',(0.,0.,-39.));
#26054=CARTESIAN_POINT('Ctrl Pts',(2.48705727606859,3.24064362520075,-38.7031482120265));
#26055=CARTESIAN_POINT('Ctrl Pts',(2.58203140296112,3.16775498928613,-38.7089631647656));
#26056=CARTESIAN_POINT('Ctrl Pts',(2.67381530421241,3.09067498482409,-38.7147781175047));
#26057=CARTESIAN_POINT('Ctrl Pts',(2.76202883781055,3.00972119956366,-38.7205930702438));
#26058=CARTESIAN_POINT('Ctrl Pts',(2.85024920780721,2.92876114052283,-38.7264084736318));
#26059=CARTESIAN_POINT('Ctrl Pts',(2.93489836057956,2.84392697867096,-38.7322238770199));
#26060=CARTESIAN_POINT('Ctrl Pts',(3.0156317065863,2.75557442473097,-38.7380392804079));
#26061=CARTESIAN_POINT('Ctrl Pts',(3.096390141849,2.66719441373697,-38.7438564910311));
#26062=CARTESIAN_POINT('Ctrl Pts',(3.17323007601772,2.57529413591597,-38.7496737016544));
#26063=CARTESIAN_POINT('Ctrl Pts',(3.24584644002518,2.48026326985179,-38.7554909122776));
#26064=CARTESIAN_POINT('Ctrl Pts',(3.31854039094952,2.3851308681075,-38.7613143382965));
#26065=CARTESIAN_POINT('Ctrl Pts',(3.38700151711333,2.286861524617,-38.7671377643155));
#26066=CARTESIAN_POINT('Ctrl Pts',(3.45096734123387,2.18587497577908,-38.7729611903344));
#26067=CARTESIAN_POINT('Ctrl Pts',(3.51497417259674,2.08482368643423,-38.7787883496382));
#26068=CARTESIAN_POINT('Ctrl Pts',(3.5744797600348,1.98105207395486,-38.784615508942));
#26069=CARTESIAN_POINT('Ctrl Pts',(3.62926773202761,1.87500419446549,-38.7904426682458));
#26070=CARTESIAN_POINT('Ctrl Pts',(3.68413107705314,1.76881042254755,-38.7962778441023));
#26071=CARTESIAN_POINT('Ctrl Pts',(3.73426368290503,1.66033450106111,-38.8021130199589));
#26072=CARTESIAN_POINT('Ctrl Pts',(3.77949735438832,1.55004024082334,-38.8079481958155));
#26073=CARTESIAN_POINT('Ctrl Pts',(3.7891274022615,1.52655908239872,-38.8091904788538));
#26074=CARTESIAN_POINT('Ctrl Pts',(3.79853558888994,1.5029955610706,-38.8104327618922));
#26075=CARTESIAN_POINT('Ctrl Pts',(3.80772058580551,1.4793542308835,-38.8116750449306));
#26076=CARTESIAN_POINT('Ctrl Pts',(3.85054135128359,1.36913755200637,-38.8174666103641));
#26077=CARTESIAN_POINT('Ctrl Pts',(3.88864421705721,1.25687596525225,-38.8232581757977));
#26078=CARTESIAN_POINT('Ctrl Pts',(3.92182946063559,1.14301298404293,-38.8290497412312));
#26079=CARTESIAN_POINT('Ctrl Pts',(3.95497352447858,1.02929129597876,-38.8348341198822));
#26080=CARTESIAN_POINT('Ctrl Pts',(3.98321198630328,0.913972558369433,-38.8406184985331));
#26081=CARTESIAN_POINT('Ctrl Pts',(4.00639324377989,0.797520016171896,-38.846402877184));
#26082=CARTESIAN_POINT('Ctrl Pts',(4.02955195414875,0.681180740824569,-38.8521816296946));
#26083=CARTESIAN_POINT('Ctrl Pts',(4.04766316351743,0.563710257410262,-38.8579603822051));
#26084=CARTESIAN_POINT('Ctrl Pts',(4.06062532717396,0.445586077333446,-38.8637391347157));
#26085=CARTESIAN_POINT('Ctrl Pts',(4.0735787196456,0.327541829052746,-38.8695139768832));
#26086=CARTESIAN_POINT('Ctrl Pts',(4.08138995193574,0.208845173517891,-38.8752888190507));
#26087=CARTESIAN_POINT('Ctrl Pts',(4.08400883807448,0.0899822789749685,
-38.8810636612182));
#26088=CARTESIAN_POINT('Ctrl Pts',(4.08662679830471,-0.0288385915317061,
-38.8868364616873));
#26089=CARTESIAN_POINT('Ctrl Pts',(4.08405605265242,-0.147825171524291,
-38.8926092621564));
#26090=CARTESIAN_POINT('Ctrl Pts',(4.07629844063419,-0.266488316598069,
-38.8983820626256));
#26091=CARTESIAN_POINT('Ctrl Pts',(4.06854168767119,-0.385138321262834,
-38.9041542238317));
#26092=CARTESIAN_POINT('Ctrl Pts',(4.0555992376166,-0.503464549876765,-38.9099263850378));
#26093=CARTESIAN_POINT('Ctrl Pts',(4.03752497766301,-0.620980720109175,
-38.9156985462439));
#26094=CARTESIAN_POINT('Ctrl Pts',(4.01944833046838,-0.738512411830461,
-38.9214714698348));
#26095=CARTESIAN_POINT('Ctrl Pts',(3.99623858913628,-0.855233424042061,
-38.9272443934257));
#26096=CARTESIAN_POINT('Ctrl Pts',(3.96800103914963,-0.970666138951715,
-38.9330173170165));
#26097=CARTESIAN_POINT('Ctrl Pts',(3.93973585225294,-1.08621183121103,-38.9387958907353));
#26098=CARTESIAN_POINT('Ctrl Pts',(3.90643312665145,-1.20046630562591,-38.9445744644541));
#26099=CARTESIAN_POINT('Ctrl Pts',(3.86824853021083,-1.31296546356776,-38.9503530381729));
#26100=CARTESIAN_POINT('Ctrl Pts',(3.83004492559059,-1.42552062325906,-38.9561344884487));
#26101=CARTESIAN_POINT('Ctrl Pts',(3.78695475915395,-1.53631834078466,-38.9619159387245));
#26102=CARTESIAN_POINT('Ctrl Pts',(3.73918186636588,-1.64491457840235,-38.9676973890003));
#26103=CARTESIAN_POINT('Ctrl Pts',(3.69133422795344,-1.75368072604874,-38.9734878849521));
#26104=CARTESIAN_POINT('Ctrl Pts',(3.63878940876722,-1.86023814152513,-38.9792783809039));
#26105=CARTESIAN_POINT('Ctrl Pts',(3.5817974250089,-1.96416705150035,-38.9850688768557));
#26106=CARTESIAN_POINT('Ctrl Pts',(3.53281218637065,-2.0534950959169,-38.990045871993));
#26107=CARTESIAN_POINT('Ctrl Pts',(3.48054239181174,-2.14088161936829,-38.9950228671304));
#26108=CARTESIAN_POINT('Ctrl Pts',(3.42517145598068,-2.22607850201542,-38.9999998622677));
#26109=CARTESIAN_POINT('Origin',(0.,0.,-25.2396150285955));
#26110=CARTESIAN_POINT('',(2.48705727606859,3.24064362520075,-37.4531876190354));
#26111=CARTESIAN_POINT('',(2.4870572760686,3.24064362520074,-37.5572541797712));
#26112=CARTESIAN_POINT('',(2.4870572760686,3.24064362520075,-25.2396150285955));
#26113=CARTESIAN_POINT('',(-4.08499877004747,0.0031699701342642,-38.3646150285955));
#26114=CARTESIAN_POINT('Ctrl Pts',(2.4870572760686,3.24064362520074,-37.5572541797712));
#26115=CARTESIAN_POINT('Ctrl Pts',(2.58191367553083,3.16784534012255,-37.5630654428848));
#26116=CARTESIAN_POINT('Ctrl Pts',(2.67352246407981,3.09091617849925,-37.5688767059985));
#26117=CARTESIAN_POINT('Ctrl Pts',(2.76151875527619,3.01018922399537,-37.5746879691121));
#26118=CARTESIAN_POINT('Ctrl Pts',(2.84956217068161,2.92941903819358,-37.5805023443021));
#26119=CARTESIAN_POINT('Ctrl Pts',(2.9339889461399,2.84484729630921,-37.5863167194922));
#26120=CARTESIAN_POINT('Ctrl Pts',(3.01447201343793,2.75684302784897,-37.5921310946822));
#26121=CARTESIAN_POINT('Ctrl Pts',(3.09508237545809,2.66869956888225,-37.5979546660833));
#26122=CARTESIAN_POINT('Ctrl Pts',(3.171736305253,2.57711304979982,-37.6037782374843));
#26123=CARTESIAN_POINT('Ctrl Pts',(3.24414755374533,2.48248497468327,-37.6096018088854));
#26124=CARTESIAN_POINT('Ctrl Pts',(3.30369403183372,2.40466876906888,-37.614390749472));
#26125=CARTESIAN_POINT('Ctrl Pts',(3.36037217691526,2.32479640134805,-37.6191796900586));
#26126=CARTESIAN_POINT('Ctrl Pts',(3.41404578623918,2.2431041815891,-37.6239686306452));
#26127=CARTESIAN_POINT('Ctrl Pts',(3.47934871858892,2.14371191847105,-37.6297951786842));
#26128=CARTESIAN_POINT('Ctrl Pts',(3.54041199454479,2.04130679768247,-37.6356217267232));
#26129=CARTESIAN_POINT('Ctrl Pts',(3.59694625009755,1.93628579344816,-37.6414482747623));
#26130=CARTESIAN_POINT('Ctrl Pts',(3.65340951727827,1.8313966609445,-37.6472675065793));
#26131=CARTESIAN_POINT('Ctrl Pts',(3.70535488395295,1.7238985343542,-37.6530867383964));
#26132=CARTESIAN_POINT('Ctrl Pts',(3.75253602496439,1.61421757559025,-37.6589059702135));
#26133=CARTESIAN_POINT('Ctrl Pts',(3.79967018289017,1.50464583737016,-37.6647194072266));
#26134=CARTESIAN_POINT('Ctrl Pts',(3.84204939321694,1.39289596388548,-37.6705328442396));
#26135=CARTESIAN_POINT('Ctrl Pts',(3.87947335467167,1.27941841881089,-37.6763462812527));
#26136=CARTESIAN_POINT('Ctrl Pts',(3.91815149296423,1.16213793831432,-37.6823545420568));
#26137=CARTESIAN_POINT('Ctrl Pts',(3.95153621012533,1.04301234482587,-37.688362802861));
#26138=CARTESIAN_POINT('Ctrl Pts',(3.97946042882905,0.922561485963775,-37.6943710636652));
#26139=CARTESIAN_POINT('Ctrl Pts',(4.00644899369114,0.806146561285478,-37.7001780063103));
#26140=CARTESIAN_POINT('Ctrl Pts',(4.02833702888313,0.688494188699189,-37.7059849489554));
#26141=CARTESIAN_POINT('Ctrl Pts',(4.04502465962916,0.570088153702579,-37.7117918916005));
#26142=CARTESIAN_POINT('Ctrl Pts',(4.06170984580576,0.45169946399464,-37.7175979835872));
#26143=CARTESIAN_POINT('Ctrl Pts',(4.0731960857049,0.332557735198908,-37.7234040755738));
#26144=CARTESIAN_POINT('Ctrl Pts',(4.07943501693327,0.213154738672663,-37.7292101675604));
#26145=CARTESIAN_POINT('Ctrl Pts',(4.08567450227854,0.0937411372504796,
-37.7350167752209));
#26146=CARTESIAN_POINT('Ctrl Pts',(4.08666573107,-0.0259333707249715,-37.7408233828814));
#26147=CARTESIAN_POINT('Ctrl Pts',(4.08241242132786,-0.145374764618867,
-37.7466299905419));
#26148=CARTESIAN_POINT('Ctrl Pts',(4.07815773300344,-0.264854871844148,
-37.7524384802394));
#26149=CARTESIAN_POINT('Ctrl Pts',(4.06865513996115,-0.384101307339019,
-37.7582469699369));
#26150=CARTESIAN_POINT('Ctrl Pts',(4.05396035404529,-0.502623564737019,
-37.7640554596344));
#26151=CARTESIAN_POINT('Ctrl Pts',(4.03924943015729,-0.621275984554532,
-37.7698703282779));
#26152=CARTESIAN_POINT('Ctrl Pts',(4.01933498187758,-0.739202233838021,
-37.7756851969213));
#26153=CARTESIAN_POINT('Ctrl Pts',(3.9943241614115,-0.855920261218504,-37.7815000655648));
#26154=CARTESIAN_POINT('Ctrl Pts',(3.96929693958899,-0.972714828829665,
-37.7873187474271));
#26155=CARTESIAN_POINT('Ctrl Pts',(3.93916679224495,-1.08829920282149,-37.7931374292895));
#26156=CARTESIAN_POINT('Ctrl Pts',(3.90409077974541,-1.20220638141163,-37.7989561111518));
#26157=CARTESIAN_POINT('Ctrl Pts',(3.86896522204763,-1.31627445496511,-37.8047830119571));
#26158=CARTESIAN_POINT('Ctrl Pts',(3.82887999235549,-1.42866022202432,-37.8106099127624));
#26159=CARTESIAN_POINT('Ctrl Pts',(3.78404033163829,-1.53891642675447,-37.8164368135677));
#26160=CARTESIAN_POINT('Ctrl Pts',(3.77350362207393,-1.56482513320607,-37.8178060558962));
#26161=CARTESIAN_POINT('Ctrl Pts',(3.76270457892702,-1.59061635614294,-37.8191752982246));
#26162=CARTESIAN_POINT('Ctrl Pts',(3.75164622762479,-1.61628449932204,-37.820544540553));
#26163=CARTESIAN_POINT('Ctrl Pts',(3.70458780895145,-1.72551436508384,-37.8263713023365));
#26164=CARTESIAN_POINT('Ctrl Pts',(3.65268010714795,-1.83286134077567,-37.83219806412));
#26165=CARTESIAN_POINT('Ctrl Pts',(3.59609550443534,-1.93786535212846,-37.8380248259034));
#26166=CARTESIAN_POINT('Ctrl Pts',(3.53958176345365,-2.04273786541213,-37.8438442907474));
#26167=CARTESIAN_POINT('Ctrl Pts',(3.47840296306761,-2.14527289457213,-37.8496637555913));
#26168=CARTESIAN_POINT('Ctrl Pts',(3.41277953405773,-2.24503025634772,-37.8554832204352));
#26169=CARTESIAN_POINT('Ctrl Pts',(3.34722123913477,-2.3446886046342,-37.861296909209));
#26170=CARTESIAN_POINT('Ctrl Pts',(3.27722731483667,-2.44157443156378,-37.8671105979828));
#26171=CARTESIAN_POINT('Ctrl Pts',(3.20306380202618,-2.53527262442318,-37.8729242867566));
#26172=CARTESIAN_POINT('Ctrl Pts',(3.12641930508808,-2.63210529298986,-37.8789324602442));
#26173=CARTESIAN_POINT('Ctrl Pts',(3.04532156827027,-2.72553292565708,-37.8849406337319));
#26174=CARTESIAN_POINT('Ctrl Pts',(2.96011278962525,-2.81513006319371,-37.8909488072196));
#26175=CARTESIAN_POINT('Ctrl Pts',(2.87775369479293,-2.9017307546298,-37.8967560460735));
#26176=CARTESIAN_POINT('Ctrl Pts',(2.79155444190347,-2.98475274771809,-37.9025632849274));
#26177=CARTESIAN_POINT('Ctrl Pts',(2.7018641382783,-3.06384646780573,-37.9083705237813));
#26178=CARTESIAN_POINT('Ctrl Pts',(2.61218672843152,-3.14292881746806,-37.914176927793));
#26179=CARTESIAN_POINT('Ctrl Pts',(2.51901957173523,-3.21808374759441,-37.9199833318047));
#26180=CARTESIAN_POINT('Ctrl Pts',(2.42274677984221,-3.28900031024082,-37.9257897358164));
#26181=CARTESIAN_POINT('Ctrl Pts',(2.32646518265715,-3.35992335905047,-37.9315966708928));
#26182=CARTESIAN_POINT('Ctrl Pts',(2.22707771385739,-3.42660702776142,-37.9374036059692));
#26183=CARTESIAN_POINT('Ctrl Pts',(2.12499901165192,-3.48878262442336,-37.9432105410456));
#26184=CARTESIAN_POINT('Ctrl Pts',(2.0228869623055,-3.55097853265217,-37.9490193731356));
#26185=CARTESIAN_POINT('Ctrl Pts',(1.9180822791219,-3.60866322786948,-37.9548282052256));
#26186=CARTESIAN_POINT('Ctrl Pts',(1.81102526660694,-3.66161337168621,-37.9606370373156));
#26187=CARTESIAN_POINT('Ctrl Pts',(1.70385031760053,-3.71462184661117,-37.9664522685499));
#26188=CARTESIAN_POINT('Ctrl Pts',(1.59441845235195,-3.7628851784569,-37.9722674997842));
#26189=CARTESIAN_POINT('Ctrl Pts',(1.4831912131835,-3.80622763706209,-37.9780827310185));
#26190=CARTESIAN_POINT('Ctrl Pts',(1.37189080576485,-3.84959860749477,-37.9839017876674));
#26191=CARTESIAN_POINT('Ctrl Pts',(1.25879305747633,-3.88804212683319,-37.9897208443162));
#26192=CARTESIAN_POINT('Ctrl Pts',(1.14437439735977,-3.92143242179021,-37.995539900965));
#26193=CARTESIAN_POINT('Ctrl Pts',(1.02979383999381,-3.95486996251034,-38.0013671913168));
#26194=CARTESIAN_POINT('Ctrl Pts',(0.9138890351005,-3.98323991156655,-38.0071944816687));
#26195=CARTESIAN_POINT('Ctrl Pts',(0.797146427651654,-4.00646759289055,
-38.0130217720205));
#26196=CARTESIAN_POINT('Ctrl Pts',(0.769775764253665,-4.0119133942216,-38.0143879981673));
#26197=CARTESIAN_POINT('Ctrl Pts',(0.742359067800449,-4.01707675908078,
-38.0157542243141));
#26198=CARTESIAN_POINT('Ctrl Pts',(0.714902633431441,-4.02195713859718,
-38.0171204504609));
#26199=CARTESIAN_POINT('Ctrl Pts',(0.597972576197206,-4.04274144906181,
-38.0229388644397));
#26200=CARTESIAN_POINT('Ctrl Pts',(0.479945563511625,-4.0584560111944,-38.0287572784184));
#26201=CARTESIAN_POINT('Ctrl Pts',(0.361299229961964,-4.06899101331385,
-38.0345756923972));
#26202=CARTESIAN_POINT('Ctrl Pts',(0.242802307684981,-4.07951274871004,
-38.04038677925));
#26203=CARTESIAN_POINT('Ctrl Pts',(0.123688019616775,-4.08486786109853,
-38.0461978661028));
#26204=CARTESIAN_POINT('Ctrl Pts',(0.00444393378988152,-4.0849975827964,
-38.0520089529555));
#26205=CARTESIAN_POINT('Ctrl Pts',(-0.11468121592749,-4.08512717510762,
-38.05781424373));
#26206=CARTESIAN_POINT('Ctrl Pts',(-0.233935499099669,-4.08004174435223,
-38.0636195345044));
#26207=CARTESIAN_POINT('Ctrl Pts',(-0.352827096490942,-4.06973439427953,
-38.0694248252788));
#26208=CARTESIAN_POINT('Ctrl Pts',(-0.475938021876412,-4.05906124803905,
-38.0754361392409));
#26209=CARTESIAN_POINT('Ctrl Pts',(-0.59865959577594,-4.0427886210935,-38.081447453203));
#26210=CARTESIAN_POINT('Ctrl Pts',(-0.720446289394505,-4.02096781187038,
-38.087458767165));
#26211=CARTESIAN_POINT('Ctrl Pts',(-0.837928434466314,-3.99991825876597,
-38.0932576113407));
#26212=CARTESIAN_POINT('Ctrl Pts',(-0.954540230615088,-3.973706162567,-38.0990564555164));
#26213=CARTESIAN_POINT('Ctrl Pts',(-1.06979876696172,-3.94243016402411,
-38.1048552996921));
#26214=CARTESIAN_POINT('Ctrl Pts',(-1.18504102029999,-3.91115858395956,
-38.1106533246432));
#26215=CARTESIAN_POINT('Ctrl Pts',(-1.2989299992701,-3.87482463129699,-38.1164513495942));
#26216=CARTESIAN_POINT('Ctrl Pts',(-1.41099576212991,-3.83357743618822,
-38.1222493745453));
#26217=CARTESIAN_POINT('Ctrl Pts',(-1.5230722653205,-3.79232628796738,-38.1280479551764));
#26218=CARTESIAN_POINT('Ctrl Pts',(-1.63332482102462,-3.74616110239697,
-38.1338465358075));
#26219=CARTESIAN_POINT('Ctrl Pts',(-1.74130196855822,-3.6952797531845,-38.1396451164386));
#26220=CARTESIAN_POINT('Ctrl Pts',(-1.84931506733781,-3.64438146290678,
-38.1454456277208));
#26221=CARTESIAN_POINT('Ctrl Pts',(-1.95505088140968,-3.58876406050027,
-38.151246139003));
#26222=CARTESIAN_POINT('Ctrl Pts',(-2.05808170810105,-3.52867180151114,
-38.1570466502852));
#26223=CARTESIAN_POINT('Ctrl Pts',(-2.16122781774006,-3.46851230426945,
-38.1628536518583));
#26224=CARTESIAN_POINT('Ctrl Pts',(-2.26166254517085,-3.40386816266328,
-38.1686606534315));
#26225=CARTESIAN_POINT('Ctrl Pts',(-2.3589862701395,-3.33502755270378,-38.1744676550046));
#26226=CARTESIAN_POINT('Ctrl Pts',(-2.45637483884643,-3.26614107641007,
-38.1802785256003));
#26227=CARTESIAN_POINT('Ctrl Pts',(-2.55064795489363,-3.19305281395483,
-38.186089396196));
#26228=CARTESIAN_POINT('Ctrl Pts',(-2.64143955913574,-3.11609082913717,
-38.1919002667917));
#26229=CARTESIAN_POINT('Ctrl Pts',(-2.73236176628603,-3.0390181351948,-38.1977194962726));
#26230=CARTESIAN_POINT('Ctrl Pts',(-2.81979216729412,-2.95806087447145,
-38.2035387257535));
#26231=CARTESIAN_POINT('Ctrl Pts',(-2.90340189323373,-2.87358355479126,
-38.2093579552345));
#26232=CARTESIAN_POINT('Ctrl Pts',(-2.92417972218139,-2.85259012037265,
-38.2108040902792));
#26233=CARTESIAN_POINT('Ctrl Pts',(-2.94472179518781,-2.83137945338585,
-38.2122502253239));
#26234=CARTESIAN_POINT('Ctrl Pts',(-2.96502346430134,-2.80995744738999,
-38.2136963603687));
#26235=CARTESIAN_POINT('Ctrl Pts',(-3.04596507285138,-2.72454911894286,
-38.2194620191451));
#26236=CARTESIAN_POINT('Ctrl Pts',(-3.12335661032414,-2.63548923203773,
-38.2252276779216));
#26237=CARTESIAN_POINT('Ctrl Pts',(-3.19684629131144,-2.54310809635145,
-38.2309933366981));
#26238=CARTESIAN_POINT('Ctrl Pts',(-3.27022120562092,-2.45087122957331,
-38.2367499914144));
#26239=CARTESIAN_POINT('Ctrl Pts',(-3.33970613289259,-2.35532376030525,
-38.2425066461308));
#26240=CARTESIAN_POINT('Ctrl Pts',(-3.40498643381326,-2.25683237869976,
-38.2482633008472));
#26241=CARTESIAN_POINT('Ctrl Pts',(-3.47020838077286,-2.15842903838954,
-38.2540148096988));
#26242=CARTESIAN_POINT('Ctrl Pts',(-3.53123294188016,-2.05708736147524,
-38.2597663185503));
#26243=CARTESIAN_POINT('Ctrl Pts',(-3.58778614809329,-1.95320648052117,
-38.2655178274018));
#26244=CARTESIAN_POINT('Ctrl Pts',(-3.6443028410371,-1.84939266969164,-38.271265622823));
#26245=CARTESIAN_POINT('Ctrl Pts',(-3.69635371924347,-1.74304327941579,
-38.2770134182442));
#26246=CARTESIAN_POINT('Ctrl Pts',(-3.74370892814126,-1.63458510373593,
-38.2827612136654));
#26247=CARTESIAN_POINT('Ctrl Pts',(-3.79104531624626,-1.52617003353273,
-38.2885067246903));
#26248=CARTESIAN_POINT('Ctrl Pts',(-3.83368958006656,-1.41564822698566,
-38.2942522357151));
#26249=CARTESIAN_POINT('Ctrl Pts',(-3.87145884581187,-1.30346898896177,
-38.29999774674));
#26250=CARTESIAN_POINT('Ctrl Pts',(-3.90923391853051,-1.19127250353233,
-38.3057441411294));
#26251=CARTESIAN_POINT('Ctrl Pts',(-3.94213235272038,-1.07741847010478,
-38.3114905355187));
#26252=CARTESIAN_POINT('Ctrl Pts',(-3.97002039009557,-0.962373681178677,
-38.3172369299081));
#26253=CARTESIAN_POINT('Ctrl Pts',(-3.99790992310238,-0.847322722416304,
-38.3229836324758));
#26254=CARTESIAN_POINT('Ctrl Pts',(-4.0207884337351,-0.731081288926688,
-38.3287303350435));
#26255=CARTESIAN_POINT('Ctrl Pts',(-4.03857306524437,-0.614127508488797,
-38.3344770376112));
#26256=CARTESIAN_POINT('Ctrl Pts',(-4.05637201751117,-0.497079553103854,
-38.3402283676088));
#26257=CARTESIAN_POINT('Ctrl Pts',(-4.06906884303718,-0.379318519535031,
-38.3459796976063));
#26258=CARTESIAN_POINT('Ctrl Pts',(-4.07663246715613,-0.261328773250282,
-38.3517310276038));
#26259=CARTESIAN_POINT('Ctrl Pts',(-4.08228042108977,-0.173222775229081,
-38.356025694601));
#26260=CARTESIAN_POINT('Ctrl Pts',(-4.08506718194844,-0.0849893876783897,
-38.3603203615983));
#26261=CARTESIAN_POINT('Ctrl Pts',(-4.08499877004747,0.0031699701342642,
-38.3646150285955));
#26262=CARTESIAN_POINT('Ctrl Pts',(-4.0847807681364,0.00317176647937747,
-38.3646151243503));
#26263=CARTESIAN_POINT('Ctrl Pts',(-4.08755373173903,0.315568510627117,
-38.3798341729923));
#26264=CARTESIAN_POINT('Ctrl Pts',(-3.91319964322216,1.97007722952994,-38.4605785249371));
#26265=CARTESIAN_POINT('Ctrl Pts',(-1.66658153270677,4.5182208917146,-38.6068481801843));
#26266=CARTESIAN_POINT('Ctrl Pts',(1.37998923899127,4.08193142921117,-38.7392005931756));
#26267=CARTESIAN_POINT('Ctrl Pts',(2.46962553701302,3.26155408523247,-38.8060277028642));
#26268=CARTESIAN_POINT('Ctrl Pts',(2.49067940755052,3.24534996886507,-38.8073295092502));
#26269=CARTESIAN_POINT('',(-4.0849985769777,-0.00340970529112389,-38.2603849714395));
#26270=CARTESIAN_POINT('Ctrl Pts',(-4.0849985769777,-0.0034097052911255,
-38.2603849714395));
#26271=CARTESIAN_POINT('Ctrl Pts',(-4.08509671274173,0.114161879992395,
-38.2661197666967));
#26272=CARTESIAN_POINT('Ctrl Pts',(-4.08011485793121,0.23189389784994,-38.271854561954));
#26273=CARTESIAN_POINT('Ctrl Pts',(-4.07003816185633,0.349305541085676,
-38.2775893572112));
#26274=CARTESIAN_POINT('Ctrl Pts',(-4.05971995163102,0.469531258801339,
-38.2834616017072));
#26275=CARTESIAN_POINT('Ctrl Pts',(-4.04405951039676,0.589420605878094,
-38.2893338462032));
#26276=CARTESIAN_POINT('Ctrl Pts',(-4.02309759022828,0.708456617937449,
-38.2952060906992));
#26277=CARTESIAN_POINT('Ctrl Pts',(-4.00265473465418,0.824545028879237,
-38.3009329251286));
#26278=CARTESIAN_POINT('Ctrl Pts',(-3.97716996340125,0.939821432329227,
-38.306659759558));
#26279=CARTESIAN_POINT('Ctrl Pts',(-3.94673347793783,1.05381205825554,-38.3123865939874));
#26280=CARTESIAN_POINT('Ctrl Pts',(-3.91630400078119,1.1677764366942,-38.3181121097556));
#26281=CARTESIAN_POINT('Ctrl Pts',(-3.88092518400022,1.28045521990363,-38.3238376255238));
#26282=CARTESIAN_POINT('Ctrl Pts',(-3.84073788806712,1.39138688910228,-38.329563141292));
#26283=CARTESIAN_POINT('Ctrl Pts',(-3.80054973343371,1.50232092862857,-38.3352887794));
#26284=CARTESIAN_POINT('Ctrl Pts',(-3.75555303948203,1.61150738475108,-38.3410144175079));
#26285=CARTESIAN_POINT('Ctrl Pts',(-3.70593760765772,1.71850267621212,-38.3467400556158));
#26286=CARTESIAN_POINT('Ctrl Pts',(-3.65410127539669,1.83028732212992,-38.3527219864074));
#26287=CARTESIAN_POINT('Ctrl Pts',(-3.59722330377182,1.93967961846452,-38.358703917199));
#26288=CARTESIAN_POINT('Ctrl Pts',(-3.53557415443047,2.04620145599676,-38.3646858479906));
#26289=CARTESIAN_POINT('Ctrl Pts',(-3.47648681993481,2.14829680544772,-38.3704192011575));
#26290=CARTESIAN_POINT('Ctrl Pts',(-3.41301717942872,2.24775515243283,-38.3761525543244));
#26291=CARTESIAN_POINT('Ctrl Pts',(-3.34544749077826,2.3441855912972,-38.3818859074913));
#26292=CARTESIAN_POINT('Ctrl Pts',(-3.2778339028369,2.44067867996762,-38.3876229855553));
#26293=CARTESIAN_POINT('Ctrl Pts',(-3.20611522154903,2.5341396135903,-38.3933600636193));
#26294=CARTESIAN_POINT('Ctrl Pts',(-3.13061348641048,2.62421115741566,-38.3990971416833));
#26295=CARTESIAN_POINT('Ctrl Pts',(-3.05500788666663,2.71440660892777,-38.4048421120077));
#26296=CARTESIAN_POINT('Ctrl Pts',(-2.9756091358878,2.80120306273816,-38.410587082332));
#26297=CARTESIAN_POINT('Ctrl Pts',(-2.89277540845927,2.8842807485079,-38.4163320526564));
#26298=CARTESIAN_POINT('Ctrl Pts',(-2.8822442845987,2.89484288818278,-38.4170624434759));
#26299=CARTESIAN_POINT('Ctrl Pts',(-2.87165768176318,2.9053449742801,-38.4177928342954));
#26300=CARTESIAN_POINT('Ctrl Pts',(-2.86101637200142,2.91578639806483,-38.418523225115));
#26301=CARTESIAN_POINT('Ctrl Pts',(-2.77624574557761,2.99896469611309,-38.4243416524225));
#26302=CARTESIAN_POINT('Ctrl Pts',(-2.68770713769223,3.07857813632915,-38.43016007973));
#26303=CARTESIAN_POINT('Ctrl Pts',(-2.59573275325813,3.15426639231105,-38.4359785070375));
#26304=CARTESIAN_POINT('Ctrl Pts',(-2.50387419153435,3.22985933459228,-38.4417896072395));
#26305=CARTESIAN_POINT('Ctrl Pts',(-2.408588771664,3.30153666605369,-38.4476007074415));
#26306=CARTESIAN_POINT('Ctrl Pts',(-2.3102457186713,3.36897457980331,-38.4534118076434));
#26307=CARTESIAN_POINT('Ctrl Pts',(-2.21200075442206,3.43634523002979,-38.4592171117724));
#26308=CARTESIAN_POINT('Ctrl Pts',(-2.11070455936081,3.499484644205,-38.4650224159013));
#26309=CARTESIAN_POINT('Ctrl Pts',(-2.00675915609902,3.55810942628424,-38.4708277200303));
#26310=CARTESIAN_POINT('Ctrl Pts',(-1.89912518552784,3.61881454523179,-38.4768390289883));
#26311=CARTESIAN_POINT('Ctrl Pts',(-1.78865084348428,3.67467839039533,-38.4828503379463));
#26312=CARTESIAN_POINT('Ctrl Pts',(-1.67581533584916,3.72543527123111,-38.4888616469043));
#26313=CARTESIAN_POINT('Ctrl Pts',(-1.56696765723321,3.77439830395504,-38.4946605043672));
#26314=CARTESIAN_POINT('Ctrl Pts',(-1.45592328864224,3.81860906005878,-38.50045936183));
#26315=CARTESIAN_POINT('Ctrl Pts',(-1.34313649121172,3.85787627665474,-38.5062582192929));
#26316=CARTESIAN_POINT('Ctrl Pts',(-1.23036562846781,3.8971379455199,-38.5120562574845));
#26317=CARTESIAN_POINT('Ctrl Pts',(-1.1158532126979,3.93145732928513,-38.5178542956761));
#26318=CARTESIAN_POINT('Ctrl Pts',(-1.00007130982692,3.96069215860827,-38.5236523338678));
#26319=CARTESIAN_POINT('Ctrl Pts',(-0.884278311697346,3.98992978947452,
-38.5294509276793));
#26320=CARTESIAN_POINT('Ctrl Pts',(-0.767215981280507,4.01408179697358,
-38.5352495214909));
#26321=CARTESIAN_POINT('Ctrl Pts',(-0.649368654361985,4.03305657668376,
-38.5410481153024));
#26322=CARTESIAN_POINT('Ctrl Pts',(-0.531482091484585,4.05203767383613,
-38.5468486396914));
#26323=CARTESIAN_POINT('Ctrl Pts',(-0.412810416039433,4.0658380502612,-38.5526491640804));
#26324=CARTESIAN_POINT('Ctrl Pts',(-0.293844544922322,4.07441779686612,
-38.5584496884694));
#26325=CARTESIAN_POINT('Ctrl Pts',(-0.174745564709313,4.08300714321846,
-38.5642567029765));
#26326=CARTESIAN_POINT('Ctrl Pts',(-0.0553521400692684,4.08636417104349,
-38.5700637174836));
#26327=CARTESIAN_POINT('Ctrl Pts',(0.0638431898660881,4.08450107688904,
-38.5758707319907));
#26328=CARTESIAN_POINT('Ctrl Pts',(0.18311793397613,4.08263674144363,-38.5816816154352));
#26329=CARTESIAN_POINT('Ctrl Pts',(0.302193913172875,4.07554538240647,-38.5874924988797));
#26330=CARTESIAN_POINT('Ctrl Pts',(0.420583764816697,4.06329106719819,-38.5933033823241));
#26331=CARTESIAN_POINT('Ctrl Pts',(0.539143914326865,4.05101912477183,-38.5991226244331));
#26332=CARTESIAN_POINT('Ctrl Pts',(0.657015563335642,4.0335694636176,-38.6049418665421));
#26333=CARTESIAN_POINT('Ctrl Pts',(0.773721465431621,4.01105722895228,-38.6107611086511));
#26334=CARTESIAN_POINT('Ctrl Pts',(0.802721420611276,4.00546322055542,-38.6122071174416));
#26335=CARTESIAN_POINT('Ctrl Pts',(0.831649470699675,3.99955685873833,-38.6136531262322));
#26336=CARTESIAN_POINT('Ctrl Pts',(0.860498453699164,3.99334038258465,-38.6150991350227));
#26337=CARTESIAN_POINT('Ctrl Pts',(0.976932508413389,3.96825077978584,-38.6209352044134));
#26338=CARTESIAN_POINT('Ctrl Pts',(1.09245176881673,3.93802512916553,-38.6267712738042));
#26339=CARTESIAN_POINT('Ctrl Pts',(1.20657033769348,3.90274429346815,-38.6326073431949));
#26340=CARTESIAN_POINT('Ctrl Pts',(1.32151675195873,3.86720752153339,-38.6384857489308));
#26341=CARTESIAN_POINT('Ctrl Pts',(1.43504165260818,3.82654194086775,-38.6443641546668));
#26342=CARTESIAN_POINT('Ctrl Pts',(1.54665721385476,3.78088302686436,-38.6502425604028));
#26343=CARTESIAN_POINT('Ctrl Pts',(1.65720292447244,3.73566175988184,-38.6560646208048));
#26344=CARTESIAN_POINT('Ctrl Pts',(1.76587534697202,3.68554260494187,-38.6618866812068));
#26345=CARTESIAN_POINT('Ctrl Pts',(1.87221503303746,3.63070735120149,-38.6677087416088));
#26346=CARTESIAN_POINT('Ctrl Pts',(1.9800984368018,3.57507606208754,-38.6736153200117));
#26347=CARTESIAN_POINT('Ctrl Pts',(2.08558043486308,3.51459078972929,-38.6795218984147));
#26348=CARTESIAN_POINT('Ctrl Pts',(2.18820258457837,3.44949191169432,-38.6854284768176));
#26349=CARTESIAN_POINT('Ctrl Pts',(2.29082473429369,3.38439303365934,-38.6913350552206));
#26350=CARTESIAN_POINT('Ctrl Pts',(2.39058665078402,3.31468076050162,-38.6972416336235));
#26351=CARTESIAN_POINT('Ctrl Pts',(2.48705727606859,3.24064362520075,-38.7031482120265));
#26352=CARTESIAN_POINT('Ctrl Pts',(2.48705727606859,3.24064362520075,-37.4531876190354));
#26353=CARTESIAN_POINT('Ctrl Pts',(2.58154277521058,3.16812999047195,-37.4590058394181));
#26354=CARTESIAN_POINT('Ctrl Pts',(2.67297790338995,3.09138577162844,-37.4648240598007));
#26355=CARTESIAN_POINT('Ctrl Pts',(2.76096338435899,3.01069862162073,-37.4706422801834));
#26356=CARTESIAN_POINT('Ctrl Pts',(2.84886139384849,2.93009168739763,-37.4764547163351));
#26357=CARTESIAN_POINT('Ctrl Pts',(2.93331627983204,2.84554989453595,-37.4822671524868));
#26358=CARTESIAN_POINT('Ctrl Pts',(3.01396078333165,2.75740192872546,-37.4880795886384));
#26359=CARTESIAN_POINT('Ctrl Pts',(3.09728856948325,2.66632101773949,-37.4940854218403));
#26360=CARTESIAN_POINT('Ctrl Pts',(3.17654763178238,2.57139004090815,-37.5000912550422));
#26361=CARTESIAN_POINT('Ctrl Pts',(3.25137283605238,2.47301429049262,-37.5060970882441));
#26362=CARTESIAN_POINT('Ctrl Pts',(3.32370804148694,2.37791224318769,-37.5119030620828));
#26363=CARTESIAN_POINT('Ctrl Pts',(3.39189952608906,2.27959139420542,-37.5177090359214));
#26364=CARTESIAN_POINT('Ctrl Pts',(3.45565796493207,2.17845198005408,-37.5235150097601));
#26365=CARTESIAN_POINT('Ctrl Pts',(3.51940720336462,2.07732716042766,-37.5293201457905));
#26366=CARTESIAN_POINT('Ctrl Pts',(3.57872445071442,1.97338492955952,-37.535125281821));
#26367=CARTESIAN_POINT('Ctrl Pts',(3.63336409647446,1.86705392060603,-37.5409304178515));
#26368=CARTESIAN_POINT('Ctrl Pts',(3.6880087263778,1.76071321230367,-37.5467360834174));
#26369=CARTESIAN_POINT('Ctrl Pts',(3.73797471985586,1.65198365558448,-37.5525417489833));
#26370=CARTESIAN_POINT('Ctrl Pts',(3.78306305086862,1.54131727854866,-37.5583474145493));
#26371=CARTESIAN_POINT('Ctrl Pts',(3.82816611386769,1.43061474281022,-37.5641549770358));
#26372=CARTESIAN_POINT('Ctrl Pts',(3.86838819097253,1.31797450582789,-37.5699625395224));
#26373=CARTESIAN_POINT('Ctrl Pts',(3.90357912415473,1.20386669588595,-37.5757701020089));
#26374=CARTESIAN_POINT('Ctrl Pts',(3.9388088432354,1.08963312133563,-37.5815840653354));
#26375=CARTESIAN_POINT('Ctrl Pts',(3.96899622984037,0.973929135335255,-37.5873980286619));
#26376=CARTESIAN_POINT('Ctrl Pts',(3.9940415137324,0.857238232104843,-37.5932119919883));
#26377=CARTESIAN_POINT('Ctrl Pts',(4.01910328721948,0.74047050060809,-37.5990297831772));
#26378=CARTESIAN_POINT('Ctrl Pts',(4.03901614768469,0.622714959157353,-37.6048475743661));
#26379=CARTESIAN_POINT('Ctrl Pts',(4.05373201773169,0.50446182057411,-37.6106653655549));
#26380=CARTESIAN_POINT('Ctrl Pts',(4.06846872001307,0.386041279241938,-37.6164913925864));
#26381=CARTESIAN_POINT('Ctrl Pts',(4.07799371587268,0.267122140066809,-37.6223174196179));
#26382=CARTESIAN_POINT('Ctrl Pts',(4.08231096862841,0.14819634076506,-37.6281434466494));
#26383=CARTESIAN_POINT('Ctrl Pts',(4.08331781380324,0.120461141099069,-37.6295021595941));
#26384=CARTESIAN_POINT('Ctrl Pts',(4.08404163839779,0.0927255626395004,
-37.6308608725389));
#26385=CARTESIAN_POINT('Ctrl Pts',(4.08448289814634,0.0649958056342169,
-37.6322195854837));
#26386=CARTESIAN_POINT('Ctrl Pts',(4.08637487043928,-0.0538999969310756,
-37.6380452862279));
#26387=CARTESIAN_POINT('Ctrl Pts',(4.08307412858401,-0.173068543203549,
-37.6438709869722));
#26388=CARTESIAN_POINT('Ctrl Pts',(4.074548991457,-0.29201971888346,-37.6496966877164));
#26389=CARTESIAN_POINT('Ctrl Pts',(4.06603455151596,-0.410821636806022,
-37.655515078478));
#26390=CARTESIAN_POINT('Ctrl Pts',(4.0523087841991,-0.529406323247199,-37.6613334692396));
#26391=CARTESIAN_POINT('Ctrl Pts',(4.03339198666198,-0.647282072925641,
-37.6671518600013));
#26392=CARTESIAN_POINT('Ctrl Pts',(4.01449400599587,-0.765040569524009,
-37.6729644631073));
#26393=CARTESIAN_POINT('Ctrl Pts',(3.99041533198627,-0.882091131739768,
-37.6787770662134));
#26394=CARTESIAN_POINT('Ctrl Pts',(3.96122814319716,-0.997946189703017,
-37.6845896693194));
#26395=CARTESIAN_POINT('Ctrl Pts',(3.93105690298246,-1.11770732220375,-37.6905982454058));
#26396=CARTESIAN_POINT('Ctrl Pts',(3.89542662395564,-1.23619046982341,-37.6966068214921));
#26397=CARTESIAN_POINT('Ctrl Pts',(3.85447479376822,-1.35286697949408,-37.7026153975784));
#26398=CARTESIAN_POINT('Ctrl Pts',(3.81490273676214,-1.46561235548406,-37.7084215291805));
#26399=CARTESIAN_POINT('Ctrl Pts',(3.77036209205679,-1.57667045762548,-37.7142276607826));
#26400=CARTESIAN_POINT('Ctrl Pts',(3.72102769838095,-1.68557938640747,-37.7200337923846));
#26401=CARTESIAN_POINT('Ctrl Pts',(3.67170044924306,-1.79447254315057,-37.7258390831508));
#26402=CARTESIAN_POINT('Ctrl Pts',(3.61758100007945,-1.90121677399024,-37.731644373917));
#26403=CARTESIAN_POINT('Ctrl Pts',(3.55889196242682,-2.00537103793133,-37.7374496646833));
#26404=CARTESIAN_POINT('Ctrl Pts',(3.50019760378482,-2.10953474492607,-37.743255481781));
#26405=CARTESIAN_POINT('Ctrl Pts',(3.43693303321699,-2.21110766270125,-37.7490612988787));
#26406=CARTESIAN_POINT('Ctrl Pts',(3.36936604001376,-2.3096747581428,-37.7548671159764));
#26407=CARTESIAN_POINT('Ctrl Pts',(3.30177701017516,-2.40827400074732,-37.7606748266122));
#26408=CARTESIAN_POINT('Ctrl Pts',(3.22988299753557,-2.50386513500164,-37.766482537248));
#26409=CARTESIAN_POINT('Ctrl Pts',(3.15399380660111,-2.59606395682422,-37.7722902478838));
#26410=CARTESIAN_POINT('Ctrl Pts',(3.07802099064959,-2.68836437583018,-37.778104358244));
#26411=CARTESIAN_POINT('Ctrl Pts',(2.99804446836205,-2.77726470579389,-37.7839184686041));
#26412=CARTESIAN_POINT('Ctrl Pts',(2.91441294484785,-2.86241544624523,-37.7897325789642));
#26413=CARTESIAN_POINT('Ctrl Pts',(2.83072640909019,-2.94762219827053,-37.7955505138063));
#26414=CARTESIAN_POINT('Ctrl Pts',(2.74338038160107,-3.02907417109918,-37.8013684486484));
#26415=CARTESIAN_POINT('Ctrl Pts',(2.65275763747355,-3.10646131745202,-37.8071863834905));
#26416=CARTESIAN_POINT('Ctrl Pts',(2.56200653012263,-3.18395807937268,-37.8130125591874));
#26417=CARTESIAN_POINT('Ctrl Pts',(2.46796976304001,-3.25737827314531,-37.8188387348842));
#26418=CARTESIAN_POINT('Ctrl Pts',(2.37106020636012,-3.32645434326334,-37.824664910581));
#26419=CARTESIAN_POINT('Ctrl Pts',(2.34815821120167,-3.34277863446439,-37.8260417721845));
#26420=CARTESIAN_POINT('Ctrl Pts',(2.32509588605495,-3.35886051195241,-37.827418633788));
#26421=CARTESIAN_POINT('Ctrl Pts',(2.30187887847011,-3.3746968202867,-37.8287954953914));
#26422=CARTESIAN_POINT('Ctrl Pts',(2.20366461610006,-3.44168871560456,-37.8346199947924));
#26423=CARTESIAN_POINT('Ctrl Pts',(2.10236600254592,-3.5044969101477,-37.8404444941933));
#26424=CARTESIAN_POINT('Ctrl Pts',(1.99837463052913,-3.56282526038783,-37.8462689935943));
#26425=CARTESIAN_POINT('Ctrl Pts',(1.89451383237716,-3.62108037226238,-37.8520861796251));
#26426=CARTESIAN_POINT('Ctrl Pts',(1.78796735364336,-3.67486663002221,-37.8579033656559));
#26427=CARTESIAN_POINT('Ctrl Pts',(1.67915672955179,-3.72393040719089,-37.8637205516867));
#26428=CARTESIAN_POINT('Ctrl Pts',(1.57045439961708,-3.77294535346254,-37.8695319481426));
#26429=CARTESIAN_POINT('Ctrl Pts',(1.45949277722068,-3.81724700264141,-37.8753433445985));
#26430=CARTESIAN_POINT('Ctrl Pts',(1.34671850405785,-3.85662731811465,-37.8811547410544));
#26431=CARTESIAN_POINT('Ctrl Pts',(1.23010905677329,-3.89734686072341,-37.8871637687312));
#26432=CARTESIAN_POINT('Ctrl Pts',(1.11156186213879,-3.93280416329357,-37.8931727964081));
#26433=CARTESIAN_POINT('Ctrl Pts',(0.991594234988161,-3.96282296767572,
-37.899181824085));
#26434=CARTESIAN_POINT('Ctrl Pts',(0.875701372069739,-3.99182216740873,
-37.9049867519423));
#26435=CARTESIAN_POINT('Ctrl Pts',(0.75848342851756,-4.01574620389473,-37.9107916797997));
#26436=CARTESIAN_POINT('Ctrl Pts',(0.640422122693153,-4.03448689485605,
-37.9165966076571));
#26437=CARTESIAN_POINT('Ctrl Pts',(0.522377853573187,-4.05322488146296,
-37.9224006978408));
#26438=CARTESIAN_POINT('Ctrl Pts',(0.403490867224466,-4.06678094610007,
-37.9282047880246));
#26439=CARTESIAN_POINT('Ctrl Pts',(0.284251756357326,-4.07509827353989,
-37.9340088782083));
#26440=CARTESIAN_POINT('Ctrl Pts',(0.16500174082723,-4.08341636161648,-37.9398134991881));
#26441=CARTESIAN_POINT('Ctrl Pts',(0.0453999439464807,-4.08649473153917,
-37.9456181201679));
#26442=CARTESIAN_POINT('Ctrl Pts',(-0.0740598973889684,-4.08432860230402,
-37.9514227411477));
#26443=CARTESIAN_POINT('Ctrl Pts',(-0.193558826744508,-4.08216176429761,
-37.9572292614364));
#26444=CARTESIAN_POINT('Ctrl Pts',(-0.312915300296527,-4.07474702170451,
-37.9630357817251));
#26445=CARTESIAN_POINT('Ctrl Pts',(-0.431638205376883,-4.06213163987321,
-37.9688423020138));
#26446=CARTESIAN_POINT('Ctrl Pts',(-0.550492257931542,-4.04950232243729,
-37.9746552364858));
#26447=CARTESIAN_POINT('Ctrl Pts',(-0.668710938938595,-4.03166094186888,
-37.9804681709578));
#26448=CARTESIAN_POINT('Ctrl Pts',(-0.785810709842292,-4.00870634099046,
-37.9862811054297));
#26449=CARTESIAN_POINT('Ctrl Pts',(-0.902987666627895,-3.98573660967158,
-37.992097871476));
#26450=CARTESIAN_POINT('Ctrl Pts',(-1.01904384872924,-3.95764704165268,
-37.9979146375223));
#26451=CARTESIAN_POINT('Ctrl Pts',(-1.13350992009048,-3.92458663569254,
-38.0037314035685));
#26452=CARTESIAN_POINT('Ctrl Pts',(-1.24813853611653,-3.89147928313467,
-38.0095564295671));
#26453=CARTESIAN_POINT('Ctrl Pts',(-1.36117214939061,-3.85338713429346,
-38.0153814555656));
#26454=CARTESIAN_POINT('Ctrl Pts',(-1.47216035055477,-3.81050769612849,
-38.0212064815642));
#26455=CARTESIAN_POINT('Ctrl Pts',(-1.49861272996384,-3.80028802272816,
-38.0225947894759));
#26456=CARTESIAN_POINT('Ctrl Pts',(-1.52494902998922,-3.78979662071743,
-38.0239830973876));
#26457=CARTESIAN_POINT('Ctrl Pts',(-1.55116336329753,-3.77903654657685,
-38.0253714052993));
#26458=CARTESIAN_POINT('Ctrl Pts',(-1.66118149265029,-3.73387792229598,
-38.0311979520825));
#26459=CARTESIAN_POINT('Ctrl Pts',(-1.76940169440656,-3.68383878208755,
-38.0370244988657));
#26460=CARTESIAN_POINT('Ctrl Pts',(-1.87536099697052,-3.62908337339358,
-38.0428510456488));
#26461=CARTESIAN_POINT('Ctrl Pts',(-1.98118724980554,-3.57439671932623,
-38.0486702762224));
#26462=CARTESIAN_POINT('Ctrl Pts',(-2.0847578910019,-3.51500576157751,-38.0544895067959));
#26463=CARTESIAN_POINT('Ctrl Pts',(-2.18562898961654,-3.45112313888505,
-38.0603087373695));
#26464=CARTESIAN_POINT('Ctrl Pts',(-2.28639964077916,-3.38730413051587,
-38.0661221731525));
#26465=CARTESIAN_POINT('Ctrl Pts',(-2.38447575474482,-3.31900257252095,
-38.0719356089356));
#26466=CARTESIAN_POINT('Ctrl Pts',(-2.47943766369157,-3.24647714790474,
-38.0777490447186));
#26467=CARTESIAN_POINT('Ctrl Pts',(-2.57758202805301,-3.17152118105499,
-38.083757305989));
#26468=CARTESIAN_POINT('Ctrl Pts',(-2.67239939373545,-3.09205346904024,
-38.0897655672593));
#26469=CARTESIAN_POINT('Ctrl Pts',(-2.76345833598413,-3.00840871978523,
-38.0957738285297));
#26470=CARTESIAN_POINT('Ctrl Pts',(-2.8514661510376,-2.92756666912177,-38.1015807699856));
#26471=CARTESIAN_POINT('Ctrl Pts',(-2.93596305295684,-2.84282331723503,
-38.1073877114415));
#26472=CARTESIAN_POINT('Ctrl Pts',(-3.01659344417503,-2.75452155420143,
-38.1131946528974));
#26473=CARTESIAN_POINT('Ctrl Pts',(-3.09721202408886,-2.66623272622844,
-38.1190007437118));
#26474=CARTESIAN_POINT('Ctrl Pts',(-3.17396494479635,-2.57438682488607,
-38.1248068345263));
#26475=CARTESIAN_POINT('Ctrl Pts',(-3.24653461441266,-2.47936241752198,
-38.1306129253407));
#26476=CARTESIAN_POINT('Ctrl Pts',(-3.31911072960496,-2.38432957017129,
-38.1364195318472));
#26477=CARTESIAN_POINT('Ctrl Pts',(-3.38750260742348,-2.28611797965193,
-38.1422261383537));
#26478=CARTESIAN_POINT('Ctrl Pts',(-3.45143436962128,-2.18513747672703,
-38.1480327448601));
#26479=CARTESIAN_POINT('Ctrl Pts',(-3.51538685359213,-2.08412424366937,
-38.153841233423));
#26480=CARTESIAN_POINT('Ctrl Pts',(-3.57487612881596,-1.98034065773014,
-38.1596497219859));
#26481=CARTESIAN_POINT('Ctrl Pts',(-3.62967121358454,-1.87422300734884,
-38.1654582105487));
#26482=CARTESIAN_POINT('Ctrl Pts',(-3.68452647523737,-1.76798881677802,
-38.1712730780915));
#26483=CARTESIAN_POINT('Ctrl Pts',(-3.7346770690846,-1.65941580786129,-38.1770879456343));
#26484=CARTESIAN_POINT('Ctrl Pts',(-3.77993924292916,-1.54896233645757,
-38.182902813177));
#26485=CARTESIAN_POINT('Ctrl Pts',(-3.82523109851871,-1.43843643256791,
-38.1887214939572));
#26486=CARTESIAN_POINT('Ctrl Pts',(-3.86562801207002,-1.32602799318487,
-38.1945401747374));
#26487=CARTESIAN_POINT('Ctrl Pts',(-3.90099591993381,-1.21221113369731,
-38.2003588555176));
#26488=CARTESIAN_POINT('Ctrl Pts',(-3.93641378552208,-1.09823350611097,
-38.2061857552756));
#26489=CARTESIAN_POINT('Ctrl Pts',(-3.96678836416692,-0.982843880774551,
-38.2120126550337));
#26490=CARTESIAN_POINT('Ctrl Pts',(-3.99203650673829,-0.866527281087397,
-38.2178395547917));
#26491=CARTESIAN_POINT('Ctrl Pts',(-3.99796952572057,-0.839194237005159,
-38.2192088082635));
#26492=CARTESIAN_POINT('Ctrl Pts',(-4.00361969092606,-0.811810029377355,
-38.2205780617353));
#26493=CARTESIAN_POINT('Ctrl Pts',(-4.00898633942689,-0.784380985420102,
-38.2219473152071));
#26494=CARTESIAN_POINT('Ctrl Pts',(-4.04160802073748,-0.617650943292322,
-38.2302704521488));
#26495=CARTESIAN_POINT('Ctrl Pts',(-4.06383608673867,-0.448826534878653,
-38.2385935890905));
#26496=CARTESIAN_POINT('Ctrl Pts',(-4.07546276612986,-0.278977135065131,
-38.2469167260322));
#26497=CARTESIAN_POINT('Ctrl Pts',(-4.08173407833672,-0.187362102213624,
-38.2514061411563));
#26498=CARTESIAN_POINT('Ctrl Pts',(-4.0849217525647,-0.0954491999141607,
-38.2558955562804));
#26499=CARTESIAN_POINT('Ctrl Pts',(-4.0849985769771,-0.00340970600798366,
-38.2603849714045));
#26500=CARTESIAN_POINT('Origin',(0.,0.,-25.2396150285955));
#26501=CARTESIAN_POINT('',(2.4870572760686,3.24064362520075,-36.2030038303486));
#26502=CARTESIAN_POINT('',(2.4870572760686,3.24064362520075,-36.3074370930634));
#26503=CARTESIAN_POINT('',(2.4870572760686,3.24064362520075,-25.2396150285955));
#26504=CARTESIAN_POINT('',(-4.08499957977947,-0.00185289005459989,-37.1146150285588));
#26505=CARTESIAN_POINT('Ctrl Pts',(2.4870572760686,3.24064362520075,-36.3074370930634));
#26506=CARTESIAN_POINT('Ctrl Pts',(2.58180014386427,3.16793247088731,-36.3132441745903));
#26507=CARTESIAN_POINT('Ctrl Pts',(2.67341078999859,3.09101770294433,-36.3190512561171));
#26508=CARTESIAN_POINT('Ctrl Pts',(2.76150160643884,3.0102049560845,-36.324858337644));
#26509=CARTESIAN_POINT('Ctrl Pts',(2.84956668578501,2.9294158199182,-36.3306637225421));
#26510=CARTESIAN_POINT('Ctrl Pts',(2.93411367992539,2.84473124498611,-36.3364691074403));
#26511=CARTESIAN_POINT('Ctrl Pts',(3.01478912421968,2.7564962427848,-36.3422744923385));
#26512=CARTESIAN_POINT('Ctrl Pts',(3.09546000078508,2.6682662363238,-36.3480795485441));
#26513=CARTESIAN_POINT('Ctrl Pts',(3.1722594882483,2.57648650359193,-36.3538846047496));
#26514=CARTESIAN_POINT('Ctrl Pts',(3.24487241507926,2.48153742866347,-36.3596896609552));
#26515=CARTESIAN_POINT('Ctrl Pts',(3.31749833426117,2.38657136486322,-36.365495755837));
#26516=CARTESIAN_POINT('Ctrl Pts',(3.38593595537108,2.28843515528463,-36.3713018507189));
#26517=CARTESIAN_POINT('Ctrl Pts',(3.44991206848321,2.18754010700007,-36.3771079456008));
#26518=CARTESIAN_POINT('Ctrl Pts',(3.51395407662326,2.08654113739707,-36.3829200207269));
#26519=CARTESIAN_POINT('Ctrl Pts',(3.573525179289,1.9827779985427,-36.3887320958531));
#26520=CARTESIAN_POINT('Ctrl Pts',(3.62839686054799,1.87668889866314,-36.3945441709792));
#26521=CARTESIAN_POINT('Ctrl Pts',(3.68329739593559,1.77054401211074,-36.4003593023697));
#26522=CARTESIAN_POINT('Ctrl Pts',(3.73349341497927,1.66207109787077,-36.4061744337602));
#26523=CARTESIAN_POINT('Ctrl Pts',(3.77880425461889,1.55172916621239,-36.4119895651507));
#26524=CARTESIAN_POINT('Ctrl Pts',(3.82418714418058,1.44121177703344,-36.4178139433299));
#26525=CARTESIAN_POINT('Ctrl Pts',(3.86466919502848,1.32881981642843,-36.4236383215092));
#26526=CARTESIAN_POINT('Ctrl Pts',(3.90011921975187,1.21502883575743,-36.4294626996885));
#26527=CARTESIAN_POINT('Ctrl Pts',(3.93065407232591,1.11701505872468,-36.4344795235251));
#26528=CARTESIAN_POINT('Ctrl Pts',(3.95745634301611,1.01796369683905,-36.4394963473616));
#26529=CARTESIAN_POINT('Ctrl Pts',(3.98047278670977,0.918183747548924,-36.4445131711982));
#26530=CARTESIAN_POINT('Ctrl Pts',(4.00719913262867,0.802320781228317,-36.4503386310762));
#26531=CARTESIAN_POINT('Ctrl Pts',(4.02890525524872,0.685104581897241,-36.4561640909541));
#26532=CARTESIAN_POINT('Ctrl Pts',(4.0454576034012,0.567007741643311,-36.4619895508321));
#26533=CARTESIAN_POINT('Ctrl Pts',(4.06198917531036,0.449059134659096,-36.4678076986857));
#26534=CARTESIAN_POINT('Ctrl Pts',(4.07337978343739,0.330232485900519,-36.4736258465394));
#26535=CARTESIAN_POINT('Ctrl Pts',(4.07954637044436,0.211012822819462,-36.479443994393));
#26536=CARTESIAN_POINT('Ctrl Pts',(4.08570682135357,0.0919117899477465,
-36.4852563528653));
#26537=CARTESIAN_POINT('Ctrl Pts',(4.08665357156166,-0.0275810740777785,
-36.4910687113376));
#26538=CARTESIAN_POINT('Ctrl Pts',(4.08235516152713,-0.146973926778875,
-36.4968810698099));
#26539=CARTESIAN_POINT('Ctrl Pts',(4.07791157546125,-0.270399196207944,
-36.5028897369472));
#26540=CARTESIAN_POINT('Ctrl Pts',(4.06786219252625,-0.393717139271351,
-36.5088984040845));
#26541=CARTESIAN_POINT('Ctrl Pts',(4.05223082381314,-0.516381981229635,
-36.5149070712219));
#26542=CARTESIAN_POINT('Ctrl Pts',(4.0371269886833,-0.634907081825153,-36.5207129554959));
#26543=CARTESIAN_POINT('Ctrl Pts',(4.01681191031066,-0.752822015257029,
-36.5265188397699));
#26544=CARTESIAN_POINT('Ctrl Pts',(3.99135989129911,-0.86963855602702,-36.5323247240439));
#26545=CARTESIAN_POINT('Ctrl Pts',(3.96591156081907,-0.986438167629546,
-36.5381297669235));
#26546=CARTESIAN_POINT('Ctrl Pts',(3.93532785707022,-1.1021393045834,-36.543934809803));
#26547=CARTESIAN_POINT('Ctrl Pts',(3.89973416268372,-1.21626414088285,-36.5497398526826));
#26548=CARTESIAN_POINT('Ctrl Pts',(3.86413724282331,-1.33039931908943,-36.5555454216108));
#26549=CARTESIAN_POINT('Ctrl Pts',(3.82352955114842,-1.44295752310767,-36.561350990539));
#26550=CARTESIAN_POINT('Ctrl Pts',(3.77808609014614,-1.55347690534629,-36.5671565594672));
#26551=CARTESIAN_POINT('Ctrl Pts',(3.7326278074101,-1.66403233433007,-36.5729640219263));
#26552=CARTESIAN_POINT('Ctrl Pts',(3.68233077364905,-1.77254724186748,-36.5787714843854));
#26553=CARTESIAN_POINT('Ctrl Pts',(3.62741752731441,-1.87858113546693,-36.5845789468445));
#26554=CARTESIAN_POINT('Ctrl Pts',(3.57244375577298,-1.98473189928922,-36.5903928102703));
#26555=CARTESIAN_POINT('Ctrl Pts',(3.5128438035658,-2.08839582834566,-36.5962066736962));
#26556=CARTESIAN_POINT('Ctrl Pts',(3.44888551003451,-2.18915822604808,-36.6020205371221));
#26557=CARTESIAN_POINT('Ctrl Pts',(3.38488513850607,-2.28998691507333,-36.6078382254738));
#26558=CARTESIAN_POINT('Ctrl Pts',(3.31652094819986,-2.38790993727525,-36.6136559138255));
#26559=CARTESIAN_POINT('Ctrl Pts',(3.24410234899087,-2.48254404780095,-36.6194736021772));
#26560=CARTESIAN_POINT('Ctrl Pts',(3.17158113638138,-2.5773122499549,-36.6252995338917));
#26561=CARTESIAN_POINT('Ctrl Pts',(3.0949943098072,-2.6687819275656,-36.6311254656062));
#26562=CARTESIAN_POINT('Ctrl Pts',(3.0146895983794,-2.75660509058208,-36.6369513973206));
#26563=CARTESIAN_POINT('Ctrl Pts',(2.9956783043551,-2.77739629877603,-36.6383306252491));
#26564=CARTESIAN_POINT('Ctrl Pts',(2.97645879095806,-2.79798330888898,-36.6397098531776));
#26565=CARTESIAN_POINT('Ctrl Pts',(2.95703594603752,-2.81836183160395,-36.6410890811061));
#26566=CARTESIAN_POINT('Ctrl Pts',(2.87499899282679,-2.90443531472711,-36.6469145746163));
#26567=CARTESIAN_POINT('Ctrl Pts',(2.78906955788716,-2.98706160281669,-36.6527400681266));
#26568=CARTESIAN_POINT('Ctrl Pts',(2.6995687634409,-3.06586912497161,-36.6585655616368));
#26569=CARTESIAN_POINT('Ctrl Pts',(2.6101803029062,-3.14457773451599,-36.6643837434749));
#26570=CARTESIAN_POINT('Ctrl Pts',(2.5172297021419,-3.21947684419097,-36.6702019253129));
#26571=CARTESIAN_POINT('Ctrl Pts',(2.4210762519493,-3.29023020201431,-36.6760201071509));
#26572=CARTESIAN_POINT('Ctrl Pts',(2.32501847416656,-3.36091316044756,-36.6818324999145));
#26573=CARTESIAN_POINT('Ctrl Pts',(2.22576451365462,-3.4274583329537,-36.6876448926782));
#26574=CARTESIAN_POINT('Ctrl Pts',(2.12370774441464,-3.48956880091413,-36.6934572854418));
#26575=CARTESIAN_POINT('Ctrl Pts',(2.01820491961201,-3.55377649500867,-36.6994659398406));
#26576=CARTESIAN_POINT('Ctrl Pts',(1.90970699030915,-3.61324440640284,-36.7054745942395));
#26577=CARTESIAN_POINT('Ctrl Pts',(1.79868276597447,-3.66769209549908,-36.7114832486383));
#26578=CARTESIAN_POINT('Ctrl Pts',(1.69140455987633,-3.72030268969541,-36.7172891677414));
#26579=CARTESIAN_POINT('Ctrl Pts',(1.58176818138103,-3.76822617288067,-36.7230950868445));
#26580=CARTESIAN_POINT('Ctrl Pts',(1.47022218216631,-3.81125592620938,-36.7289010059476));
#26581=CARTESIAN_POINT('Ctrl Pts',(1.35869234558041,-3.85427944467592,-36.7347060837931));
#26582=CARTESIAN_POINT('Ctrl Pts',(1.24525381912777,-3.8924104966771,-36.7405111616386));
#26583=CARTESIAN_POINT('Ctrl Pts',(1.13037457912866,-3.92549083693488,-36.7463162394842));
#26584=CARTESIAN_POINT('Ctrl Pts',(1.01548492698741,-3.95857417544722,-36.7521218434761));
#26585=CARTESIAN_POINT('Ctrl Pts',(0.899154693770183,-3.98660577914462,
-36.757927447468));
#26586=CARTESIAN_POINT('Ctrl Pts',(0.781865818708626,-4.00947762701516,
-36.7637330514599));
#26587=CARTESIAN_POINT('Ctrl Pts',(0.664538688028052,-4.03235693490011,
-36.7695405490412));
#26588=CARTESIAN_POINT('Ctrl Pts',(0.546252693907931,-4.05007306188573,
-36.7753480466226));
#26589=CARTESIAN_POINT('Ctrl Pts',(0.427498102411096,-4.06256942986024,
-36.7811555442039));
#26590=CARTESIAN_POINT('Ctrl Pts',(0.308612622638982,-4.0750795710121,-36.7869694426606));
#26591=CARTESIAN_POINT('Ctrl Pts',(0.189257920571902,-4.0823584270099,-36.7927833411173));
#26592=CARTESIAN_POINT('Ctrl Pts',(0.0699276512532866,-4.08440144006318,
-36.7985972395741));
#26593=CARTESIAN_POINT('Ctrl Pts',(-0.0494811243941398,-4.08644579719668,
-36.8044149629432));
#26594=CARTESIAN_POINT('Ctrl Pts',(-0.168865028371516,-4.08324746214124,
-36.8102326863123));
#26595=CARTESIAN_POINT('Ctrl Pts',(-0.287733791801261,-4.07485389493362,
-36.8160504096814));
#26596=CARTESIAN_POINT('Ctrl Pts',(-0.406770979274152,-4.06644843495884,
-36.8218763761285));
#26597=CARTESIAN_POINT('Ctrl Pts',(-0.525291165562446,-4.05283309748878,
-36.8277023425756));
#26598=CARTESIAN_POINT('Ctrl Pts',(-0.642812432542545,-4.0341067383708,
-36.8335283090228));
#26599=CARTESIAN_POINT('Ctrl Pts',(-0.670627451910066,-4.02967457000729,
-36.8349072030198));
#26600=CARTESIAN_POINT('Ctrl Pts',(-0.698386574971191,-4.02495631525664,
-36.8362860970168));
#26601=CARTESIAN_POINT('Ctrl Pts',(-0.726083535138221,-4.0199536937633,
-36.8376649910139));
#26602=CARTESIAN_POINT('Ctrl Pts',(-0.843093124115286,-3.99881943638582,
-36.8434903169291));
#26603=CARTESIAN_POINT('Ctrl Pts',(-0.959366434350854,-3.97253839256482,
-36.8493156428444));
#26604=CARTESIAN_POINT('Ctrl Pts',(-1.07441652610453,-3.94117420681115,
-36.8551409687596));
#26605=CARTESIAN_POINT('Ctrl Pts',(-1.18932220553573,-3.90984938977799,
-36.8609589826525));
#26606=CARTESIAN_POINT('Ctrl Pts',(-1.30300733016968,-3.87345422796144,
-36.8667769965454));
#26607=CARTESIAN_POINT('Ctrl Pts',(-1.41499344566709,-3.83210367144721,
-36.8725950104383));
#26608=CARTESIAN_POINT('Ctrl Pts',(-1.52686812925343,-3.79079426085108,
-36.8784072351098));
#26609=CARTESIAN_POINT('Ctrl Pts',(-1.63704678640305,-3.74453940564873,
-36.8842194597814));
#26610=CARTESIAN_POINT('Ctrl Pts',(-1.74506504863759,-3.69350415947017,
-36.890031684453));
#26611=CARTESIAN_POINT('Ctrl Pts',(-1.85673506199582,-3.64074357524484,
-36.8960404018058));
#26612=CARTESIAN_POINT('Ctrl Pts',(-1.9660955919792,-3.58287377121514,-36.9020491191587));
#26613=CARTESIAN_POINT('Ctrl Pts',(-2.07265446226879,-3.52013188389828,
-36.9080578365116));
#26614=CARTESIAN_POINT('Ctrl Pts',(-2.17561393055959,-3.45950932530555,
-36.9138635882249));
#26615=CARTESIAN_POINT('Ctrl Pts',(-2.27595757457715,-3.39433873481196,
-36.9196693399383));
#26616=CARTESIAN_POINT('Ctrl Pts',(-2.37326606047514,-3.32488093113074,
-36.9254750916517));
#26617=CARTESIAN_POINT('Ctrl Pts',(-2.47056045552059,-3.25543318535619,
-36.9312800026574));
#26618=CARTESIAN_POINT('Ctrl Pts',(-2.56482023449916,-3.18169969803635,
-36.9370849136632));
#26619=CARTESIAN_POINT('Ctrl Pts',(-2.65565576540302,-3.1039841261968,-36.9428898246689));
#26620=CARTESIAN_POINT('Ctrl Pts',(-2.74649954090315,-3.02626150058096,
-36.9486952625515));
#26621=CARTESIAN_POINT('Ctrl Pts',(-2.83391814032715,-2.94455633711105,
-36.9545007004342));
#26622=CARTESIAN_POINT('Ctrl Pts',(-2.91755618456264,-2.85921158886856,
-36.9603061383169));
#26623=CARTESIAN_POINT('Ctrl Pts',(-3.00122152258653,-2.77383898988517,
-36.9661134707009));
#26624=CARTESIAN_POINT('Ctrl Pts',(-3.0811035663642,-2.68482473527792,-36.971920803085));
#26625=CARTESIAN_POINT('Ctrl Pts',(-3.15688530885822,-2.59254703847686,
-36.9777281354691));
#26626=CARTESIAN_POINT('Ctrl Pts',(-3.23275060673821,-2.50016759819091,
-36.9835418708981));
#26627=CARTESIAN_POINT('Ctrl Pts',(-3.3045063202977,-2.40451784903669,-36.989355606327));
#26628=CARTESIAN_POINT('Ctrl Pts',(-3.3718770139343,-2.30600745942018,-36.995169341756));
#26629=CARTESIAN_POINT('Ctrl Pts',(-3.43929204391157,-2.20743224057366,
-37.0009869031773));
#26630=CARTESIAN_POINT('Ctrl Pts',(-3.50231609198979,-2.10599297779654,
-37.0068044645985));
#26631=CARTESIAN_POINT('Ctrl Pts',(-3.56071902041228,-2.00212513536847,
-37.0126220260198));
#26632=CARTESIAN_POINT('Ctrl Pts',(-3.61920472967253,-1.89811006972326,
-37.0184478333051));
#26633=CARTESIAN_POINT('Ctrl Pts',(-3.67305606280072,-1.79165991683374,
-37.0242736405904));
#26634=CARTESIAN_POINT('Ctrl Pts',(-3.72209039230199,-1.68323144918732,
-37.0300994478757));
#26635=CARTESIAN_POINT('Ctrl Pts',(-3.73370957589475,-1.65753821987064,
-37.0314799322244));
#26636=CARTESIAN_POINT('Ctrl Pts',(-3.74505850319891,-1.63173397917305,
-37.032860416573));
#26637=CARTESIAN_POINT('Ctrl Pts',(-3.75613515493064,-1.60582492753544,
-37.0342409009217));
#26638=CARTESIAN_POINT('Ctrl Pts',(-3.80987693409516,-1.48011920299036,
-37.0409387448915));
#26639=CARTESIAN_POINT('Ctrl Pts',(-3.8573578000689,-1.35158683004276,-37.0476365888612));
#26640=CARTESIAN_POINT('Ctrl Pts',(-3.89830388899858,-1.22084060753995,
-37.054334432831));
#26641=CARTESIAN_POINT('Ctrl Pts',(-3.93744257703139,-1.09586565272087,
-37.0607366273379));
#26642=CARTESIAN_POINT('Ctrl Pts',(-3.97061085531542,-0.968868392783439,
-37.0671388218447));
#26643=CARTESIAN_POINT('Ctrl Pts',(-3.99761682229106,-0.8404074857684,-37.0735410163516));
#26644=CARTESIAN_POINT('Ctrl Pts',(-4.02455076465145,-0.712289182571588,
-37.0799261362766));
#26645=CARTESIAN_POINT('Ctrl Pts',(-4.04535509838463,-0.582715268947795,
-37.0863112562016));
#26646=CARTESIAN_POINT('Ctrl Pts',(-4.05988750416817,-0.452259276852506,
-37.0926963761265));
#26647=CARTESIAN_POINT('Ctrl Pts',(-4.07436256324668,-0.322318080545952,
-37.0990562995634));
#26648=CARTESIAN_POINT('Ctrl Pts',(-4.08261499785419,-0.191502005844116,
-37.1054162230003));
#26649=CARTESIAN_POINT('Ctrl Pts',(-4.08455354278761,-0.0603933448418993,
-37.1117761464372));
#26650=CARTESIAN_POINT('Ctrl Pts',(-4.08484197920292,-0.0408856658898553,
-37.1127224404777));
#26651=CARTESIAN_POINT('Ctrl Pts',(-4.08499072643696,-0.0213715335651584,
-37.1136687345182));
#26652=CARTESIAN_POINT('Ctrl Pts',(-4.08499957977947,-0.00185289005462216,
-37.1146150285587));
#26653=CARTESIAN_POINT('Ctrl Pts',(-4.08499957977981,-0.00185288929646346,
-37.1146150285955));
#26654=CARTESIAN_POINT('Ctrl Pts',(-4.08505473546161,0.119746894016321,
-37.1205103742538));
#26655=CARTESIAN_POINT('Ctrl Pts',(-4.07967598016496,0.241334433021924,
-37.1264057199121));
#26656=CARTESIAN_POINT('Ctrl Pts',(-4.06889302361888,0.362401106987252,
-37.1323010655705));
#26657=CARTESIAN_POINT('Ctrl Pts',(-4.0581063695184,0.483509295597695,-37.1381984327858));
#26658=CARTESIAN_POINT('Ctrl Pts',(-4.04191185845429,0.604095875033717,
-37.1440958000011));
#26659=CARTESIAN_POINT('Ctrl Pts',(-4.02039100139374,0.723658203789787,
-37.1499931672164));
#26660=CARTESIAN_POINT('Ctrl Pts',(-3.9988583612579,0.84328599517664,-37.1558937633516));
#26661=CARTESIAN_POINT('Ctrl Pts',(-3.97199363687583,0.961888035660562,
-37.1617943594867));
#26662=CARTESIAN_POINT('Ctrl Pts',(-3.93992918942795,1.07897311472235,-37.1676949556219));
#26663=CARTESIAN_POINT('Ctrl Pts',(-3.90781874707215,1.1962261466995,-37.1736040158784));
#26664=CARTESIAN_POINT('Ctrl Pts',(-3.87049378751551,1.31195749460793,-37.1795130761349));
#26665=CARTESIAN_POINT('Ctrl Pts',(-3.82813637309824,1.42569172999012,-37.1854221363915));
#26666=CARTESIAN_POINT('Ctrl Pts',(-3.78574545813174,1.5395159179675,-37.1913358701336));
#26667=CARTESIAN_POINT('Ctrl Pts',(-3.73831430745432,1.65133948690727,-37.1972496038757));
#26668=CARTESIAN_POINT('Ctrl Pts',(-3.68607220043215,1.76070915633483,-37.2031633376178));
#26669=CARTESIAN_POINT('Ctrl Pts',(-3.63373917189645,1.87026917137525,-37.2090873635485));
#26670=CARTESIAN_POINT('Ctrl Pts',(-3.57657864329999,1.97736641136903,-37.2150113894793));
#26671=CARTESIAN_POINT('Ctrl Pts',(-3.51486503032096,2.08157363997213,-37.2209354154101));
#26672=CARTESIAN_POINT('Ctrl Pts',(-3.48055184422449,2.13951356367859,-37.2242292138832));
#26673=CARTESIAN_POINT('Ctrl Pts',(-3.44483186559839,2.19656059362429,-37.2275230123564));
#26674=CARTESIAN_POINT('Ctrl Pts',(-3.40775771819042,2.25264562994574,-37.2308168108295));
#26675=CARTESIAN_POINT('Ctrl Pts',(-3.34218511804745,2.35184256144197,-37.2366425127089));
#26676=CARTESIAN_POINT('Ctrl Pts',(-3.27217279490521,2.44833254806676,-37.2424682145883));
#26677=CARTESIAN_POINT('Ctrl Pts',(-3.19797134279151,2.54169319365739,-37.2482939164677));
#26678=CARTESIAN_POINT('Ctrl Pts',(-3.12386299720566,2.63493669213967,-37.2541123083705));
#26679=CARTESIAN_POINT('Ctrl Pts',(-3.04557622945642,2.72505834313826,-37.2599307002734));
#26680=CARTESIAN_POINT('Ctrl Pts',(-2.96340543128871,2.81166378676551,-37.2657490921762));
#26681=CARTESIAN_POINT('Ctrl Pts',(-2.8813163697767,2.89818308252169,-37.2715616964281));
#26682=CARTESIAN_POINT('Ctrl Pts',(-2.79535124321465,2.98119283488133,-37.2773743006801));
#26683=CARTESIAN_POINT('Ctrl Pts',(-2.70584492772651,3.06033139171181,-37.283186904932));
#26684=CARTESIAN_POINT('Ctrl Pts',(-2.61332091521497,3.14213809755591,-37.2891954805905));
#26685=CARTESIAN_POINT('Ctrl Pts',(-2.51701298912991,3.21980761384266,-37.2952040562491));
#26686=CARTESIAN_POINT('Ctrl Pts',(-2.41733312448836,3.29298125795628,-37.3012126319077));
#26687=CARTESIAN_POINT('Ctrl Pts',(-2.32101170661539,3.3636895115971,-37.3070187646598));
#26688=CARTESIAN_POINT('Ctrl Pts',(-2.22154226226428,3.43019970545135,-37.312824897412));
#26689=CARTESIAN_POINT('Ctrl Pts',(-2.11932990166901,3.49222934067791,-37.3186310301642));
#26690=CARTESIAN_POINT('Ctrl Pts',(-2.01713234332954,3.5542499928566,-37.3244363220801));
#26691=CARTESIAN_POINT('Ctrl Pts',(-1.91219300741612,3.61179116524839,-37.330241613996));
#26692=CARTESIAN_POINT('Ctrl Pts',(-1.80494465494147,3.66461454898032,-37.3360469059119));
#26693=CARTESIAN_POINT('Ctrl Pts',(-1.69768657892346,3.71744272188103,-37.3418527241577));
#26694=CARTESIAN_POINT('Ctrl Pts',(-1.58811943612311,3.76555207541462,-37.3476585424034));
#26695=CARTESIAN_POINT('Ctrl Pts',(-1.47669858897939,3.80875127532716,-37.3534643606491));
#26696=CARTESIAN_POINT('Ctrl Pts',(-1.36524140254996,3.85196456441699,-37.35927207243));
#26697=CARTESIAN_POINT('Ctrl Pts',(-1.25192968958113,3.89026436757713,-37.3650797842109));
#26698=CARTESIAN_POINT('Ctrl Pts',(-1.13723608154764,3.92350851851072,-37.3708874959917));
#26699=CARTESIAN_POINT('Ctrl Pts',(-1.02241608874378,3.95678930229991,-37.3767016074869));
#26700=CARTESIAN_POINT('Ctrl Pts',(-0.906211553442713,3.98500320025736,
-37.382515718982));
#26701=CARTESIAN_POINT('Ctrl Pts',(-0.789107617796565,4.00805865320549,
-37.3883298304771));
#26702=CARTESIAN_POINT('Ctrl Pts',(-0.671926652090707,4.03112927185158,
-37.3941477664497));
#26703=CARTESIAN_POINT('Ctrl Pts',(-0.553845510216698,4.04903462673042,
-37.3999657024222));
#26704=CARTESIAN_POINT('Ctrl Pts',(-0.435355176305768,4.06173495817536,
-37.4057836383947));
#26705=CARTESIAN_POINT('Ctrl Pts',(-0.316697006269296,4.07445327905751,
-37.4116098152069));
#26706=CARTESIAN_POINT('Ctrl Pts',(-0.197628893062967,4.08195183605581,
-37.4174359920189));
#26707=CARTESIAN_POINT('Ctrl Pts',(-0.0786426664223028,4.08424293241942,
-37.4232621688311));
#26708=CARTESIAN_POINT('Ctrl Pts',(-0.0505236671123266,4.0847843676669,
-37.4246390194665));
#26709=CARTESIAN_POINT('Ctrl Pts',(-0.0224092201751181,4.08503520577175,
-37.4260158701019));
#26710=CARTESIAN_POINT('Ctrl Pts',(0.00569423172731292,4.08499603129857,
-37.4273927207374));
#26711=CARTESIAN_POINT('Ctrl Pts',(0.12455891370801,4.08483034128609,-37.433216165967));
#26712=CARTESIAN_POINT('Ctrl Pts',(0.24360683494036,4.07947201898683,-37.4390396111966));
#26713=CARTESIAN_POINT('Ctrl Pts',(0.362347851072246,4.06889776657307,-37.4448630564262));
#26714=CARTESIAN_POINT('Ctrl Pts',(0.480949503326026,4.05833592494097,-37.4506796667985));
#26715=CARTESIAN_POINT('Ctrl Pts',(0.59924456398741,4.0425703610407,-37.4564962771707));
#26716=CARTESIAN_POINT('Ctrl Pts',(0.716742062204008,4.02162974629286,-37.462312887543));
#26717=CARTESIAN_POINT('Ctrl Pts',(0.834129368664295,4.00070877011734,-37.4681240429691));
#26718=CARTESIAN_POINT('Ctrl Pts',(0.950720200828518,3.97462246633722,-37.4739351983953));
#26719=CARTESIAN_POINT('Ctrl Pts',(1.06602852163193,3.94345130451325,-37.4797463538215));
#26720=CARTESIAN_POINT('Ctrl Pts',(1.18125589513586,3.9123020250769,-37.4855534297733));
#26721=CARTESIAN_POINT('Ctrl Pts',(1.2952021557613,3.87607509511182,-37.4913605057252));
#26722=CARTESIAN_POINT('Ctrl Pts',(1.40739190563755,3.83490195754023,-37.497167581677));
#26723=CARTESIAN_POINT('Ctrl Pts',(1.51953878294409,3.79374455401042,-37.5029724384932));
#26724=CARTESIAN_POINT('Ctrl Pts',(1.6299301014438,3.74764484111999,-37.5087772953095));
#26725=CARTESIAN_POINT('Ctrl Pts',(1.73810656286463,3.69678381517325,-37.5145821521257));
#26726=CARTESIAN_POINT('Ctrl Pts',(1.84625869051855,3.64593423016601,-37.5203857031677));
#26727=CARTESIAN_POINT('Ctrl Pts',(1.95219658478059,3.59032563997139,-37.5261892542097));
#26728=CARTESIAN_POINT('Ctrl Pts',(2.05548253496176,3.53018647502751,-37.5319928052517));
#26729=CARTESIAN_POINT('Ctrl Pts',(2.15879230275974,3.47003344206399,-37.5377976945857));
#26730=CARTESIAN_POINT('Ctrl Pts',(2.25944855246946,3.40534795340386,-37.5436025839197));
#26731=CARTESIAN_POINT('Ctrl Pts',(2.3570399952545,3.33640337201164,-37.5494074732536));
#26732=CARTESIAN_POINT('Ctrl Pts',(2.40101277785794,3.30533830111272,-37.5520230420928));
#26733=CARTESIAN_POINT('Ctrl Pts',(2.44436372773356,3.27340912252422,-37.554638610932));
#26734=CARTESIAN_POINT('Ctrl Pts',(2.4870572760686,3.24064362520074,-37.5572541797712));
#26735=CARTESIAN_POINT('',(-4.08499880087778,0.00312998835824307,-37.0103849713737));
#26736=CARTESIAN_POINT('Ctrl Pts',(-4.08499880087729,0.00312998898833224,
-37.0103849714045));
#26737=CARTESIAN_POINT('Ctrl Pts',(-4.08485458355566,0.191350327181431,
-37.0195759887022));
#26738=CARTESIAN_POINT('Ctrl Pts',(-4.07169872079374,0.379076168690209,
-37.0287670059998));
#26739=CARTESIAN_POINT('Ctrl Pts',(-4.04575227482873,0.564901346004933,
-37.0379580232975));
#26740=CARTESIAN_POINT('Ctrl Pts',(-4.04148590491574,0.5954565498521,-37.039469300785));
#26741=CARTESIAN_POINT('Ctrl Pts',(-4.0368738005675,0.625960438495345,-37.0409805782726));
#26742=CARTESIAN_POINT('Ctrl Pts',(-4.03191704667525,0.656406831720633,
-37.0424918557601));
#26743=CARTESIAN_POINT('Ctrl Pts',(-4.01281033940161,0.773767978862407,
-37.048317349055));
#26744=CARTESIAN_POINT('Ctrl Pts',(-3.98854459284321,0.890481918751973,
-37.0541428423498));
#26745=CARTESIAN_POINT('Ctrl Pts',(-3.95917503351028,1.00606066120731,-37.0599683356447));
#26746=CARTESIAN_POINT('Ctrl Pts',(-3.92984233639821,1.12149433886671,-37.0657865172663));
#26747=CARTESIAN_POINT('Ctrl Pts',(-3.89541866753644,1.23579526104816,-37.071604698888));
#26748=CARTESIAN_POINT('Ctrl Pts',(-3.85601069792159,1.34848303567908,-37.0774228805096));
#26749=CARTESIAN_POINT('Ctrl Pts',(-3.81664193913112,1.4610586862756,-37.0832352730561));
#26750=CARTESIAN_POINT('Ctrl Pts',(-3.77229887976568,1.57202399953313,-37.0890476656026));
#26751=CARTESIAN_POINT('Ctrl Pts',(-3.72313853025277,1.68091180153725,-37.0948600581491));
#26752=CARTESIAN_POINT('Ctrl Pts',(-3.67231822656987,1.79347632192906,-37.100868712629));
#26753=CARTESIAN_POINT('Ctrl Pts',(-3.61634966291073,1.90382011894975,-37.106877367109));
#26754=CARTESIAN_POINT('Ctrl Pts',(-3.5554614139301,2.01144702491868,-37.1128860215889));
#26755=CARTESIAN_POINT('Ctrl Pts',(-3.496627570872,2.11544253473566,-37.1186919404745));
#26756=CARTESIAN_POINT('Ctrl Pts',(-3.43320089022276,2.21690115161157,-37.12449785936));
#26757=CARTESIAN_POINT('Ctrl Pts',(-3.36543490981202,2.31539907312293,-37.1303037782455));
#26758=CARTESIAN_POINT('Ctrl Pts',(-3.29767874845482,2.41388272262999,-37.1361088558737));
#26759=CARTESIAN_POINT('Ctrl Pts',(-3.22558476896845,2.50940619388783,-37.1419139335019));
#26760=CARTESIAN_POINT('Ctrl Pts',(-3.14944985494286,2.60157464071289,-37.1477190111301));
#26761=CARTESIAN_POINT('Ctrl Pts',(-3.07330804038194,2.69375144128252,-37.1535246149052));
#26762=CARTESIAN_POINT('Ctrl Pts',(-2.99312482293973,2.78257229824525,-37.1593302186802));
#26763=CARTESIAN_POINT('Ctrl Pts',(-2.90923696921039,2.86767593304745,-37.1651358224552));
#26764=CARTESIAN_POINT('Ctrl Pts',(-2.82532175412129,2.95280732575577,-37.1709433198204));
#26765=CARTESIAN_POINT('Ctrl Pts',(-2.73769978589935,3.03421879460071,-37.1767508171856));
#26766=CARTESIAN_POINT('Ctrl Pts',(-2.64674375059762,3.11158681683035,-37.1825583145507));
#26767=CARTESIAN_POINT('Ctrl Pts',(-2.55568746584244,3.18904011214734,-37.1883722127934));
#26768=CARTESIAN_POINT('Ctrl Pts',(-2.46129009004387,3.26244080079951,-37.194186111036));
#26769=CARTESIAN_POINT('Ctrl Pts',(-2.36395647938206,3.33150638054133,-37.2000000092786));
#26770=CARTESIAN_POINT('Ctrl Pts',(-2.2665588337801,3.40061739793037,-37.2058177324346));
#26771=CARTESIAN_POINT('Ctrl Pts',(-2.16622144816884,3.46538740566566,-37.2116354555906));
#26772=CARTESIAN_POINT('Ctrl Pts',(-2.06337575569537,3.52557874551237,-37.2174531787466));
#26773=CARTESIAN_POINT('Ctrl Pts',(-1.96038434205945,3.58585536994223,-37.2232791449836));
#26774=CARTESIAN_POINT('Ctrl Pts',(-1.85487788776261,3.64154018859385,-37.2291051112207));
#26775=CARTESIAN_POINT('Ctrl Pts',(-1.74730995426144,3.69244267710941,-37.2349310774577));
#26776=CARTESIAN_POINT('Ctrl Pts',(-1.72185065794288,3.70449033384398,-37.2363099735278));
#26777=CARTESIAN_POINT('Ctrl Pts',(-1.69627595666987,3.71627031161957,-37.2376888695979));
#26778=CARTESIAN_POINT('Ctrl Pts',(-1.67059199348252,3.72778049129936,-37.239067765668));
#26779=CARTESIAN_POINT('Ctrl Pts',(-1.56208673973579,3.77640674721308,-37.2448930920354));
#26780=CARTESIAN_POINT('Ctrl Pts',(-1.45128304613134,3.82036945305346,-37.2507184184027));
#26781=CARTESIAN_POINT('Ctrl Pts',(-1.33861873677264,3.85944618793438,-37.2565437447701));
#26782=CARTESIAN_POINT('Ctrl Pts',(-1.22609584505556,3.89847387321193,-37.2623617591154));
#26783=CARTESIAN_POINT('Ctrl Pts',(-1.11171736502236,3.9326276534788,-37.2681797734607));
#26784=CARTESIAN_POINT('Ctrl Pts',(-0.995943087002967,3.96173224328084,
-37.273997787806));
#26785=CARTESIAN_POINT('Ctrl Pts',(-0.880284010305376,3.990807872529,-37.2798100129298));
#26786=CARTESIAN_POINT('Ctrl Pts',(-0.763232292185154,4.01484420762205,
-37.2856222380536));
#26787=CARTESIAN_POINT('Ctrl Pts',(-0.645264388233329,4.03371526874145,
-37.2914344631774));
#26788=CARTESIAN_POINT('Ctrl Pts',(-0.523308380602152,4.05322429786537,
-37.2974431803606));
#26789=CARTESIAN_POINT('Ctrl Pts',(-0.400373562924836,4.06721247861894,
-37.3034518975439));
#26790=CARTESIAN_POINT('Ctrl Pts',(-0.277000042696729,4.07559762198699,
-37.3094606147272));
#26791=CARTESIAN_POINT('Ctrl Pts',(-0.157793886046388,4.08369952839299,
-37.3152663668893));
#26792=CARTESIAN_POINT('Ctrl Pts',(-0.0381786251328157,4.08657077786004,
-37.3210721190515));
#26793=CARTESIAN_POINT('Ctrl Pts',(0.0813523796059202,4.08418985728289,
-37.3268778712136));
#26794=CARTESIAN_POINT('Ctrl Pts',(0.200866075497529,4.08180928147814,-37.3326827826661));
#26795=CARTESIAN_POINT('Ctrl Pts',(0.320295131630733,4.07417805629591,-37.3384876941185));
#26796=CARTESIAN_POINT('Ctrl Pts',(0.439146512970421,4.06132679553689,-37.3442926055709));
#26797=CARTESIAN_POINT('Ctrl Pts',(0.558008681684835,4.04847436835166,-37.3500980438978));
#26798=CARTESIAN_POINT('Ctrl Pts',(0.676292665669839,4.03040100744962,-37.3559034822247));
#26799=CARTESIAN_POINT('Ctrl Pts',(0.79351151155194,4.00718909973495,-37.3617089205516));
#26800=CARTESIAN_POINT('Ctrl Pts',(0.910768609656701,3.98396961723948,-37.3675162533769));
#26801=CARTESIAN_POINT('Ctrl Pts',(1.02695947832406,3.95560833219552,-37.3733235862022));
#26802=CARTESIAN_POINT('Ctrl Pts',(1.14160892428342,3.92223839968919,-37.3791309190275));
#26803=CARTESIAN_POINT('Ctrl Pts',(1.25638478021734,3.88883167422426,-37.3849446548911));
#26804=CARTESIAN_POINT('Ctrl Pts',(1.36961542909423,3.85040539238144,-37.3907583907547));
#26805=CARTESIAN_POINT('Ctrl Pts',(1.48084222697353,3.80714214323711,-37.3965721266184));
#26806=CARTESIAN_POINT('Ctrl Pts',(1.59214222262247,3.76385042277648,-37.4023896884709));
#26807=CARTESIAN_POINT('Ctrl Pts',(1.70143536841723,3.7157155596164,-37.4082072503235));
#26808=CARTESIAN_POINT('Ctrl Pts',(1.80828584066702,3.66296701028595,-37.414024812176));
#26809=CARTESIAN_POINT('Ctrl Pts',(1.91528776358037,3.61014369476467,-37.4198506198845));
#26810=CARTESIAN_POINT('Ctrl Pts',(2.01983974643858,3.55269383693167,-37.4256764275931));
#26811=CARTESIAN_POINT('Ctrl Pts',(2.12153314572536,3.49089130618366,-37.4315022353016));
#26812=CARTESIAN_POINT('Ctrl Pts',(2.14563035596093,3.4762466135392,-37.432882715393));
#26813=CARTESIAN_POINT('Ctrl Pts',(2.16956719796205,3.46135770180052,-37.4342631954844));
#26814=CARTESIAN_POINT('Ctrl Pts',(2.19333850413813,3.44622854817627,-37.4356436755758));
#26815=CARTESIAN_POINT('Ctrl Pts',(2.29403836309909,3.38213852195406,-37.441491656729));
#26816=CARTESIAN_POINT('Ctrl Pts',(2.392088474289,3.31352817431584,-37.4473396378822));
#26817=CARTESIAN_POINT('Ctrl Pts',(2.48705727606859,3.24064362520075,-37.4531876190354));
#26818=CARTESIAN_POINT('Ctrl Pts',(2.4870572760686,3.24064362520075,-36.2030038303486));
#26819=CARTESIAN_POINT('Ctrl Pts',(2.58187463704937,3.16787530051023,-36.2088183190398));
#26820=CARTESIAN_POINT('Ctrl Pts',(2.67342647523315,3.09099531024705,-36.2146328077311));
#26821=CARTESIAN_POINT('Ctrl Pts',(2.76135293747853,3.01034133524401,-36.2204472964224));
#26822=CARTESIAN_POINT('Ctrl Pts',(2.85143172726396,2.92771305390383,-36.2264041163735));
#26823=CARTESIAN_POINT('Ctrl Pts',(2.93770502899664,2.84112395663559,-36.2323609363245));
#26824=CARTESIAN_POINT('Ctrl Pts',(3.01982847136758,2.75097455522906,-36.2383177562756));
#26825=CARTESIAN_POINT('Ctrl Pts',(3.10195191373852,2.66082515382254,-36.2442745762267));
#26826=CARTESIAN_POINT('Ctrl Pts',(3.17992525499167,2.56711583740487,-36.2502313961777));
#26827=CARTESIAN_POINT('Ctrl Pts',(3.25345117218819,2.47027943160026,-36.2561882161288));
#26828=CARTESIAN_POINT('Ctrl Pts',(3.32535558943459,2.37557860238101,-36.2620136676642));
#26829=CARTESIAN_POINT('Ctrl Pts',(3.39323680231942,2.27758420590494,-36.2678391191996));
#26830=CARTESIAN_POINT('Ctrl Pts',(3.45677914334209,2.17667244990034,-36.273664570735));
#26831=CARTESIAN_POINT('Ctrl Pts',(3.52024172793067,2.07588735529484,-36.2794827103389));
#26832=CARTESIAN_POINT('Ctrl Pts',(3.57937605736851,1.97219252677822,-36.2853008499429));
#26833=CARTESIAN_POINT('Ctrl Pts',(3.63390741223458,1.86599622703439,-36.2911189895468));
#26834=CARTESIAN_POINT('Ctrl Pts',(3.68838450623552,1.75990559682896,-36.2969313398707));
#26835=CARTESIAN_POINT('Ctrl Pts',(3.73826755215734,1.65131880808949,-36.3027436901945));
#26836=CARTESIAN_POINT('Ctrl Pts',(3.78332609109917,1.54067150567805,-36.3085560405183));
#26837=CARTESIAN_POINT('Ctrl Pts',(3.82990654245871,1.42628694263898,-36.3145647107483));
#26838=CARTESIAN_POINT('Ctrl Pts',(3.8713305729448,1.30970058469697,-36.3205733809782));
#26839=CARTESIAN_POINT('Ctrl Pts',(3.90739600376305,1.19141993846693,-36.3265820512081));
#26840=CARTESIAN_POINT('Ctrl Pts',(3.94224421918767,1.07713128734392,-36.3323879276343));
#26841=CARTESIAN_POINT('Ctrl Pts',(3.97208957743956,0.961261289019829,-36.3381938040605));
#26842=CARTESIAN_POINT('Ctrl Pts',(3.99679955667867,0.844285676612574,-36.3439996804867));
#26843=CARTESIAN_POINT('Ctrl Pts',(4.02150595544695,0.727327013947177,-36.3498047156426));
#26844=CARTESIAN_POINT('Ctrl Pts',(4.04107837076155,0.609263454906169,-36.3556097507985));
#26845=CARTESIAN_POINT('Ctrl Pts',(4.05543513104386,0.490582202994803,-36.3614147859544));
#26846=CARTESIAN_POINT('Ctrl Pts',(4.06979319265331,0.371890193563596,-36.367220347291));
#26847=CARTESIAN_POINT('Ctrl Pts',(4.07893461027165,0.252580785023341,-36.3730259086276));
#26848=CARTESIAN_POINT('Ctrl Pts',(4.08282951957093,0.133146964367187,-36.3788314699642));
#26849=CARTESIAN_POINT('Ctrl Pts',(4.08672569932034,0.0136741865233215,
-36.3846389249716));
#26850=CARTESIAN_POINT('Ctrl Pts',(4.08537195399314,-0.105922676559767,
-36.390446379979));
#26851=CARTESIAN_POINT('Ctrl Pts',(4.07879053171232,-0.225150612732684,
-36.3962538349864));
#26852=CARTESIAN_POINT('Ctrl Pts',(4.07220185512428,-0.344509966711937,
-36.4020676912033));
#26853=CARTESIAN_POINT('Ctrl Pts',(4.06037402255944,-0.463499174477577,
-36.4078815474203));
#26854=CARTESIAN_POINT('Ctrl Pts',(4.04338117799063,-0.581630165544313,
-36.4136954036372));
#26855=CARTESIAN_POINT('Ctrl Pts',(4.02637715346937,-0.699838877492785,
-36.4195130849133));
#26856=CARTESIAN_POINT('Ctrl Pts',(4.00420142488322,-0.817187848249899,
-36.4253307661893));
#26857=CARTESIAN_POINT('Ctrl Pts',(3.97697895021239,-0.933200637359189,
-36.4311484474654));
#26858=CARTESIAN_POINT('Ctrl Pts',(3.94971790150782,-1.04937781568341,-36.4369743723504));
#26859=CARTESIAN_POINT('Ctrl Pts',(3.91739594400822,-1.16421464215036,-36.4428002972354));
#26860=CARTESIAN_POINT('Ctrl Pts',(3.8801874447013,-1.27725110842873,-36.4486262221203));
#26861=CARTESIAN_POINT('Ctrl Pts',(3.87137824570172,-1.30401275547719,-36.4500055234258));
#26862=CARTESIAN_POINT('Ctrl Pts',(3.86229535711031,-1.33067358484663,-36.4513848247312));
#26863=CARTESIAN_POINT('Ctrl Pts',(3.85294147739799,-1.35722767866935,-36.4527641260367));
#26864=CARTESIAN_POINT('Ctrl Pts',(3.81343551102534,-1.46937848345629,-36.458589583779));
#26865=CARTESIAN_POINT('Ctrl Pts',(3.76896558452616,-1.57998236229261,-36.4644150415214));
#26866=CARTESIAN_POINT('Ctrl Pts',(3.71967212011802,-1.6885687190093,-36.4702404992638));
#26867=CARTESIAN_POINT('Ctrl Pts',(3.67044052693488,-1.79701878238592,-36.4760586451198));
#26868=CARTESIAN_POINT('Ctrl Pts',(3.61639760517508,-1.9034559921634,-36.4818767909759));
#26869=CARTESIAN_POINT('Ctrl Pts',(3.55773307516494,-2.00742630397168,-36.487694936832));
#26870=CARTESIAN_POINT('Ctrl Pts',(3.49912691825589,-2.11129316196348,-36.4935072934451));
#26871=CARTESIAN_POINT('Ctrl Pts',(3.43590850110133,-2.21269765195627,-36.4993196500582));
#26872=CARTESIAN_POINT('Ctrl Pts',(3.36831476321685,-2.31120761851795,-36.5051320066713));
#26873=CARTESIAN_POINT('Ctrl Pts',(3.29843805929445,-2.41304474104254,-36.5111406745577));
#26874=CARTESIAN_POINT('Ctrl Pts',(3.22388543561436,-2.51178795092408,-36.5171493424441));
#26875=CARTESIAN_POINT('Ctrl Pts',(3.14496939547503,-2.60698916405984,-36.5231580103305));
#26876=CARTESIAN_POINT('Ctrl Pts',(3.06871667421491,-2.69897745384287,-36.5289638930975));
#26877=CARTESIAN_POINT('Ctrl Pts',(2.98839058523314,-2.78765862612755,-36.5347697758645));
#26878=CARTESIAN_POINT('Ctrl Pts',(2.90431543353171,-2.87266024140508,-36.5405756586315));
#26879=CARTESIAN_POINT('Ctrl Pts',(2.82025246417479,-2.95764954009513,-36.5463807001361));
#26880=CARTESIAN_POINT('Ctrl Pts',(2.7324417993068,-3.03896005209655,-36.5521857416407));
#26881=CARTESIAN_POINT('Ctrl Pts',(2.64124530328099,-3.11625548501661,-36.5579907831453));
#26882=CARTESIAN_POINT('Ctrl Pts',(2.55004054100715,-3.19355792416221,-36.5637963508314));
#26883=CARTESIAN_POINT('Ctrl Pts',(2.45544964865562,-3.26684429681266,-36.5696019185176));
#26884=CARTESIAN_POINT('Ctrl Pts',(2.35786782809665,-3.33581838612758,-36.5754074862037));
#26885=CARTESIAN_POINT('Ctrl Pts',(2.26025417822233,-3.40481497346545,-36.5812149475545));
#26886=CARTESIAN_POINT('Ctrl Pts',(2.15964799291212,-3.46949624467323,-36.5870224089053));
#26887=CARTESIAN_POINT('Ctrl Pts',(2.05647317141115,-3.5296094819776,-36.5928298702561));
#26888=CARTESIAN_POINT('Ctrl Pts',(1.9531846273436,-3.58978897800219,-36.5986437327753));
#26889=CARTESIAN_POINT('Ctrl Pts',(1.84732214855163,-3.64539018445363,-36.6044575952946));
#26890=CARTESIAN_POINT('Ctrl Pts',(1.73933406526962,-3.69620643489953,-36.6102714578138));
#26891=CARTESIAN_POINT('Ctrl Pts',(1.63127493472827,-3.74705611825037,-36.6160891453754));
#26892=CARTESIAN_POINT('Ctrl Pts',(1.52108779013081,-3.79311441897661,-36.6219068329371));
#26893=CARTESIAN_POINT('Ctrl Pts',(1.40923921274804,-3.83422349912643,-36.6277245204987));
#26894=CARTESIAN_POINT('Ctrl Pts',(1.29723214835793,-3.87539082995086,-36.6335504515974));
#26895=CARTESIAN_POINT('Ctrl Pts',(1.1835593398292,-3.91159481993312,-36.639376382696));
#26896=CARTESIAN_POINT('Ctrl Pts',(1.06870083667109,-3.94272792894698,-36.6452023137947));
#26897=CARTESIAN_POINT('Ctrl Pts',(1.04150904165693,-3.95009843348239,-36.6465815545113));
#26898=CARTESIAN_POINT('Ctrl Pts',(1.01425082784076,-3.95718495949799,-36.6479607952279));
#26899=CARTESIAN_POINT('Ctrl Pts',(0.986932620584834,-3.96398650381476,
-36.6493400359445));
#26900=CARTESIAN_POINT('Ctrl Pts',(0.871549970582555,-3.99271387234318,
-36.6551654712441));
#26901=CARTESIAN_POINT('Ctrl Pts',(0.75472741436091,-4.01644522789889,-36.6609909065437));
#26902=CARTESIAN_POINT('Ctrl Pts',(0.636935158523994,-4.03503886026343,
-36.6668163418433));
#26903=CARTESIAN_POINT('Ctrl Pts',(0.519290752117458,-4.05360915443877,
-36.6726344652252));
#26904=CARTESIAN_POINT('Ctrl Pts',(0.400679466532992,-4.06705448897578,
-36.678452588607));
#26905=CARTESIAN_POINT('Ctrl Pts',(0.281584815870499,-4.07528342467995,
-36.6842707119888));
#26906=CARTESIAN_POINT('Ctrl Pts',(0.162608668781168,-4.08350417228937,
-36.6900830461231));
#26907=CARTESIAN_POINT('Ctrl Pts',(0.0431505182011207,-4.08651881918968,
-36.6958953802575));
#26908=CARTESIAN_POINT('Ctrl Pts',(-0.076298414708443,-4.0842873983001,
-36.7017077143918));
#26909=CARTESIAN_POINT('Ctrl Pts',(-0.199782364003948,-4.08198059942568,
-36.7077163907026));
#26910=CARTESIAN_POINT('Ctrl Pts',(-0.323256023145913,-4.07406696201024,
-36.7137250670135));
#26911=CARTESIAN_POINT('Ctrl Pts',(-0.446173281238826,-4.06056084834455,
-36.7197337433243));
#26912=CARTESIAN_POINT('Ctrl Pts',(-0.564941610016865,-4.04751061786228,
-36.7255396037436));
#26913=CARTESIAN_POINT('Ctrl Pts',(-0.683190055011587,-4.02923940164376,
-36.7313454641629));
#26914=CARTESIAN_POINT('Ctrl Pts',(-0.800429181120055,-4.00581304181954,
-36.7371513245822));
#26915=CARTESIAN_POINT('Ctrl Pts',(-0.917651321175641,-3.9823900760959,
-36.7429563438262));
#26916=CARTESIAN_POINT('Ctrl Pts',(-1.03386403316443,-3.95381353209138,
-36.7487613630702));
#26917=CARTESIAN_POINT('Ctrl Pts',(-1.14858739600384,-3.92020050427795,
-36.7545663823143));
#26918=CARTESIAN_POINT('Ctrl Pts',(-1.26332115985405,-3.88658442905154,
-36.760371927851));
#26919=CARTESIAN_POINT('Ctrl Pts',(-1.37656491451374,-3.84793107688222,
-36.7661774733877));
#26920=CARTESIAN_POINT('Ctrl Pts',(-1.48785385632197,-3.80440743115506,
-36.7719830189244));
#26921=CARTESIAN_POINT('Ctrl Pts',(-1.59917910117831,-3.76086958778185,
-36.7777904582612));
#26922=CARTESIAN_POINT('Ctrl Pts',(-1.70854788519361,-3.71245843974745,
-36.7835978975979));
#26923=CARTESIAN_POINT('Ctrl Pts',(-1.81551593411231,-3.65938886878455,
-36.7894053369346));
#26924=CARTESIAN_POINT('Ctrl Pts',(-1.92260189275794,-3.60626079980581,
-36.7952191777491));
#26925=CARTESIAN_POINT('Ctrl Pts',(-2.02728146845473,-3.548464239783,-36.8010330185636));
#26926=CARTESIAN_POINT('Ctrl Pts',(-2.12913539516145,-3.4862598108963,-36.8068468593781));
#26927=CARTESIAN_POINT('Ctrl Pts',(-2.23105633633623,-3.42401445480288,
-36.8126645253907));
#26928=CARTESIAN_POINT('Ctrl Pts',(-2.33014758821295,-3.35735568125718,
-36.8184821914033));
#26929=CARTESIAN_POINT('Ctrl Pts',(-2.42602061258807,-3.28658622088297,
-36.8242998574159));
#26930=CARTESIAN_POINT('Ctrl Pts',(-2.52202949385745,-3.21571647662643,
-36.8301257673537));
#26931=CARTESIAN_POINT('Ctrl Pts',(-2.61481072952792,-3.14072467505461,
-36.8359516772915));
#26932=CARTESIAN_POINT('Ctrl Pts',(-2.70401036796732,-3.06195247022635,
-36.8417775872292));
#26933=CARTESIAN_POINT('Ctrl Pts',(-2.72513096525623,-3.04330086978441,
-36.8431570401036));
#26934=CARTESIAN_POINT('Ctrl Pts',(-2.74605093321617,-3.02443747840542,
-36.8445364929779));
#26935=CARTESIAN_POINT('Ctrl Pts',(-2.76676589646178,-3.00536711138191,
-36.8459159458523));
#26936=CARTESIAN_POINT('Ctrl Pts',(-2.85296777305954,-2.92600894862088,
-36.8516563097158));
#26937=CARTESIAN_POINT('Ctrl Pts',(-2.9359102855324,-2.84279355617639,-36.8573966735792));
#26938=CARTESIAN_POINT('Ctrl Pts',(-3.0152216656466,-2.75602309624128,-36.8631370374427));
#26939=CARTESIAN_POINT('Ctrl Pts',(-3.0944324328739,-2.66936271163783,-36.8688701191912));
#26940=CARTESIAN_POINT('Ctrl Pts',(-3.17002094314047,-2.57915653263523,
-36.8746032009398));
#26941=CARTESIAN_POINT('Ctrl Pts',(-3.24164959019338,-2.48574595129894,
-36.8803362826884));
#26942=CARTESIAN_POINT('Ctrl Pts',(-3.31319919234215,-2.39243845204993,
-36.8860630377658));
#26943=CARTESIAN_POINT('Ctrl Pts',(-3.38079737053372,-2.29593391815368,
-36.8917897928432));
#26944=CARTESIAN_POINT('Ctrl Pts',(-3.44414503611396,-2.19660874308821,
-36.8975165479206));
#26945=CARTESIAN_POINT('Ctrl Pts',(-3.50745410289587,-2.09734408852285,
-36.9032398135898));
#26946=CARTESIAN_POINT('Ctrl Pts',(-3.56651757797437,-1.9952625620178,-36.908963079259));
#26947=CARTESIAN_POINT('Ctrl Pts',(-3.62107844800158,-1.89077123772773,
-36.9146863449282));
#26948=CARTESIAN_POINT('Ctrl Pts',(-3.67561984362926,-1.78631720950343,
-36.9204075677934));
#26949=CARTESIAN_POINT('Ctrl Pts',(-3.72566163443285,-1.67945546632966,
-36.9261287906586));
#26950=CARTESIAN_POINT('Ctrl Pts',(-3.77099212964895,-1.57061878192185,
-36.9318500135238));
#26951=CARTESIAN_POINT('Ctrl Pts',(-3.81631788456961,-1.46179347877154,
-36.93757063811));
#26952=CARTESIAN_POINT('Ctrl Pts',(-3.85693316314368,-1.35099403439447,
-36.9432912626961));
#26953=CARTESIAN_POINT('Ctrl Pts',(-3.89267423871781,-1.23867359349537,
-36.9490118872823));
#26954=CARTESIAN_POINT('Ctrl Pts',(-3.92843606666944,-1.12628793586306,
-36.9547358334405));
#26955=CARTESIAN_POINT('Ctrl Pts',(-3.95931790999905,-1.01237991932313,
-36.9604597795988));
#26956=CARTESIAN_POINT('Ctrl Pts',(-3.98520586797416,-0.897418068608123,
-36.9661837257571));
#26957=CARTESIAN_POINT('Ctrl Pts',(-4.01110192825184,-0.782420237623872,
-36.9719094633716));
#26958=CARTESIAN_POINT('Ctrl Pts',(-4.03200091337673,-0.666368329771364,
-36.9776352009861));
#26959=CARTESIAN_POINT('Ctrl Pts',(-4.04784031633376,-0.549739732476181,
-36.9833609386006));
#26960=CARTESIAN_POINT('Ctrl Pts',(-4.06369764127743,-0.43297917211602,
-36.9890931547796));
#26961=CARTESIAN_POINT('Ctrl Pts',(-4.07448391270157,-0.315641038569806,
-36.9948253709586));
#26962=CARTESIAN_POINT('Ctrl Pts',(-4.080188622196,-0.1982064764388,-37.0005575871376));
#26963=CARTESIAN_POINT('Ctrl Pts',(-4.08344869767159,-0.131096041391466,
-37.003833381883));
#26964=CARTESIAN_POINT('Ctrl Pts',(-4.08505020174386,-0.0639541194029987,
-37.0071091766283));
#26965=CARTESIAN_POINT('Ctrl Pts',(-4.08499880087778,0.00312998835824298,
-37.0103849713737));
#26966=CARTESIAN_POINT('Origin',(0.,0.,-25.2396150285955));
#26967=CARTESIAN_POINT('',(2.48705727606859,3.24064362520075,-34.9531798329663));
#26968=CARTESIAN_POINT('',(2.4870572760686,3.24064362520075,-35.057284109232));
#26969=CARTESIAN_POINT('',(2.4870572760686,3.24064362520075,-25.2396150285955));
#26970=CARTESIAN_POINT('',(-4.08499983154849,-0.00117313631325986,-35.8646150286259));
#26971=CARTESIAN_POINT('Ctrl Pts',(2.4870572760686,3.24064362520074,-35.057284109232));
#26972=CARTESIAN_POINT('Ctrl Pts',(2.54761296302863,3.19416968999538,-35.0610166734358));
#26973=CARTESIAN_POINT('Ctrl Pts',(2.60681072845989,3.14603993011952,-35.0647492376396));
#26974=CARTESIAN_POINT('Ctrl Pts',(2.66455867416279,3.09634495364193,-35.0684818018434));
#26975=CARTESIAN_POINT('Ctrl Pts',(2.75468648016539,3.0187854985867,-35.0743072527466));
#26976=CARTESIAN_POINT('Ctrl Pts',(2.84156927643091,2.93716357340725,-35.0801327036498));
#26977=CARTESIAN_POINT('Ctrl Pts',(2.92481966594463,2.85178100872132,-35.085958154553));
#26978=CARTESIAN_POINT('Ctrl Pts',(3.00796556229563,2.76650561343455,-35.091776293541));
#26979=CARTESIAN_POINT('Ctrl Pts',(3.08748783801294,2.67747925686239,-35.097594432529));
#26980=CARTESIAN_POINT('Ctrl Pts',(3.16303243065348,2.58504368292575,-35.1034125715171));
#26981=CARTESIAN_POINT('Ctrl Pts',(3.23850185363169,2.49270008580223,-35.1092249212417));
#26982=CARTESIAN_POINT('Ctrl Pts',(3.31000121079498,2.39695433415158,-35.1150372709663));
#26983=CARTESIAN_POINT('Ctrl Pts',(3.37721399111375,2.29818420894096,-35.1208496206909));
#26984=CARTESIAN_POINT('Ctrl Pts',(3.44669698281696,2.19607797619791,-35.1268582911518));
#26985=CARTESIAN_POINT('Ctrl Pts',(3.51159839093206,2.09073976606651,-35.1328669616126));
#26986=CARTESIAN_POINT('Ctrl Pts',(3.5716143222271,1.98262354804493,-35.1388756320735));
#26987=CARTESIAN_POINT('Ctrl Pts',(3.62960469625512,1.87815628766459,-35.1446815079454));
#26988=CARTESIAN_POINT('Ctrl Pts',(3.68303383120364,1.77109589607329,-35.1504873838173));
#26989=CARTESIAN_POINT('Ctrl Pts',(3.73167259726826,1.66187984728053,-35.1562932596892));
#26990=CARTESIAN_POINT('Ctrl Pts',(3.78030431573155,1.55267962354324,-35.1620982943083));
#26991=CARTESIAN_POINT('Ctrl Pts',(3.82414687977847,1.44132473641654,-35.1679033289274));
#26992=CARTESIAN_POINT('Ctrl Pts',(3.86301848424554,1.32827451619658,-35.1737083635465));
#26993=CARTESIAN_POINT('Ctrl Pts',(3.90189361223779,1.21521404851444,-35.1795139243642));
#26994=CARTESIAN_POINT('Ctrl Pts',(3.93579675208558,1.10045832805974,-35.185319485182));
#26995=CARTESIAN_POINT('Ctrl Pts',(3.9645955489872,0.984483180633828,-35.1911250459997));
#26996=CARTESIAN_POINT('Ctrl Pts',(3.99340373963669,0.868470203804875,-35.1969325005068));
#26997=CARTESIAN_POINT('Ctrl Pts',(4.01710417778607,0.751237404722748,-35.2027399550139));
#26998=CARTESIAN_POINT('Ctrl Pts',(4.03561546230076,0.633271537682692,-35.2085474095209));
#26999=CARTESIAN_POINT('Ctrl Pts',(4.05414715079073,0.515175643326956,-35.2143612652671));
#27000=CARTESIAN_POINT('Ctrl Pts',(4.06747820553746,0.396345471471962,-35.2201751210133));
#27001=CARTESIAN_POINT('Ctrl Pts',(4.07557900651325,0.277273802708554,-35.2259889767595));
#27002=CARTESIAN_POINT('Ctrl Pts',(4.08368513720139,0.158123793822433,-35.2318066575816));
#27003=CARTESIAN_POINT('Ctrl Pts',(4.08655415117709,0.0387323785405584,
-35.2376243384036));
#27004=CARTESIAN_POINT('Ctrl Pts',(4.08420855108277,-0.0804084029337425,
-35.2434420192257));
#27005=CARTESIAN_POINT('Ctrl Pts',(4.08185962728007,-0.199718006542317,
-35.2492679436843));
#27006=CARTESIAN_POINT('Ctrl Pts',(4.07428136757816,-0.318775861817394,
-35.2550938681429));
#27007=CARTESIAN_POINT('Ctrl Pts',(4.0615480281694,-0.437095658721621,-35.2609197926015));
#27008=CARTESIAN_POINT('Ctrl Pts',(4.05853336904505,-0.465108251795378,
-35.2622990989847));
#27009=CARTESIAN_POINT('Ctrl Pts',(4.055229981517,-0.493079524776221,-35.263678405368));
#27010=CARTESIAN_POINT('Ctrl Pts',(4.05163926609921,-0.521003126097207,
-35.2650577117513));
#27011=CARTESIAN_POINT('Ctrl Pts',(4.03647400820025,-0.638937455674511,
-35.2708831628355));
#27012=CARTESIAN_POINT('Ctrl Pts',(4.01613100473269,-0.756397754621066,
-35.2767086139198));
#27013=CARTESIAN_POINT('Ctrl Pts',(3.99064910219284,-0.872894462788894,
-35.2825340650041));
#27014=CARTESIAN_POINT('Ctrl Pts',(3.96519918371308,-0.989244948055602,
-35.2883522041705));
#27015=CARTESIAN_POINT('Ctrl Pts',(3.93462328211081,-1.10463385306709,-35.2941703433369));
#27016=CARTESIAN_POINT('Ctrl Pts',(3.8990119140391,-1.2185774879675,-35.2999884825034));
#27017=CARTESIAN_POINT('Ctrl Pts',(3.86343598061113,-1.33240774468762,-35.3058008324036));
#27018=CARTESIAN_POINT('Ctrl Pts',(3.82283466967113,-1.44479520503797,-35.3116131823039));
#27019=CARTESIAN_POINT('Ctrl Pts',(3.77734925186654,-1.55526770345922,-35.3174255322041));
#27020=CARTESIAN_POINT('Ctrl Pts',(3.7303274985294,-1.66947156970967,-35.3234342025981));
#27021=CARTESIAN_POINT('Ctrl Pts',(3.67808595754768,-1.7816283891354,-35.329442872992));
#27022=CARTESIAN_POINT('Ctrl Pts',(3.62083645882539,-1.89123460692766,-35.335451543386));
#27023=CARTESIAN_POINT('Ctrl Pts',(3.56551914715493,-1.9971415833371,-35.3412574194255));
#27024=CARTESIAN_POINT('Ctrl Pts',(3.50552666701297,-2.10066695656878,-35.3470632954651));
#27025=CARTESIAN_POINT('Ctrl Pts',(3.44109821563374,-2.20137867491313,-35.3528691715046));
#27026=CARTESIAN_POINT('Ctrl Pts',(3.37667909976621,-2.30207580039664,-35.3586742062881));
#27027=CARTESIAN_POINT('Ctrl Pts',(3.3078255107762,-2.39995973817966,-35.3644792410716));
#27028=CARTESIAN_POINT('Ctrl Pts',(3.23482093722727,-2.4946259246781,-35.3702842758551));
#27029=CARTESIAN_POINT('Ctrl Pts',(3.16180974620552,-2.58930069215833,-35.3760898368339));
#27030=CARTESIAN_POINT('Ctrl Pts',(3.08464707169867,-2.68075680532705,-35.3818953978126));
#27031=CARTESIAN_POINT('Ctrl Pts',(3.00365738718824,-2.76862191358616,-35.3877009587914));
#27032=CARTESIAN_POINT('Ctrl Pts',(2.92264128507332,-2.85651568210852,-35.3935084134559));
#27033=CARTESIAN_POINT('Ctrl Pts',(2.83779596670142,-2.94081581632806,-35.3993158681204));
#27034=CARTESIAN_POINT('Ctrl Pts',(2.74948306936067,-3.02118649727206,-35.405123322785));
#27035=CARTESIAN_POINT('Ctrl Pts',(2.66107282964314,-3.10164576633108,-35.4109371786826));
#27036=CARTESIAN_POINT('Ctrl Pts',(2.56918768375993,-3.17816666203462,-35.4167510345802));
#27037=CARTESIAN_POINT('Ctrl Pts',(2.47422279488574,-3.2504532855077,-35.4225648904778));
#27038=CARTESIAN_POINT('Ctrl Pts',(2.3791954263768,-3.32278746805114,-35.428382571448));
#27039=CARTESIAN_POINT('Ctrl Pts',(2.28108461392576,-3.39088159813571,-35.4342002524182));
#27040=CARTESIAN_POINT('Ctrl Pts',(2.18031358449793,-3.45448370574444,-35.4400179333884));
#27041=CARTESIAN_POINT('Ctrl Pts',(2.07939976292653,-3.51817593728394,-35.4458438579892));
#27042=CARTESIAN_POINT('Ctrl Pts',(1.97581855388177,-3.57736324060849,-35.4516697825899));
#27043=CARTESIAN_POINT('Ctrl Pts',(1.87001687863024,-3.63184001212031,-35.4574957071907));
#27044=CARTESIAN_POINT('Ctrl Pts',(1.844968020134,-3.64473754836146,-35.4588750120135));
#27045=CARTESIAN_POINT('Ctrl Pts',(1.81979478230675,-3.65737126489159,-35.4602543168362));
#27046=CARTESIAN_POINT('Ctrl Pts',(1.79450323923852,-3.66973883598853,-35.461633621659));
#27047=CARTESIAN_POINT('Ctrl Pts',(1.68768517348913,-3.721972897747,-35.4674590737816));
#27048=CARTESIAN_POINT('Ctrl Pts',(1.57841371056643,-3.76962278931479,-35.4732845259041));
#27049=CARTESIAN_POINT('Ctrl Pts',(1.4671190004969,-3.81245155226673,-35.4791099780267));
#27050=CARTESIAN_POINT('Ctrl Pts',(1.35596398381554,-3.85522655799154,-35.4849281182371));
#27051=CARTESIAN_POINT('Ctrl Pts',(1.24279114860668,-3.89319232601522,-35.4907462584475));
#27052=CARTESIAN_POINT('Ctrl Pts',(1.12805417629044,-3.92615827181657,-35.4965643986578));
#27053=CARTESIAN_POINT('Ctrl Pts',(1.01343137144864,-3.95909141529886,-35.5023767496064));
#27054=CARTESIAN_POINT('Ctrl Pts',(0.897247915708348,-3.98703452188866,
-35.508189100555));
#27055=CARTESIAN_POINT('Ctrl Pts',(0.779975796753611,-4.00984572726665,
-35.5140014515035));
#27056=CARTESIAN_POINT('Ctrl Pts',(0.658742672748291,-4.03342740818918,
-35.5200101215062));
#27057=CARTESIAN_POINT('Ctrl Pts',(0.536346456490509,-4.05152421987872,
-35.5260187915088));
#27058=CARTESIAN_POINT('Ctrl Pts',(0.413324171960105,-4.06403594089342,
-35.5320274615114));
#27059=CARTESIAN_POINT('Ctrl Pts',(0.294453895636837,-4.07612539070306,
-35.5378333386034));
#27060=CARTESIAN_POINT('Ctrl Pts',(0.174999567079131,-4.08300061619102,
-35.5436392156953));
#27061=CARTESIAN_POINT('Ctrl Pts',(0.0554535665679267,-4.08462359366869,
-35.5494450927872));
#27062=CARTESIAN_POINT('Ctrl Pts',(-0.0640751120410736,-4.08624633598117,
-35.5552501286227));
#27063=CARTESIAN_POINT('Ctrl Pts',(-0.183695028315242,-4.08261833826464,
-35.5610551644582));
#27064=CARTESIAN_POINT('Ctrl Pts',(-0.302912381463827,-4.07375368538108,
-35.5668602002938));
#27065=CARTESIAN_POINT('Ctrl Pts',(-0.422140540992919,-4.06488822896674,
-35.572665762323));
#27066=CARTESIAN_POINT('Ctrl Pts',(-0.540965657934851,-4.0507852038775,
-35.5784713243523));
#27067=CARTESIAN_POINT('Ctrl Pts',(-0.658898275603472,-4.03151064272523,
-35.5842768863816));
#27068=CARTESIAN_POINT('Ctrl Pts',(-0.776869361039087,-4.01222979451393,
-35.590084342094));
#27069=CARTESIAN_POINT('Ctrl Pts',(-0.893946965763019,-3.9877741211649,
-35.5958917978064));
#27070=CARTESIAN_POINT('Ctrl Pts',(-1.00965168584978,-3.9582607889401,-35.6016992535188));
#27071=CARTESIAN_POINT('Ctrl Pts',(-1.12548394058473,-3.9287149258692,-35.6075131104551));
#27072=CARTESIAN_POINT('Ctrl Pts',(-1.23993989458916,-3.8941003773362,-35.6133269673914));
#27073=CARTESIAN_POINT('Ctrl Pts',(-1.35255502787744,-3.85458427026359,
-35.6191408243277));
#27074=CARTESIAN_POINT('Ctrl Pts',(-1.46524425321756,-3.81504216464736,
-35.6249585063325));
#27075=CARTESIAN_POINT('Ctrl Pts',(-1.5760898680173,-3.77059222953675,-35.6307761883372));
#27076=CARTESIAN_POINT('Ctrl Pts',(-1.68464858914159,-3.72144919770555,
-35.6365938703419));
#27077=CARTESIAN_POINT('Ctrl Pts',(-1.79336113725128,-3.67223653052527,
-35.6424197959634));
#27078=CARTESIAN_POINT('Ctrl Pts',(-1.89977996141944,-3.61831767766219,
-35.6482457215848));
#27079=CARTESIAN_POINT('Ctrl Pts',(-2.00348745511604,-3.55995267063941,
-35.6540716472062));
#27080=CARTESIAN_POINT('Ctrl Pts',(-2.02804032700518,-3.54613468614128,
-35.6554509419931));
#27081=CARTESIAN_POINT('Ctrl Pts',(-2.05244135994231,-3.53206767651095,
-35.65683023678));
#27082=CARTESIAN_POINT('Ctrl Pts',(-2.07668526966656,-3.51775543361813,
-35.6582095315669));
#27083=CARTESIAN_POINT('Ctrl Pts',(-2.1790793810782,-3.45730770014667,-35.6640349807492));
#27084=CARTESIAN_POINT('Ctrl Pts',(-2.27899585314593,-3.39228885905836,
-35.6698604299315));
#27085=CARTESIAN_POINT('Ctrl Pts',(-2.37600012791215,-3.32292768385974,
-35.6756858791139));
#27086=CARTESIAN_POINT('Ctrl Pts',(-2.47288264606866,-3.2536535685516,-35.6815040163819));
#27087=CARTESIAN_POINT('Ctrl Pts',(-2.56685990835396,-3.18004819524483,
-35.6873221536499));
#27088=CARTESIAN_POINT('Ctrl Pts',(-2.65752312928818,-3.10238550430123,
-35.693140290918));
#27089=CARTESIAN_POINT('Ctrl Pts',(-2.74809613698508,-3.02480009058974,
-35.6989526389255));
#27090=CARTESIAN_POINT('Ctrl Pts',(-2.83536135550246,-2.94316565481485,
-35.7047649869331));
#27091=CARTESIAN_POINT('Ctrl Pts',(-2.91894060623687,-2.85779823242677,
-35.7105773349407));
#27092=CARTESIAN_POINT('Ctrl Pts',(-3.00534290497359,-2.76954736314105,
-35.7165860060463));
#27093=CARTESIAN_POINT('Ctrl Pts',(-3.08780546588963,-2.67730712428515,
-35.7225946771519));
#27094=CARTESIAN_POINT('Ctrl Pts',(-3.16594909253999,-2.58147077137147,
-35.7286033482575));
#27095=CARTESIAN_POINT('Ctrl Pts',(-3.24145531609227,-2.48886896367815,
-35.7344092224305));
#27096=CARTESIAN_POINT('Ctrl Pts',(-3.31292915685849,-2.39291020915543,
-35.7402150966034));
#27097=CARTESIAN_POINT('Ctrl Pts',(-3.38006791958474,-2.29398471202275,
-35.7460209707764));
#27098=CARTESIAN_POINT('Ctrl Pts',(-3.44719695422765,-2.19507354871812,
-35.7518260037061));
#27099=CARTESIAN_POINT('Ctrl Pts',(-3.5099919309662,-2.09319683522284,-35.7576310366359));
#27100=CARTESIAN_POINT('Ctrl Pts',(-3.56819288252017,-1.98877463608433,
-35.7634360695656));
#27101=CARTESIAN_POINT('Ctrl Pts',(-3.62639910982831,-1.88434297136432,
-35.7692416287054));
#27102=CARTESIAN_POINT('Ctrl Pts',(-3.68001028532705,-1.77736571864468,
-35.7750471878452));
#27103=CARTESIAN_POINT('Ctrl Pts',(-3.72881220759218,-1.6682879009666,-35.7808527469851));
#27104=CARTESIAN_POINT('Ctrl Pts',(-3.77763004844898,-1.55917450343512,
-35.7866601998274));
#27105=CARTESIAN_POINT('Ctrl Pts',(-3.82163534966172,-1.44795955050639,
-35.7924676526698));
#27106=CARTESIAN_POINT('Ctrl Pts',(-3.86066213725814,-1.33510780910808,
-35.7982751055122));
#27107=CARTESIAN_POINT('Ctrl Pts',(-3.89973194214464,-1.22213167683893,
-35.8040889596215));
#27108=CARTESIAN_POINT('Ctrl Pts',(-3.93381214655235,-1.10751554075407,
-35.8099028137307));
#27109=CARTESIAN_POINT('Ctrl Pts',(-3.96278668303157,-0.991739232251915,
-35.81571666784));
#27110=CARTESIAN_POINT('Ctrl Pts',(-3.99178028263405,-0.875886751416868,
-35.8215343470396));
#27111=CARTESIAN_POINT('Ctrl Pts',(-4.01566144296388,-0.758872976833628,
-35.8273520262391));
#27112=CARTESIAN_POINT('Ctrl Pts',(-4.03436553274525,-0.64118620399781,
-35.8331697054386));
#27113=CARTESIAN_POINT('Ctrl Pts',(-4.05309612627992,-0.523332668639482,
-35.8389956283077));
#27114=CARTESIAN_POINT('Ctrl Pts',(-4.06663496159447,-0.404804635581587,
-35.8448215511767));
#27115=CARTESIAN_POINT('Ctrl Pts',(-4.07496936030051,-0.286093887757309,
-35.8506474740457));
#27116=CARTESIAN_POINT('Ctrl Pts',(-4.07694257960332,-0.257988400208571,
-35.8520267965221));
#27117=CARTESIAN_POINT('Ctrl Pts',(-4.07862430221465,-0.229872661637646,
-35.8534061189984));
#27118=CARTESIAN_POINT('Ctrl Pts',(-4.08001478647782,-0.201753171281986,
-35.8547854414747));
#27119=CARTESIAN_POINT('Ctrl Pts',(-4.08331782992595,-0.134956371890456,
-35.858061970515));
#27120=CARTESIAN_POINT('Ctrl Pts',(-4.08498061775683,-0.0680778031167455,
-35.8613384995552));
#27121=CARTESIAN_POINT('Ctrl Pts',(-4.08499983154831,-0.00117313693436384,
-35.8646150285955));
#27122=CARTESIAN_POINT('Ctrl Pts',(-4.08499983154849,-0.00117313631325986,
-35.8646150286259));
#27123=CARTESIAN_POINT('Ctrl Pts',(-4.08503373102818,0.116868874034736,
-35.8703959120372));
#27124=CARTESIAN_POINT('Ctrl Pts',(-4.07994688931445,0.235111042198397,
-35.8761767954485));
#27125=CARTESIAN_POINT('Ctrl Pts',(-4.06971340855855,0.353069075676062,
-35.8819576788598));
#27126=CARTESIAN_POINT('Ctrl Pts',(-4.05949248493801,0.470882367102661,
-35.8877314687574));
#27127=CARTESIAN_POINT('Ctrl Pts',(-4.04413751518853,0.588411807383864,
-35.8935052586551));
#27128=CARTESIAN_POINT('Ctrl Pts',(-4.02367460274052,0.705172100455546,
-35.8992790485527));
#27129=CARTESIAN_POINT('Ctrl Pts',(-4.00323126266263,0.82182071462144,-35.9050473159348));
#27130=CARTESIAN_POINT('Ctrl Pts',(-3.97768976799366,0.937701238296356,
-35.9108155833168));
#27131=CARTESIAN_POINT('Ctrl Pts',(-3.94712805194677,1.0523331894105,-35.9165838506989));
#27132=CARTESIAN_POINT('Ctrl Pts',(-3.91658616023214,1.16689078272738,-35.9223483764046));
#27133=CARTESIAN_POINT('Ctrl Pts',(-3.88103063010538,1.28020101451192,-35.9281129021103));
#27134=CARTESIAN_POINT('Ctrl Pts',(-3.84059040645634,1.39179392506057,-35.9338774278161));
#27135=CARTESIAN_POINT('Ctrl Pts',(-3.80016369775302,1.50334954174702,-35.9396400270426));
#27136=CARTESIAN_POINT('Ctrl Pts',(-3.75485568164683,1.6131885883631,-35.945402626269));
#27137=CARTESIAN_POINT('Ctrl Pts',(-3.70484486777294,1.72085720085558,-35.9511652254955));
#27138=CARTESIAN_POINT('Ctrl Pts',(-3.65483852056453,1.82851619703436,-35.9569273100413));
#27139=CARTESIAN_POINT('Ctrl Pts',(-3.60013038570784,1.93400476833678,-35.962689394587));
#27140=CARTESIAN_POINT('Ctrl Pts',(-3.54094643027633,2.03689061510757,-35.9684514791327));
#27141=CARTESIAN_POINT('Ctrl Pts',(-3.48175326739319,2.13979246818365,-35.9742144601058));
#27142=CARTESIAN_POINT('Ctrl Pts',(-3.41808310698881,2.24009043237277,-35.9799774410789));
#27143=CARTESIAN_POINT('Ctrl Pts',(-3.3502066488331,2.33737896159662,-35.9857404220519));
#27144=CARTESIAN_POINT('Ctrl Pts',(-3.28226204563824,2.43476516431158,-35.9915091888095));
#27145=CARTESIAN_POINT('Ctrl Pts',(-3.21010294911753,2.52913555748799,-35.9972779555672));
#27146=CARTESIAN_POINT('Ctrl Pts',(-3.13404206357346,2.62011552107006,-36.0030467223248));
#27147=CARTESIAN_POINT('Ctrl Pts',(-3.05794147341163,2.71114297719249,-36.008818500442));
#27148=CARTESIAN_POINT('Ctrl Pts',(-2.97793531758722,2.79877617279207,-36.0145902785593));
#27149=CARTESIAN_POINT('Ctrl Pts',(-2.89437384388307,2.88267671649902,-36.0203620566765));
#27150=CARTESIAN_POINT('Ctrl Pts',(-2.81068169672052,2.96670846390213,-36.0261428607022));
#27151=CARTESIAN_POINT('Ctrl Pts',(-2.72342343142299,3.04699561907668,-36.0319236647278));
#27152=CARTESIAN_POINT('Ctrl Pts',(-2.63298340357745,3.12323924739775,-36.0377044687535));
#27153=CARTESIAN_POINT('Ctrl Pts',(-2.56176327342611,3.18327993139126,-36.0422567629632));
#27154=CARTESIAN_POINT('Ctrl Pts',(-2.48857073233364,3.24081387347772,-36.0468090571729));
#27155=CARTESIAN_POINT('Ctrl Pts',(-2.41360551266508,3.29571440346896,-36.0513613513826));
#27156=CARTESIAN_POINT('Ctrl Pts',(-2.31767438385452,3.36596924748385,-36.0571868091634));
#27157=CARTESIAN_POINT('Ctrl Pts',(-2.21851980173033,3.43214448006078,-36.0630122669443));
#27158=CARTESIAN_POINT('Ctrl Pts',(-2.11652338183446,3.49393099161217,-36.0688377247252));
#27159=CARTESIAN_POINT('Ctrl Pts',(-2.01465498384444,3.5556399511576,-36.07465587062));
#27160=CARTESIAN_POINT('Ctrl Pts',(-1.90995218878251,3.6129709367171,-36.0804740165147));
#27161=CARTESIAN_POINT('Ctrl Pts',(-1.802827953626,3.66565633545,-36.0862921624095));
#27162=CARTESIAN_POINT('Ctrl Pts',(-1.6958103105392,3.71828931051157,-36.0921045190614));
#27163=CARTESIAN_POINT('Ctrl Pts',(-1.58637638474194,3.7662857157977,-36.0979168757133));
#27164=CARTESIAN_POINT('Ctrl Pts',(-1.47496574524972,3.80942266627634,-36.1037292323652));
#27165=CARTESIAN_POINT('Ctrl Pts',(-1.35979223299051,3.85401655890115,-36.1097379002371));
#27166=CARTESIAN_POINT('Ctrl Pts',(-1.24250649722304,3.89341670215756,-36.115746568109));
#27167=CARTESIAN_POINT('Ctrl Pts',(-1.12361946629171,3.92742973138544,-36.1217552359808));
#27168=CARTESIAN_POINT('Ctrl Pts',(-1.00874472476286,3.96029486318795,-36.1275611187866));
#27169=CARTESIAN_POINT('Ctrl Pts',(-0.892375451068235,3.98813050942876,
-36.1333670015924));
#27170=CARTESIAN_POINT('Ctrl Pts',(-0.774989601447213,4.01081240120361,
-36.1391728843982));
#27171=CARTESIAN_POINT('Ctrl Pts',(-0.657620760834644,4.03349100641122,
-36.1449779259415));
#27172=CARTESIAN_POINT('Ctrl Pts',(-0.539236037740283,4.05101726491168,
-36.1507829674848));
#27173=CARTESIAN_POINT('Ctrl Pts',(-0.420323977030102,4.06331794895915,
-36.1565880090282));
#27174=CARTESIAN_POINT('Ctrl Pts',(-0.301401137875816,4.07561974796699,
-36.1623935767529));
#27175=CARTESIAN_POINT('Ctrl Pts',(-0.181951271937012,4.08269498879295,
-36.1681991444776));
#27176=CARTESIAN_POINT('Ctrl Pts',(-0.0624678101101076,4.08452234327345,
-36.1740047122023));
#27177=CARTESIAN_POINT('Ctrl Pts',(0.0570546249246556,4.08635029380185,
-36.1798121735916));
#27178=CARTESIAN_POINT('Ctrl Pts',(0.176610269889323,4.08292694740399,-36.1856196349809));
#27179=CARTESIAN_POINT('Ctrl Pts',(0.295706570594373,4.07428308099809,-36.1914270963702));
#27180=CARTESIAN_POINT('Ctrl Pts',(0.414934143016387,4.0656296870487,-36.1972409589275));
#27181=CARTESIAN_POINT('Ctrl Pts',(0.533700953405311,4.0517443169522,-36.2030548214848));
#27182=CARTESIAN_POINT('Ctrl Pts',(0.651520286599236,4.03270955018455,-36.2088686840421));
#27183=CARTESIAN_POINT('Ctrl Pts',(0.769417135199933,4.01366226010982,-36.2146863716415));
#27184=CARTESIAN_POINT('Ctrl Pts',(0.886364866532126,3.98945890871128,-36.220504059241));
#27185=CARTESIAN_POINT('Ctrl Pts',(1.00188927308175,3.96023268059892,-36.2263217468405));
#27186=CARTESIAN_POINT('Ctrl Pts',(1.11757737519665,3.93096503955855,-36.2321476779765));
#27187=CARTESIAN_POINT('Ctrl Pts',(1.23183773787284,3.89666043349518,-36.2379736091124));
#27188=CARTESIAN_POINT('Ctrl Pts',(1.34421343830507,3.85750116426166,-36.2437995402484));
#27189=CARTESIAN_POINT('Ctrl Pts',(1.3708174431377,3.84823053561219,-36.2451787805957));
#27190=CARTESIAN_POINT('Ctrl Pts',(1.39731591818232,3.83868802715506,-36.2465580209431));
#27191=CARTESIAN_POINT('Ctrl Pts',(1.42370299393941,3.82887643898937,-36.2479372612904));
#27192=CARTESIAN_POINT('Ctrl Pts',(1.53513902979679,3.78744083237973,-36.2537619717743));
#27193=CARTESIAN_POINT('Ctrl Pts',(1.64494289311034,3.7410700433615,-36.2595866822581));
#27194=CARTESIAN_POINT('Ctrl Pts',(1.75264666459632,3.68991255574972,-36.265411392742));
#27195=CARTESIAN_POINT('Ctrl Pts',(1.86023165407244,3.63881148760323,-36.271229679395));
#27196=CARTESIAN_POINT('Ctrl Pts',(1.96572079000933,3.58293438695173,-36.2770479660479));
#27197=CARTESIAN_POINT('Ctrl Pts',(2.06866334150336,3.52247881179151,-36.2828662527009));
#27198=CARTESIAN_POINT('Ctrl Pts',(2.17149549035802,3.46208807332871,-36.2886782994249));
#27199=CARTESIAN_POINT('Ctrl Pts',(2.2717861402928,3.39712883799668,-36.2944903461489));
#27200=CARTESIAN_POINT('Ctrl Pts',(2.36910736359178,3.3278454440937,-36.300302392873));
#27201=CARTESIAN_POINT('Ctrl Pts',(2.40893026840626,3.29949534832737,-36.3026806262698));
#27202=CARTESIAN_POINT('Ctrl Pts',(2.44825626195152,3.27042176671815,-36.3050588596666));
#27203=CARTESIAN_POINT('Ctrl Pts',(2.4870572760686,3.24064362520075,-36.3074370930634));
#27204=CARTESIAN_POINT('',(-4.08499997274305,-0.000471899681166237,-35.7603849713613));
#27205=CARTESIAN_POINT('Ctrl Pts',(-4.08499997274315,-0.000471898789758368,
-35.7603849714045));
#27206=CARTESIAN_POINT('Ctrl Pts',(-4.08501433561535,0.123860550885335,
-35.7664085457386));
#27207=CARTESIAN_POINT('Ctrl Pts',(-4.07934803225326,0.248109173627762,
-35.7724321200727));
#27208=CARTESIAN_POINT('Ctrl Pts',(-4.06804995739247,0.371745267836846,
-35.7784556944068));
#27209=CARTESIAN_POINT('Ctrl Pts',(-4.0567401997084,0.495509208485071,-35.7844854974441));
#27210=CARTESIAN_POINT('Ctrl Pts',(-4.03978709161203,0.618658998081323,
-35.7905153004814));
#27211=CARTESIAN_POINT('Ctrl Pts',(-4.01729103004486,0.740673868798626,
-35.7965451035186));
#27212=CARTESIAN_POINT('Ctrl Pts',(-3.99474910373659,0.862937502191047,
-35.8025872000569));
#27213=CARTESIAN_POINT('Ctrl Pts',(-3.96664170401674,0.984061236009943,
-35.8086292965951));
#27214=CARTESIAN_POINT('Ctrl Pts',(-3.93312004227064,1.10353601349887,-35.8146713931334));
#27215=CARTESIAN_POINT('Ctrl Pts',(-3.89956210969393,1.22314006409633,-35.8207200272909));
#27216=CARTESIAN_POINT('Ctrl Pts',(-3.86057834267863,1.34109125660982,-35.8267686614483));
#27217=CARTESIAN_POINT('Ctrl Pts',(-3.8163687679715,1.45689890756076,-35.8328172956058));
#27218=CARTESIAN_POINT('Ctrl Pts',(-3.77206545519309,1.57295210681002,-35.8388787547521));
#27219=CARTESIAN_POINT('Ctrl Pts',(-3.72251432922099,1.68685234722564,-35.8449402138983));
#27220=CARTESIAN_POINT('Ctrl Pts',(-3.66796273133031,1.79813080769222,-35.8510016730446));
#27221=CARTESIAN_POINT('Ctrl Pts',(-3.63185957703299,1.87177674261505,-35.8550132474675));
#27222=CARTESIAN_POINT('Ctrl Pts',(-3.59356715360858,1.94427485830153,-35.8590248218903));
#27223=CARTESIAN_POINT('Ctrl Pts',(-3.55316758175896,2.01549625053911,-35.8630363963132));
#27224=CARTESIAN_POINT('Ctrl Pts',(-3.49450089718306,2.11892118209559,-35.8688618484292));
#27225=CARTESIAN_POINT('Ctrl Pts',(-3.43122090777399,2.2199479492658,-35.8746873005453));
#27226=CARTESIAN_POINT('Ctrl Pts',(-3.36354883275847,2.31813809977946,-35.8805127526613));
#27227=CARTESIAN_POINT('Ctrl Pts',(-3.29596169746274,2.41620500530811,-35.8863308928651));
#27228=CARTESIAN_POINT('Ctrl Pts',(-3.22399367114155,2.51144204289252,-35.892149033069));
#27229=CARTESIAN_POINT('Ctrl Pts',(-3.14791157911544,2.60343574725226,-35.8979671732728));
#27230=CARTESIAN_POINT('Ctrl Pts',(-3.07190519154733,2.69533791451908,-35.9037795242149));
#27231=CARTESIAN_POINT('Ctrl Pts',(-2.99179314080898,2.78400285624025,-35.9095918751569));
#27232=CARTESIAN_POINT('Ctrl Pts',(-2.90788487067213,2.86904698095311,-35.9154042260989));
#27233=CARTESIAN_POINT('Ctrl Pts',(-2.82114249895735,2.95696357208256,-35.921412896104));
#27234=CARTESIAN_POINT('Ctrl Pts',(-2.73034317695568,3.04101005616904,-35.9274215661091));
#27235=CARTESIAN_POINT('Ctrl Pts',(-2.63587353853775,3.1208004884703,-35.9334302361142));
#27236=CARTESIAN_POINT('Ctrl Pts',(-2.54459225524385,3.19789798960409,-35.9392361131996));
#27237=CARTESIAN_POINT('Ctrl Pts',(-2.44988474113596,3.27102180295613,-35.9450419902849));
#27238=CARTESIAN_POINT('Ctrl Pts',(-2.35213590391129,3.33986252554375,-35.9508478673703));
#27239=CARTESIAN_POINT('Ctrl Pts',(-2.25440123023684,3.40869327329115,-35.9566529031993));
#27240=CARTESIAN_POINT('Ctrl Pts',(-2.15362644335434,3.47324192964129,-35.9624579390283));
#27241=CARTESIAN_POINT('Ctrl Pts',(-2.05022704626308,3.53324129642618,-35.9682629748573));
#27242=CARTESIAN_POINT('Ctrl Pts',(-1.94681827659931,3.59324610181547,-35.9740685368801));
#27243=CARTESIAN_POINT('Ctrl Pts',(-1.84078477663318,3.64870059296511,-35.9798740989029));
#27244=CARTESIAN_POINT('Ctrl Pts',(-1.73256779614466,3.69938289877683,-35.9856796609256));
#27245=CARTESIAN_POINT('Ctrl Pts',(-1.62431551697691,3.75008173636061,-35.9914871166316));
#27246=CARTESIAN_POINT('Ctrl Pts',(-1.51387871013573,3.7960051198592,-35.9972945723375));
#27247=CARTESIAN_POINT('Ctrl Pts',(-1.40171920096156,3.8369790567132,-36.0031020280434));
#27248=CARTESIAN_POINT('Ctrl Pts',(-1.28943606481925,3.87799815677826,-36.0089158849733));
#27249=CARTESIAN_POINT('Ctrl Pts',(-1.17542681963514,3.91405678070922,-36.0147297419032));
#27250=CARTESIAN_POINT('Ctrl Pts',(-1.0601692166547,3.94503057428682,-36.0205435988331));
#27251=CARTESIAN_POINT('Ctrl Pts',(-0.944835783080895,3.97602474622632,
-36.0263612808315));
#27252=CARTESIAN_POINT('Ctrl Pts',(-0.82825275337201,4.00192733692282,-36.0321789628299));
#27253=CARTESIAN_POINT('Ctrl Pts',(-0.710907231777638,4.02266527414428,
-36.0379966448282));
#27254=CARTESIAN_POINT('Ctrl Pts',(-0.593395432357713,4.04343259688519,
-36.0438225704434));
#27255=CARTESIAN_POINT('Ctrl Pts',(-0.475119387659319,4.05902060671436,
-36.0496484960586));
#27256=CARTESIAN_POINT('Ctrl Pts',(-0.356570587963855,4.06940811615143,
-36.0554744216737));
#27257=CARTESIAN_POINT('Ctrl Pts',(-0.328504018016518,4.07186737141966,
-36.0568537165228));
#27258=CARTESIAN_POINT('Ctrl Pts',(-0.300422154589264,4.07403536270349,
-36.0582330113719));
#27259=CARTESIAN_POINT('Ctrl Pts',(-0.272331500023082,4.07591223581853,
-36.059612306221));
#27260=CARTESIAN_POINT('Ctrl Pts',(-0.150652121165061,4.08404222632104,
-36.0655869530596));
#27261=CARTESIAN_POINT('Ctrl Pts',(-0.0284087048904191,4.08673200763319,
-36.0715615998983));
#27262=CARTESIAN_POINT('Ctrl Pts',(0.0938723505112838,4.08392127517286,
-36.0775362467369));
#27263=CARTESIAN_POINT('Ctrl Pts',(0.212929860204959,4.08118463861012,-36.083353391278));
#27264=CARTESIAN_POINT('Ctrl Pts',(0.332022605367885,4.07323384029929,-36.0891705358191));
#27265=CARTESIAN_POINT('Ctrl Pts',(0.450658698680455,4.06006548436151,-36.0949876803602));
#27266=CARTESIAN_POINT('Ctrl Pts',(0.569186150230049,4.04690918743009,-36.1007994978139));
#27267=CARTESIAN_POINT('Ctrl Pts',(0.687257378507995,4.02854487922045,-36.1066113152676));
#27268=CARTESIAN_POINT('Ctrl Pts',(0.804382026689269,4.00502116787655,-36.1124231327213));
#27269=CARTESIAN_POINT('Ctrl Pts',(0.921427010307248,3.98151345663358,-36.1182309971565));
#27270=CARTESIAN_POINT('Ctrl Pts',(1.03752629592987,3.95285340288052,-36.1240388615917));
#27271=CARTESIAN_POINT('Ctrl Pts',(1.1521968018633,3.91914117247338,-36.1298467260269));
#27272=CARTESIAN_POINT('Ctrl Pts',(1.2725646562154,3.88375396626459,-36.135943151387));
#27273=CARTESIAN_POINT('Ctrl Pts',(1.39135763936013,3.84279971606564,-36.1420395767472));
#27274=CARTESIAN_POINT('Ctrl Pts',(1.50803172254238,3.79645430945848,-36.1481360021073));
#27275=CARTESIAN_POINT('Ctrl Pts',(1.61912987400424,3.75232378053234,-36.1539410752612));
#27276=CARTESIAN_POINT('Ctrl Pts',(1.72830655847884,3.70330564643782,-36.1597461484151));
#27277=CARTESIAN_POINT('Ctrl Pts',(1.8351108847196,3.64960176468387,-36.165551221569));
#27278=CARTESIAN_POINT('Ctrl Pts',(1.94191608605904,3.59589744290847,-36.1713563422866));
#27279=CARTESIAN_POINT('Ctrl Pts',(2.04634852902581,3.5375074861917,-36.1771614630042));
#27280=CARTESIAN_POINT('Ctrl Pts',(2.14798132902517,3.47468001550636,-36.1829665837219));
#27281=CARTESIAN_POINT('Ctrl Pts',(2.24966183811596,3.41182305196494,-36.1887744295148));
#27282=CARTESIAN_POINT('Ctrl Pts',(2.34853973848285,3.34452463795732,-36.1945822753078));
#27283=CARTESIAN_POINT('Ctrl Pts',(2.44421682960853,3.27307639535933,-36.2003901211007));
#27284=CARTESIAN_POINT('Ctrl Pts',(2.45856937424092,3.26235842642101,-36.2012613575167));
#27285=CARTESIAN_POINT('Ctrl Pts',(2.47284994982935,3.25154714875453,-36.2021325939326));
#27286=CARTESIAN_POINT('Ctrl Pts',(2.4870572760686,3.24064362520075,-36.2030038303486));
#27287=CARTESIAN_POINT('Ctrl Pts',(2.48705727606859,3.24064362520075,-34.9531798329663));
#27288=CARTESIAN_POINT('Ctrl Pts',(2.58185257295869,3.16789223376906,-34.9589854944241));
#27289=CARTESIAN_POINT('Ctrl Pts',(2.67349144398005,3.09094849285946,-34.9647911558819));
#27290=CARTESIAN_POINT('Ctrl Pts',(2.76159033964477,3.01012355161391,-34.9705968173397));
#27291=CARTESIAN_POINT('Ctrl Pts',(2.84967960198705,2.92930744830796,-34.9764018439676));
#27292=CARTESIAN_POINT('Ctrl Pts',(2.93422935823234,2.84461126453053,-34.9822068705956));
#27293=CARTESIAN_POINT('Ctrl Pts',(3.0148909053675,2.75638492027735,-34.9880118972235));
#27294=CARTESIAN_POINT('Ctrl Pts',(3.09556263158334,2.66814744230421,-34.9938176564165));
#27295=CARTESIAN_POINT('Ctrl Pts',(3.17234489771808,2.57637921918024,-34.9996234156096));
#27296=CARTESIAN_POINT('Ctrl Pts',(3.24492791543381,2.48146485440322,-35.0054291748026));
#27297=CARTESIAN_POINT('Ctrl Pts',(3.31921376641181,2.38432375198843,-35.0113711399592));
#27298=CARTESIAN_POINT('Ctrl Pts',(3.38910060130646,2.28388740056329,-35.0173131051158));
#27299=CARTESIAN_POINT('Ctrl Pts',(3.45430273132409,2.18060029358132,-35.0232550702724));
#27300=CARTESIAN_POINT('Ctrl Pts',(3.51810542786156,2.07953003803565,-35.029069503016));
#27301=CARTESIAN_POINT('Ctrl Pts',(3.57742233900376,1.97573055458253,-35.0348839357595));
#27302=CARTESIAN_POINT('Ctrl Pts',(3.63203245277187,1.8696430841238,-35.0406983685031));
#27303=CARTESIAN_POINT('Ctrl Pts',(3.68843927480726,1.76006526687625,-35.0467040998662));
#27304=CARTESIAN_POINT('Ctrl Pts',(3.73982405310811,1.64804675411381,-35.0527098312293));
#27305=CARTESIAN_POINT('Ctrl Pts',(3.7859976477236,1.53409478567375,-35.0587155625925));
#27306=CARTESIAN_POINT('Ctrl Pts',(3.83217124233908,1.42014281723368,-35.0647212939556));
#27307=CARTESIAN_POINT('Ctrl Pts',(3.87313355733504,1.3042578606197,-35.0707270253187));
#27308=CARTESIAN_POINT('Ctrl Pts',(3.9087526211886,1.18696164485262,-35.0767327566819));
#27309=CARTESIAN_POINT('Ctrl Pts',(3.94330247076365,1.07318643090717,-35.0825582077953));
#27310=CARTESIAN_POINT('Ctrl Pts',(3.97293584875576,0.957719453854558,-35.0883836589087));
#27311=CARTESIAN_POINT('Ctrl Pts',(3.99748734984815,0.84102311966082,-35.0942091100221));
#27312=CARTESIAN_POINT('Ctrl Pts',(4.02200803469859,0.724473258892695,-35.1000272492196));
#27313=CARTESIAN_POINT('Ctrl Pts',(4.04145944653533,0.60669750594145,-35.1058453884172));
#27314=CARTESIAN_POINT('Ctrl Pts',(4.05572571045719,0.488174109858925,-35.1116635276147));
#27315=CARTESIAN_POINT('Ctrl Pts',(4.06997777891732,0.369768648951444,-35.1174758775479));
#27316=CARTESIAN_POINT('Ctrl Pts',(4.07905491520925,0.250617427705652,-35.1232882274811));
#27317=CARTESIAN_POINT('Ctrl Pts',(4.08289225877019,0.13120900607235,-35.1291005774144));
#27318=CARTESIAN_POINT('Ctrl Pts',(4.08685921410945,0.00776739386600114,
-35.1351092477967));
#27319=CARTESIAN_POINT('Ctrl Pts',(4.08522605676269,-0.115948666280446,
-35.141117918179));
#27320=CARTESIAN_POINT('Ctrl Pts',(4.07797939808869,-0.239393042430706,
-35.1471265885613));
#27321=CARTESIAN_POINT('Ctrl Pts',(4.07097731617103,-0.358671136371906,
-35.1529324646382));
#27322=CARTESIAN_POINT('Ctrl Pts',(4.05873455894428,-0.477695149436253,
-35.1587383407151));
#27323=CARTESIAN_POINT('Ctrl Pts',(4.04129202904109,-0.595972932278733,
-35.1645442167921));
#27324=CARTESIAN_POINT('Ctrl Pts',(4.02385202650952,-0.714233577016134,
-35.1703492516145));
#27325=CARTESIAN_POINT('Ctrl Pts',(4.0012138092065,-0.831747803024423,-35.176154286437));
#27326=CARTESIAN_POINT('Ctrl Pts',(3.97346994912334,-0.948030359964137,
-35.1819593212594));
#27327=CARTESIAN_POINT('Ctrl Pts',(3.94572357420098,-1.06432345732371,-35.1877648822786));
#27328=CARTESIAN_POINT('Ctrl Pts',(3.91287073103484,-1.17938426674482,-35.1935704432978));
#27329=CARTESIAN_POINT('Ctrl Pts',(3.87505458387088,-1.29274010227163,-35.199376004317));
#27330=CARTESIAN_POINT('Ctrl Pts',(3.83722610164495,-1.4061329127777,-35.2051834590235));
#27331=CARTESIAN_POINT('Ctrl Pts',(3.79443122469791,-1.51781925650291,-35.2109909137299));
#27332=CARTESIAN_POINT('Ctrl Pts',(3.74686199638506,-1.62734451793263,-35.2167983684364));
#27333=CARTESIAN_POINT('Ctrl Pts',(3.69924033515195,-1.73699050297933,-35.2226122243778));
#27334=CARTESIAN_POINT('Ctrl Pts',(3.64683398098893,-1.84447027662019,-35.2284260803192));
#27335=CARTESIAN_POINT('Ctrl Pts',(3.58988192869939,-1.94935187639316,-35.2342399362607));
#27336=CARTESIAN_POINT('Ctrl Pts',(3.53289240630361,-2.05430248025867,-35.2400576172759));
#27337=CARTESIAN_POINT('Ctrl Pts',(3.47135143935218,-2.15665115703625,-35.2458752982911));
#27338=CARTESIAN_POINT('Ctrl Pts',(3.40554163728126,-2.25599449395242,-35.2516929793063));
#27339=CARTESIAN_POINT('Ctrl Pts',(3.33963858297056,-2.3554786,-35.2575189039534));
#27340=CARTESIAN_POINT('Ctrl Pts',(3.26945485984531,-2.45194853794407,-35.2633448286005));
#27341=CARTESIAN_POINT('Ctrl Pts',(3.19531370704236,-2.54503346020975,-35.2691707532476));
#27342=CARTESIAN_POINT('Ctrl Pts',(3.17776057548174,-2.56707158377632,-35.2705500576949));
#27343=CARTESIAN_POINT('Ctrl Pts',(3.15998578540621,-2.58892013290523,-35.2719293621423));
#27344=CARTESIAN_POINT('Ctrl Pts',(3.14199392218859,-2.61057449480568,-35.2733086665896));
#27345=CARTESIAN_POINT('Ctrl Pts',(3.06600582348427,-2.70203104766893,-35.2791341178629));
#27346=CARTESIAN_POINT('Ctrl Pts',(2.98589970471296,-2.7903133811064,-35.2849595691361));
#27347=CARTESIAN_POINT('Ctrl Pts',(2.90197064707861,-2.87502893263601,-35.2907850204093));
#27348=CARTESIAN_POINT('Ctrl Pts',(2.81814693444228,-2.95963815198628,-35.2966031597673));
#27349=CARTESIAN_POINT('Ctrl Pts',(2.73051011176688,-3.04068920674115,-35.3024212991253));
#27350=CARTESIAN_POINT('Ctrl Pts',(2.63939574446582,-3.11782217326385,-35.3082394384834));
#27351=CARTESIAN_POINT('Ctrl Pts',(2.54837203932978,-3.19487838963236,-35.3140517885776));
#27352=CARTESIAN_POINT('Ctrl Pts',(2.45387798317224,-3.26802401166205,-35.3198641386717));
#27353=CARTESIAN_POINT('Ctrl Pts',(2.35628582291631,-3.33693603785323,-35.3256764887659));
#27354=CARTESIAN_POINT('Ctrl Pts',(2.25539735138565,-3.40817566380552,-35.3316851590881));
#27355=CARTESIAN_POINT('Ctrl Pts',(2.15119809820872,-3.47489032488061,-35.3376938294102));
#27356=CARTESIAN_POINT('Ctrl Pts',(2.04413670567813,-3.53676831705151,-35.3437024997324));
#27357=CARTESIAN_POINT('Ctrl Pts',(1.94068866117255,-3.59655791194382,-35.3495083759704));
#27358=CARTESIAN_POINT('Ctrl Pts',(1.83456893706537,-3.65183182685612,-35.3553142522085));
#27359=CARTESIAN_POINT('Ctrl Pts',(1.72621097659092,-3.70235339538205,-35.3611201284465));
#27360=CARTESIAN_POINT('Ctrl Pts',(1.61786871687178,-3.75286764347871,-35.3669251634299));
#27361=CARTESIAN_POINT('Ctrl Pts',(1.50728923546747,-3.79863074227898,-35.3727301984132));
#27362=CARTESIAN_POINT('Ctrl Pts',(1.39492864762283,-3.83945296468666,-35.3785352333966));
#27363=CARTESIAN_POINT('Ctrl Pts',(1.28255787487331,-3.88027888741719,-35.3843407945762));
#27364=CARTESIAN_POINT('Ctrl Pts',(1.16840605819321,-3.91616290395843,-35.3901463557559));
#27365=CARTESIAN_POINT('Ctrl Pts',(1.05294666164762,-3.94696444469989,-35.3959519169356));
#27366=CARTESIAN_POINT('Ctrl Pts',(0.937449603985241,-3.9777760324402,-35.4017593718019));
#27367=CARTESIAN_POINT('Ctrl Pts',(0.82064451223023,-4.00350174218263,-35.4075668266683));
#27368=CARTESIAN_POINT('Ctrl Pts',(0.703016659107214,-4.02405176122496,
-35.4133742815346));
#27369=CARTESIAN_POINT('Ctrl Pts',(0.585259151366584,-4.04462443140637,
-35.4191881376343));
#27370=CARTESIAN_POINT('Ctrl Pts',(0.466677474225332,-4.06000995344015,
-35.425001993734));
#27371=CARTESIAN_POINT('Ctrl Pts',(0.347763821923251,-4.07017018368536,
-35.4308158498337));
#27372=CARTESIAN_POINT('Ctrl Pts',(0.228771933525952,-4.08033709858557,
-35.4366335310064));
#27373=CARTESIAN_POINT('Ctrl Pts',(0.109448041697635,-4.08527185822192,
-35.4424512121792));
#27374=CARTESIAN_POINT('Ctrl Pts',(-0.009715497563873,-4.0849884466308,
-35.4482688933519));
#27375=CARTESIAN_POINT('Ctrl Pts',(-0.129047891055146,-4.08470463344665,
-35.4540948181541));
#27376=CARTESIAN_POINT('Ctrl Pts',(-0.248219072395885,-4.07918791013412,
-35.4599207429563));
#27377=CARTESIAN_POINT('Ctrl Pts',(-0.366741519249476,-4.06850410569519,
-35.4657466677586));
#27378=CARTESIAN_POINT('Ctrl Pts',(-0.394802018096425,-4.06597468709054,
-35.4671259706716));
#27379=CARTESIAN_POINT('Ctrl Pts',(-0.422826199933721,-4.06315586969311,
-35.4685052735845));
#27380=CARTESIAN_POINT('Ctrl Pts',(-0.450807689956826,-4.06004894387688,
-35.4698845764975));
#27381=CARTESIAN_POINT('Ctrl Pts',(-0.56898680408474,-4.0469269214142,-35.4757100274021));
#27382=CARTESIAN_POINT('Ctrl Pts',(-0.686781564327053,-4.02861972549075,
-35.4815354783067));
#27383=CARTESIAN_POINT('Ctrl Pts',(-0.803701811597009,-4.00515772448922,
-35.4873609292113));
#27384=CARTESIAN_POINT('Ctrl Pts',(-0.920475304401193,-3.98172517222308,
-35.4931790682007));
#27385=CARTESIAN_POINT('Ctrl Pts',(-1.03637607093199,-3.95315076368354,
-35.4989972071901));
#27386=CARTESIAN_POINT('Ctrl Pts',(-1.1509189273156,-3.91951663126293,-35.5048153461795));
#27387=CARTESIAN_POINT('Ctrl Pts',(-1.26534780932296,-3.88591596604738,
-35.5106276959055));
#27388=CARTESIAN_POINT('Ctrl Pts',(-1.37842107995376,-3.84726570720263,
-35.5164400456315));
#27389=CARTESIAN_POINT('Ctrl Pts',(-1.48966419956015,-3.80369893295314,
-35.5222523953575));
#27390=CARTESIAN_POINT('Ctrl Pts',(-1.6046647205544,-3.75866062627441,-35.5282610658178));
#27391=CARTESIAN_POINT('Ctrl Pts',(-1.7177088345245,-3.70836788741373,-35.5342697362782));
#27392=CARTESIAN_POINT('Ctrl Pts',(-1.82828939612217,-3.65302380009044,
-35.5402784067385));
#27393=CARTESIAN_POINT('Ctrl Pts',(-1.93513782771306,-3.59954759375829,
-35.5460842826118));
#27394=CARTESIAN_POINT('Ctrl Pts',(-2.03968592103842,-3.54135570345619,
-35.551890158485));
#27395=CARTESIAN_POINT('Ctrl Pts',(-2.14149754958436,-3.47867981353906,
-35.5576960343583));
#27396=CARTESIAN_POINT('Ctrl Pts',(-2.24329442595143,-3.41601300515763,
-35.5635010689787));
#27397=CARTESIAN_POINT('Ctrl Pts',(-2.34235527872662,-3.34886370313172,
-35.5693061035992));
#27398=CARTESIAN_POINT('Ctrl Pts',(-2.4382706989037,-3.27750835221936,-35.5751111382196));
#27399=CARTESIAN_POINT('Ctrl Pts',(-2.53419481335538,-3.20614653328534,
-35.5809166990387));
#27400=CARTESIAN_POINT('Ctrl Pts',(-2.62697260094794,-3.13057815098081,
-35.5867222598578));
#27401=CARTESIAN_POINT('Ctrl Pts',(-2.71622615155643,-3.05112118631839,
-35.5925278206769));
#27402=CARTESIAN_POINT('Ctrl Pts',(-2.80550881537117,-2.97163830395315,
-35.5983352751853));
#27403=CARTESIAN_POINT('Ctrl Pts',(-2.89126465137951,-2.88826458779838,
-35.6041427296937));
#27404=CARTESIAN_POINT('Ctrl Pts',(-2.97315163245833,-2.8013558093199,-35.609950184202));
#27405=CARTESIAN_POINT('Ctrl Pts',(-3.05512887307286,-2.7143512360534,-35.6157640399495));
#27406=CARTESIAN_POINT('Ctrl Pts',(-3.13322846680991,-2.62380411998626,
-35.621577895697));
#27407=CARTESIAN_POINT('Ctrl Pts',(-3.2071477204704,-2.53010444430295,-35.6273917514445));
#27408=CARTESIAN_POINT('Ctrl Pts',(-3.28111560739103,-2.43634312134267,
-35.6332094322679));
#27409=CARTESIAN_POINT('Ctrl Pts',(-3.35089743891608,-2.33942543833364,
-35.6390271130913));
#27410=CARTESIAN_POINT('Ctrl Pts',(-3.41623395845745,-2.23977019827529,
-35.6448447939148));
#27411=CARTESIAN_POINT('Ctrl Pts',(-3.48166305965255,-2.13997374703839,
-35.6506707183746));
#27412=CARTESIAN_POINT('Ctrl Pts',(-3.54263406914116,-2.0374323459784,-35.6564966428345));
#27413=CARTESIAN_POINT('Ctrl Pts',(-3.59893367975997,-1.93258929125911,
-35.6623225672943));
#27414=CARTESIAN_POINT('Ctrl Pts',(-3.61226279381032,-1.90776736054981,
-35.6637018736646));
#27415=CARTESIAN_POINT('Ctrl Pts',(-3.62533027957415,-1.88281650320364,
-35.665081180035));
#27416=CARTESIAN_POINT('Ctrl Pts',(-3.63813370655198,-1.85774275217274,
-35.6664604864053));
#27417=CARTESIAN_POINT('Ctrl Pts',(-3.6955115031636,-1.74537622800449,-35.6726417658799));
#27418=CARTESIAN_POINT('Ctrl Pts',(-3.74774736328879,-1.63021694586954,
-35.6788230453544));
#27419=CARTESIAN_POINT('Ctrl Pts',(-3.79457835110188,-1.51274589318529,
-35.685004324829));
#27420=CARTESIAN_POINT('Ctrl Pts',(-3.84217030669429,-1.39336602562715,
-35.6912860453734));
#27421=CARTESIAN_POINT('Ctrl Pts',(-3.88417997960303,-1.27159886783622,
-35.6975677659177));
#27422=CARTESIAN_POINT('Ctrl Pts',(-3.92037933535891,-1.14797685816867,
-35.7038494864621));
#27423=CARTESIAN_POINT('Ctrl Pts',(-3.9558410409636,-1.02687394841927,-35.7100032016314));
#27424=CARTESIAN_POINT('Ctrl Pts',(-3.98572681192188,-0.903991386433874,
-35.7161569168008));
#27425=CARTESIAN_POINT('Ctrl Pts',(-4.00986993742051,-0.779851322350109,
-35.7223106319701));
#27426=CARTESIAN_POINT('Ctrl Pts',(-4.0347663761004,-0.651837843177621,
-35.728656355202));
#27427=CARTESIAN_POINT('Ctrl Pts',(-4.05355578670384,-0.522487414956089,
-35.7350020784338));
#27428=CARTESIAN_POINT('Ctrl Pts',(-4.06611043343708,-0.392391313734325,
-35.7413478016657));
#27429=CARTESIAN_POINT('Ctrl Pts',(-4.07866508017031,-0.262295212512561,
-35.7476935248976));
#27430=CARTESIAN_POINT('Ctrl Pts',(-4.08498484169645,-0.131453816830751,
-35.7540392481294));
#27431=CARTESIAN_POINT('Ctrl Pts',(-4.08499997274305,-0.000471899681166737,
-35.7603849713613));
#27432=CARTESIAN_POINT('Origin',(0.,0.,-25.2396150285955));
#27433=CARTESIAN_POINT('',(2.4870572760686,3.24064362520074,-33.7031235592767));
#27434=CARTESIAN_POINT('',(2.48364276907221,3.23615213332545,-33.8072572988311));
#27435=CARTESIAN_POINT('',(2.4870572760686,3.24064362520075,-25.2396150285955));
#27436=CARTESIAN_POINT('',(-4.08499870649295,0.00325083849409857,-34.6146150643215));
#27437=CARTESIAN_POINT('Ctrl Pts',(2.48364276907218,3.23615213332547,-33.8072572988311));
#27438=CARTESIAN_POINT('Ctrl Pts',(2.93053432606008,2.89620766874513,-33.8345136466862));
#27439=CARTESIAN_POINT('Ctrl Pts',(4.22102243221385,1.44257110886102,-33.9272952978439));
#27440=CARTESIAN_POINT('Ctrl Pts',(4.26353275186578,-2.23312212597346,-34.0856022523043));
#27441=CARTESIAN_POINT('Ctrl Pts',(0.481516845971146,-4.78880856471269,
-34.2821781622121));
#27442=CARTESIAN_POINT('Ctrl Pts',(-3.29963218394254,-3.21756865493895,
-34.4585157543092));
#27443=CARTESIAN_POINT('Ctrl Pts',(-4.07505368127094,-0.928043141231352,
-34.5693280431036));
#27444=CARTESIAN_POINT('Ctrl Pts',(-4.08219506199217,0.0032478726848344,
-34.6146150285955));
#27445=CARTESIAN_POINT('Ctrl Pts',(-4.08499870649295,0.00325083849409857,
-34.6146150643215));
#27446=CARTESIAN_POINT('Ctrl Pts',(-4.0848857285227,0.145218784049321,-34.6215140152461));
#27447=CARTESIAN_POINT('Ctrl Pts',(-4.07736808054459,0.286878155519986,
-34.6284129661707));
#27448=CARTESIAN_POINT('Ctrl Pts',(-4.06256514836033,0.427538788097697,
-34.6353119170953));
#27449=CARTESIAN_POINT('Ctrl Pts',(-4.04759363057255,0.569801357193021,
-34.6422894378459));
#27450=CARTESIAN_POINT('Ctrl Pts',(-4.02517001513738,0.711042259284884,
-34.6492669585965));
#27451=CARTESIAN_POINT('Ctrl Pts',(-3.9954672708171,0.850568214683206,-34.6562444793471));
#27452=CARTESIAN_POINT('Ctrl Pts',(-3.968385454481,0.977782597888755,-34.662606313574));
#27453=CARTESIAN_POINT('Ctrl Pts',(-3.93525307540227,1.10357157241974,-34.6689681478009));
#27454=CARTESIAN_POINT('Ctrl Pts',(-3.89623577907751,1.22742484651251,-34.6753299820277));
#27455=CARTESIAN_POINT('Ctrl Pts',(-3.86050813447011,1.34083572263829,-34.6811554331409));
#27456=CARTESIAN_POINT('Ctrl Pts',(-3.81976751612471,1.45286679822255,-34.6869808842541));
#27457=CARTESIAN_POINT('Ctrl Pts',(-3.7741385054851,1.56304303888752,-34.6928063353673));
#27458=CARTESIAN_POINT('Ctrl Pts',(-3.72856676688873,1.67308098993515,-34.6986244745646));
#27459=CARTESIAN_POINT('Ctrl Pts',(-3.67811899487606,1.78126836305931,-34.7044426137619));
#27460=CARTESIAN_POINT('Ctrl Pts',(-3.62296959571413,1.88714501523625,-34.7102607529592));
#27461=CARTESIAN_POINT('Ctrl Pts',(-3.5678750722497,1.99291631621757,-34.7160731028923));
#27462=CARTESIAN_POINT('Ctrl Pts',(-3.50808841614009,2.09638111060591,-34.7218854528253));
#27463=CARTESIAN_POINT('Ctrl Pts',(-3.44383195947611,2.19709955051903,-34.7276978027583));
#27464=CARTESIAN_POINT('Ctrl Pts',(-3.37740514889466,2.30121990009191,-34.7337064731407));
#27465=CARTESIAN_POINT('Ctrl Pts',(-3.30620141507986,2.40240467677481,-34.7397151435231));
#27466=CARTESIAN_POINT('Ctrl Pts',(-3.23051807941002,2.50019558007068,-34.7457238139055));
#27467=CARTESIAN_POINT('Ctrl Pts',(-3.15738907748324,2.59468601303393,-34.7515296899822));
#27468=CARTESIAN_POINT('Ctrl Pts',(-3.08007823973709,2.68600761593496,-34.7573355660589));
#27469=CARTESIAN_POINT('Ctrl Pts',(-2.99889721484469,2.77377729726032,-34.7631414421356));
#27470=CARTESIAN_POINT('Ctrl Pts',(-2.91772795284556,2.86153426101534,-34.7689464769578));
#27471=CARTESIAN_POINT('Ctrl Pts',(-2.83268989593037,2.94574002727901,-34.7747515117801));
#27472=CARTESIAN_POINT('Ctrl Pts',(-2.74413344169413,3.02604637343448,-34.7805565466023));
#27473=CARTESIAN_POINT('Ctrl Pts',(-2.65556896026765,3.10635999895002,-34.7863621076213));
#27474=CARTESIAN_POINT('Ctrl Pts',(-2.56348574968054,3.18277322748858,-34.7921676686403));
#27475=CARTESIAN_POINT('Ctrl Pts',(-2.46826886854475,3.25497677296979,-34.7979732296592));
#27476=CARTESIAN_POINT('Ctrl Pts',(-2.37302092908558,3.32720387016827,-34.8037806843654));
#27477=CARTESIAN_POINT('Ctrl Pts',(-2.27463761115528,3.39521830701507,-34.8095881390717));
#27478=CARTESIAN_POINT('Ctrl Pts',(-2.17353411149157,3.45875331097529,-34.8153955937779));
#27479=CARTESIAN_POINT('Ctrl Pts',(-2.07231917105122,3.52235834604432,-34.8212094497191));
#27480=CARTESIAN_POINT('Ctrl Pts',(-1.96837840977851,3.58147387567573,-34.8270233056603));
#27481=CARTESIAN_POINT('Ctrl Pts',(-1.8621529840195,3.63587833461287,-34.8328371616016));
#27482=CARTESIAN_POINT('Ctrl Pts',(-1.75585767003262,3.69031858753432,-34.8386548426166));
#27483=CARTESIAN_POINT('Ctrl Pts',(-1.64727506808491,3.74004142740467,-34.8444725236316));
#27484=CARTESIAN_POINT('Ctrl Pts',(-1.53686621063264,3.78487347881216,-34.8502902046465));
#27485=CARTESIAN_POINT('Ctrl Pts',(-1.42630090424893,3.82976905706613,-34.8561161292934));
#27486=CARTESIAN_POINT('Ctrl Pts',(-1.31390456045862,3.86975987876471,-34.8619420539403));
#27487=CARTESIAN_POINT('Ctrl Pts',(-1.20015335692215,3.9047223870422,-34.8677679785872));
#27488=CARTESIAN_POINT('Ctrl Pts',(-1.17322243167338,3.91299986163286,-34.8691472830367));
#27489=CARTESIAN_POINT('Ctrl Pts',(-1.14621560689718,3.92099571550889,-34.8705265874861));
#27490=CARTESIAN_POINT('Ctrl Pts',(-1.11913927164857,3.92870873069688,-34.8719058919356));
#27491=CARTESIAN_POINT('Ctrl Pts',(-1.00477888093834,3.9612856441659,-34.8777315620014));
#27492=CARTESIAN_POINT('Ctrl Pts',(-0.888811943804751,3.98891717273778,
-34.8835572320672));
#27493=CARTESIAN_POINT('Ctrl Pts',(-0.771703712261843,4.01144592142052,
-34.889382902133));
#27494=CARTESIAN_POINT('Ctrl Pts',(-0.654743540980267,4.03394618694393,
-34.895201206788));
#27495=CARTESIAN_POINT('Ctrl Pts',(-0.536645342689016,4.05135642868629,
-34.901019511443));
#27496=CARTESIAN_POINT('Ctrl Pts',(-0.417889341804417,4.06356905909156,
-34.906837816098));
#27497=CARTESIAN_POINT('Ctrl Pts',(-0.299252591448985,4.07576942601013,
-34.9126502782196));
#27498=CARTESIAN_POINT('Ctrl Pts',(-0.179959756285397,4.08278252384552,
-34.9184627403411));
#27499=CARTESIAN_POINT('Ctrl Pts',(-0.060500474495871,4.084551957386,-34.9242752024627));
#27500=CARTESIAN_POINT('Ctrl Pts',(0.0588684033324125,4.08632005186098,
-34.9300832658503));
#27501=CARTESIAN_POINT('Ctrl Pts',(0.178403070480959,4.08285237366982,-34.9358913292378));
#27502=CARTESIAN_POINT('Ctrl Pts',(0.297610172620584,4.07414447278846,-34.9416993926254));
#27503=CARTESIAN_POINT('Ctrl Pts',(0.416769399934111,4.06544006909169,-34.9475051234337));
#27504=CARTESIAN_POINT('Ctrl Pts',(0.535600917600651,4.05149965774601,-34.9533108542419));
#27505=CARTESIAN_POINT('Ctrl Pts',(0.65361324170988,4.03237085723294,-34.9591165850501));
#27506=CARTESIAN_POINT('Ctrl Pts',(0.771605967742213,4.01324523340252,-34.964921351712));
#27507=CARTESIAN_POINT('Ctrl Pts',(0.888779368345493,3.98893300005499,-34.9707261183738));
#27508=CARTESIAN_POINT('Ctrl Pts',(1.00464957269879,3.959533335644,-34.9765308850356));
#27509=CARTESIAN_POINT('Ctrl Pts',(1.12052782646279,3.93013162886177,-34.9823360549499));
#27510=CARTESIAN_POINT('Ctrl Pts',(1.23510230882257,3.89564188957588,-34.9881412248643));
#27511=CARTESIAN_POINT('Ctrl Pts',(1.34790241018648,3.85621369903348,-34.9939463947786));
#27512=CARTESIAN_POINT('Ctrl Pts',(1.46079370495804,3.81675363271252,-34.9997562578911));
#27513=CARTESIAN_POINT('Ctrl Pts',(1.57190736800501,3.77234727584653,-35.0055661210036));
#27514=CARTESIAN_POINT('Ctrl Pts',(1.68079085356918,3.72319313312621,-35.011375984116));
#27515=CARTESIAN_POINT('Ctrl Pts',(1.78972161361045,3.6740176489106,-35.0171883697253));
#27516=CARTESIAN_POINT('Ctrl Pts',(1.89641990205823,3.62009045420047,-35.0230007553346));
#27517=CARTESIAN_POINT('Ctrl Pts',(2.00045733956525,3.56165627659092,-35.0288131409438));
#27518=CARTESIAN_POINT('Ctrl Pts',(2.10463072800272,3.50314574011473,-35.0346331218884));
#27519=CARTESIAN_POINT('Ctrl Pts',(2.20613597300339,3.44011667098013,-35.0404531028331));
#27520=CARTESIAN_POINT('Ctrl Pts',(2.30457302903138,3.37285756501236,-35.0462730837777));
#27521=CARTESIAN_POINT('Ctrl Pts',(2.36665186513484,3.33044094687771,-35.0499434255958));
#27522=CARTESIAN_POINT('Ctrl Pts',(2.42751106117837,3.28634283317704,-35.0536137674139));
#27523=CARTESIAN_POINT('Ctrl Pts',(2.4870572760686,3.24064362520074,-35.057284109232));
#27524=CARTESIAN_POINT('',(-4.08499921798789,-0.00252765470411389,-34.5103849714454));
#27525=CARTESIAN_POINT('Ctrl Pts',(-4.08499921798789,-0.00252765470410572,
-34.5103849714454));
#27526=CARTESIAN_POINT('Ctrl Pts',(-4.08507189103842,0.114920885278749,
-34.5161279682783));
#27527=CARTESIAN_POINT('Ctrl Pts',(-4.0800751941379,0.232562318317247,-34.5218709651111));
#27528=CARTESIAN_POINT('Ctrl Pts',(-4.0699856738512,0.349916582410724,-34.527613961944));
#27529=CARTESIAN_POINT('Ctrl Pts',(-4.05990723653758,0.467141937089886,
-34.5333506503025));
#27530=CARTESIAN_POINT('Ctrl Pts',(-4.04474713355492,0.584080334458861,
-34.5390873386611));
#27531=CARTESIAN_POINT('Ctrl Pts',(-4.02453394165429,0.700251063885355,
-34.5448240270196));
#27532=CARTESIAN_POINT('Ctrl Pts',(-4.00416272258904,0.817330018547843,
-34.5506055649299));
#27533=CARTESIAN_POINT('Ctrl Pts',(-3.97865904795262,0.933628817439481,
-34.5563871028402));
#27534=CARTESIAN_POINT('Ctrl Pts',(-3.94810563132553,1.04865958437217,-34.5621686407504));
#27535=CARTESIAN_POINT('Ctrl Pts',(-3.91782816729369,1.1626514154943,-34.5678979609199));
#27536=CARTESIAN_POINT('Ctrl Pts',(-3.88259192065302,1.27539761376406,-34.5736272810893));
#27537=CARTESIAN_POINT('Ctrl Pts',(-3.84252864447435,1.38643377641851,-34.5793566012588));
#27538=CARTESIAN_POINT('Ctrl Pts',(-3.80247324529,1.49744810782735,-34.5850847949646));
#27539=CARTESIAN_POINT('Ctrl Pts',(-3.75759284556215,1.60675267684264,-34.5908129886704));
#27540=CARTESIAN_POINT('Ctrl Pts',(-3.70806856918763,1.71389978884496,-34.5965411823763));
#27541=CARTESIAN_POINT('Ctrl Pts',(-3.65854159187046,1.82105274440979,-34.6022696884849));
#27542=CARTESIAN_POINT('Ctrl Pts',(-3.60437041159065,1.92604762802633,-34.6079981945936));
#27543=CARTESIAN_POINT('Ctrl Pts',(-3.5457833064289,2.02845895789146,-34.6137267007022));
#27544=CARTESIAN_POINT('Ctrl Pts',(-3.48624833339938,2.13252717810146,-34.6195478870492));
#27545=CARTESIAN_POINT('Ctrl Pts',(-3.42215350945476,2.233927120391,-34.6253690733962));
#27546=CARTESIAN_POINT('Ctrl Pts',(-3.35378495433835,2.33224172847792,-34.6311902597432));
#27547=CARTESIAN_POINT('Ctrl Pts',(-3.28641177720436,2.42912497391467,-34.6369266954221));
#27548=CARTESIAN_POINT('Ctrl Pts',(-3.2148887863614,2.52301182450451,-34.6426631311011));
#27549=CARTESIAN_POINT('Ctrl Pts',(-3.13953055420171,2.61353647367583,-34.64839956678));
#27550=CARTESIAN_POINT('Ctrl Pts',(-3.06250229707934,2.70606725302725,-34.654263128461));
#27551=CARTESIAN_POINT('Ctrl Pts',(-2.98146712601755,2.79508471007264,-34.6601266901421));
#27552=CARTESIAN_POINT('Ctrl Pts',(-2.89679987682826,2.88023878760213,-34.6659902518231));
#27553=CARTESIAN_POINT('Ctrl Pts',(-2.81213262763897,2.96539286513162,-34.6718538135041));
#27554=CARTESIAN_POINT('Ctrl Pts',(-2.72383368600946,3.04668330119613,-34.6777173751852));
#27555=CARTESIAN_POINT('Ctrl Pts',(-2.63231171170454,3.123805380049,-34.6835809368662));
#27556=CARTESIAN_POINT('Ctrl Pts',(-2.54138458930515,3.20042619987734,-34.6894063880184));
#27557=CARTESIAN_POINT('Ctrl Pts',(-2.44696383970992,3.27319626328287,-34.6952318391706));
#27558=CARTESIAN_POINT('Ctrl Pts',(-2.34940915475552,3.3417812052184,-34.7010572903228));
#27559=CARTESIAN_POINT('Ctrl Pts',(-2.25197691724743,3.4102800615805,-34.7068754295595));
#27560=CARTESIAN_POINT('Ctrl Pts',(-2.15141889928821,3.47460401221233,-34.7126935687962));
#27561=CARTESIAN_POINT('Ctrl Pts',(-2.04812888576518,3.53445795947473,-34.7185117080329));
#27562=CARTESIAN_POINT('Ctrl Pts',(-1.94494164963081,3.594252349843,-34.7243240580055));
#27563=CARTESIAN_POINT('Ctrl Pts',(-1.83902817706856,3.64958538199854,-34.7301364079782));
#27564=CARTESIAN_POINT('Ctrl Pts',(-1.7308118474824,3.70020477117342,-34.7359487579509));
#27565=CARTESIAN_POINT('Ctrl Pts',(-1.61894035730438,3.752533902281,-34.7419574283185));
#27566=CARTESIAN_POINT('Ctrl Pts',(-1.50460805523535,3.7998250786186,-34.7479660986861));
#27567=CARTESIAN_POINT('Ctrl Pts',(-1.3883115259683,3.84185060964941,-34.7539747690538));
#27568=CARTESIAN_POINT('Ctrl Pts',(-1.27594003603281,3.8824577676362,-34.7597806451706));
#27569=CARTESIAN_POINT('Ctrl Pts',(-1.16173518016177,3.91814882911819,-34.7655865212874));
#27570=CARTESIAN_POINT('Ctrl Pts',(-1.04616534780103,3.94876728423699,-34.7713923974042));
#27571=CARTESIAN_POINT('Ctrl Pts',(-0.930612261169279,3.97938130283164,
-34.7771974322667));
#27572=CARTESIAN_POINT('Ctrl Pts',(-0.813694985692373,4.00492407234662,
-34.7830024671291));
#27573=CARTESIAN_POINT('Ctrl Pts',(-0.695895948715241,4.02528928507775,
-34.7888075019916));
#27574=CARTESIAN_POINT('Ctrl Pts',(-0.578086233855809,4.04565634381161,
-34.7946130630509));
#27575=CARTESIAN_POINT('Ctrl Pts',(-0.459395000651461,4.06084484313215,
-34.8004186241101));
#27576=CARTESIAN_POINT('Ctrl Pts',(-0.340313083382252,4.07079992203975,
-34.8062241851694));
#27577=CARTESIAN_POINT('Ctrl Pts',(-0.221192323371624,4.08075824814529,
-34.8120316399159));
#27578=CARTESIAN_POINT('Ctrl Pts',(-0.101681032236312,4.08547972485986,
-34.8178390946624));
#27579=CARTESIAN_POINT('Ctrl Pts',(0.0177272842119958,4.08496153511811,
-34.8236465494089));
#27580=CARTESIAN_POINT('Ctrl Pts',(0.137267217815624,4.08444277420458,-34.8294604053903));
#27581=CARTESIAN_POINT('Ctrl Pts',(0.256703541938331,4.07867282065794,-34.8352742613716));
#27582=CARTESIAN_POINT('Ctrl Pts',(0.375545050646511,4.06770093725373,-34.8410881173529));
#27583=CARTESIAN_POINT('Ctrl Pts',(0.494464748001043,4.05672183518729,-34.846905798408));
#27584=CARTESIAN_POINT('Ctrl Pts',(0.612788447254424,4.0405340423935,-34.852723479463));
#27585=CARTESIAN_POINT('Ctrl Pts',(0.730033977028201,4.01923816069468,-34.858541160518));
#27586=CARTESIAN_POINT('Ctrl Pts',(0.84744564326344,3.997912102814,-34.8643670852046));
#27587=CARTESIAN_POINT('Ctrl Pts',(0.963775694404563,3.9714635997781,-34.8701930098911));
#27588=CARTESIAN_POINT('Ctrl Pts',(1.07855586087678,3.94004343313222,-34.8760189345777));
#27589=CARTESIAN_POINT('Ctrl Pts',(1.10573038831509,3.93260462025298,-34.8773982386431));
#27590=CARTESIAN_POINT('Ctrl Pts',(1.13281812654346,3.92488735000989,-34.8787775427086));
#27591=CARTESIAN_POINT('Ctrl Pts',(1.15981302825806,3.9168940168816,-34.880156846774));
#27592=CARTESIAN_POINT('Ctrl Pts',(1.27890982403516,3.88162882594951,-34.8862420956234));
#27593=CARTESIAN_POINT('Ctrl Pts',(1.39659581265874,3.84086790255425,-34.8923273444727));
#27594=CARTESIAN_POINT('Ctrl Pts',(1.51232740443447,3.79474515900561,-34.8984125933221));
#27595=CARTESIAN_POINT('Ctrl Pts',(1.62296374346671,3.75065303675922,-34.9042299301829));
#27596=CARTESIAN_POINT('Ctrl Pts',(1.73181365772583,3.70166130574987,-34.9100472670436));
#27597=CARTESIAN_POINT('Ctrl Pts',(1.83841493028788,3.64793853348636,-34.9158646039044));
#27598=CARTESIAN_POINT('Ctrl Pts',(1.94492283349963,3.5942628156362,-34.9216768455074));
#27599=CARTESIAN_POINT('Ctrl Pts',(2.04918564850979,3.53586447764656,-34.9274890871104));
#27600=CARTESIAN_POINT('Ctrl Pts',(2.15076070959423,3.47296031795149,-34.9333013287134));
#27601=CARTESIAN_POINT('Ctrl Pts',(2.25225919348319,3.41010358155189,-34.9391091884814));
#27602=CARTESIAN_POINT('Ctrl Pts',(2.35107361069731,3.34274799860495,-34.9449170482494));
#27603=CARTESIAN_POINT('Ctrl Pts',(2.44678622254801,3.27115609244641,-34.9507249080173));
#27604=CARTESIAN_POINT('Ctrl Pts',(2.46027181438137,3.2610690286169,-34.9515432163337));
#27605=CARTESIAN_POINT('Ctrl Pts',(2.47369587352053,3.25089793800677,-34.95236152465));
#27606=CARTESIAN_POINT('Ctrl Pts',(2.48705727606859,3.24064362520075,-34.9531798329663));
#27607=CARTESIAN_POINT('Ctrl Pts',(2.4870572760686,3.24064362520074,-33.7031235592767));
#27608=CARTESIAN_POINT('Ctrl Pts',(2.58140861963151,3.16823294921954,-33.7089479065311));
#27609=CARTESIAN_POINT('Ctrl Pts',(2.6727421027167,3.09158538855808,-33.7147722537854));
#27610=CARTESIAN_POINT('Ctrl Pts',(2.76065463340963,3.01098173276324,-33.7205966010398));
#27611=CARTESIAN_POINT('Ctrl Pts',(2.84845998739043,2.93047634321948,-33.7264138476637));
#27612=CARTESIAN_POINT('Ctrl Pts',(2.93285238629096,2.84602472527932,-33.7322310942876));
#27613=CARTESIAN_POINT('Ctrl Pts',(3.01345992186858,2.75794929237139,-33.7380483409115));
#27614=CARTESIAN_POINT('Ctrl Pts',(3.09399015369909,2.6699583250279,-33.7438600087151));
#27615=CARTESIAN_POINT('Ctrl Pts',(3.1707424694783,2.57835075612183,-33.7496716765187));
#27616=CARTESIAN_POINT('Ctrl Pts',(3.24338055930375,2.48348697349724,-33.7554833443222));
#27617=CARTESIAN_POINT('Ctrl Pts',(3.31722369002888,2.38704943338212,-33.7613914256936));
#27618=CARTESIAN_POINT('Ctrl Pts',(3.38681454731882,2.28724696092719,-33.7672995070649));
#27619=CARTESIAN_POINT('Ctrl Pts',(3.45184110457183,2.18449490472931,-33.7732075884363));
#27620=CARTESIAN_POINT('Ctrl Pts',(3.51574082737825,2.08352342190441,-33.7790132896436));
#27621=CARTESIAN_POINT('Ctrl Pts',(3.5752329498575,1.97970412336723,-33.7848189908508));
#27622=CARTESIAN_POINT('Ctrl Pts',(3.63006449254069,1.87346117653803,-33.7906246920581));
#27623=CARTESIAN_POINT('Ctrl Pts',(3.68488965641702,1.76723058944204,-33.7964297178613));
#27624=CARTESIAN_POINT('Ctrl Pts',(3.73505513173854,1.65857727733264,-33.8022347436645));
#27625=CARTESIAN_POINT('Ctrl Pts',(3.78035399916738,1.54794981862435,-33.8080397694677));
#27626=CARTESIAN_POINT('Ctrl Pts',(3.82565826654194,1.43730917233973,-33.813845487271));
#27627=CARTESIAN_POINT('Ctrl Pts',(3.86609461788279,1.32469428912235,-33.8196512050744));
#27628=CARTESIAN_POINT('Ctrl Pts',(3.90150460760563,1.21057292090646,-33.8254569228778));
#27629=CARTESIAN_POINT('Ctrl Pts',(3.93800825802992,1.09292683956332,-33.8314419540742));
#27630=CARTESIAN_POINT('Ctrl Pts',(3.96916987962091,0.973680146299653,-33.8374269852706));
#27631=CARTESIAN_POINT('Ctrl Pts',(3.99487195022529,0.85335988967327,-33.8434120164671));
#27632=CARTESIAN_POINT('Ctrl Pts',(4.01984107880477,0.736470787442399,-33.8492263734423));
#27633=CARTESIAN_POINT('Ctrl Pts',(4.0396578047206,0.618568938570236,-33.8550407304175));
#27634=CARTESIAN_POINT('Ctrl Pts',(4.0542669145193,0.500144764877267,-33.8608550873927));
#27635=CARTESIAN_POINT('Ctrl Pts',(4.06951927647338,0.376506269023205,-33.8669254556997));
#27636=CARTESIAN_POINT('Ctrl Pts',(4.07909491797284,0.252298906764303,-33.8729958240067));
#27637=CARTESIAN_POINT('Ctrl Pts',(4.08299155861645,0.128081740567421,-33.8790661923138));
#27638=CARTESIAN_POINT('Ctrl Pts',(4.08688819926007,0.00386457437053903,
-33.8851365606208));
#27639=CARTESIAN_POINT('Ctrl Pts',(4.08510591468131,-0.120361897969216,
-33.8912069289278));
#27640=CARTESIAN_POINT('Ctrl Pts',(4.07770364345426,-0.244045069935603,
-33.8972772972349));
#27641=CARTESIAN_POINT('Ctrl Pts',(4.0706000268172,-0.362738077953689,-33.9031027483669));
#27642=CARTESIAN_POINT('Ctrl Pts',(4.05829840808877,-0.481310545933248,
-33.9089281994989));
#27643=CARTESIAN_POINT('Ctrl Pts',(4.04080422479748,-0.59927140500681,-33.9147536506308));
#27644=CARTESIAN_POINT('Ctrl Pts',(4.02333199963246,-0.717084203471046,
-33.9205717898473));
#27645=CARTESIAN_POINT('Ctrl Pts',(4.0006802327364,-0.834286519845738,-33.9263899290637));
#27646=CARTESIAN_POINT('Ctrl Pts',(3.97290631151279,-0.950389625333658,
-33.9322080682801));
#27647=CARTESIAN_POINT('Ctrl Pts',(3.94516002636953,-1.06637720393122,-33.9380204182324));
#27648=CARTESIAN_POINT('Ctrl Pts',(3.91230182081931,-1.18126735300376,-33.9438327681848));
#27649=CARTESIAN_POINT('Ctrl Pts',(3.8744405029074,-1.29457938707159,-33.9496451181372));
#27650=CARTESIAN_POINT('Ctrl Pts',(3.83530036489639,-1.41171869696148,-33.9556537885124));
#27651=CARTESIAN_POINT('Ctrl Pts',(3.79081322265837,-1.52717095930536,-33.9616624588877));
#27652=CARTESIAN_POINT('Ctrl Pts',(3.74115614356725,-1.64041936999324,-33.9676711292629));
#27653=CARTESIAN_POINT('Ctrl Pts',(3.69317500455989,-1.74984561565717,-33.9734770053595));
#27654=CARTESIAN_POINT('Ctrl Pts',(3.6403674480488,-1.85721396695235,-33.9792828814561));
#27655=CARTESIAN_POINT('Ctrl Pts',(3.58294271170609,-1.96207709446703,-33.9850887575528));
#27656=CARTESIAN_POINT('Ctrl Pts',(3.52552629603823,-2.06692502762399,-33.9908937923951));
#27657=CARTESIAN_POINT('Ctrl Pts',(3.46349422697335,-2.16926810114257,-33.9966988272374));
#27658=CARTESIAN_POINT('Ctrl Pts',(3.39710180162501,-2.26868339558346,-34.0025038620797));
#27659=CARTESIAN_POINT('Ctrl Pts',(3.33070335814077,-2.36810770151549,-34.0083094231189));
#27660=CARTESIAN_POINT('Ctrl Pts',(3.25994399914227,-2.46460336139142,-34.0141149841581));
#27661=CARTESIAN_POINT('Ctrl Pts',(3.18512210400834,-2.5577768046797,-34.0199205451973));
#27662=CARTESIAN_POINT('Ctrl Pts',(3.11027580308902,-2.65098063975445,-34.0257279999239));
#27663=CARTESIAN_POINT('Ctrl Pts',(3.03136458594073,-2.74085978509838,-34.0315354546505));
#27664=CARTESIAN_POINT('Ctrl Pts',(2.94872639587784,-2.82705458777387,-34.037342909377));
#27665=CARTESIAN_POINT('Ctrl Pts',(2.86599711832371,-2.91334439819732,-34.0431567653387));
#27666=CARTESIAN_POINT('Ctrl Pts',(2.77953295055453,-2.99594146523343,-34.0489706213003));
#27667=CARTESIAN_POINT('Ctrl Pts',(2.68970800095107,-3.07452368174646,-34.054784477262));
#27668=CARTESIAN_POINT('Ctrl Pts',(2.59982395338143,-3.15315759936475,-34.0606021582975));
#27669=CARTESIAN_POINT('Ctrl Pts',(2.50657503821053,-3.22777115151494,-34.0664198393329));
#27670=CARTESIAN_POINT('Ctrl Pts',(2.41036635228617,-3.29808414807243,-34.0722375203684));
#27671=CARTESIAN_POINT('Ctrl Pts',(2.31402133902063,-3.368496777878,-34.0780634450357));
#27672=CARTESIAN_POINT('Ctrl Pts',(2.21470852277989,-3.43459646429006,-34.0838893697031));
#27673=CARTESIAN_POINT('Ctrl Pts',(2.11285979541865,-3.49614766348669,-34.0897152943704));
#27674=CARTESIAN_POINT('Ctrl Pts',(2.08874681914687,-3.51072008519663,-34.0910945986278));
#27675=CARTESIAN_POINT('Ctrl Pts',(2.06449179678867,-3.5250377642382,-34.0924739028853));
#27676=CARTESIAN_POINT('Ctrl Pts',(2.04010063005674,-3.5390979668896,-34.0938532071427));
#27677=CARTESIAN_POINT('Ctrl Pts',(1.93708525171181,-3.59848082100475,-34.0996786582781));
#27678=CARTESIAN_POINT('Ctrl Pts',(1.83131017195687,-3.65345711139818,-34.1055041094136));
#27679=CARTESIAN_POINT('Ctrl Pts',(1.72318841613334,-3.70376115354431,-34.111329560549));
#27680=CARTESIAN_POINT('Ctrl Pts',(1.61520237119852,-3.75400205570337,-34.1171476997689));
#27681=CARTESIAN_POINT('Ctrl Pts',(1.50487587551227,-3.79958220349568,-34.1229658389887));
#27682=CARTESIAN_POINT('Ctrl Pts',(1.39264858741361,-3.84028057724626,-34.1287839782086));
#27683=CARTESIAN_POINT('Ctrl Pts',(1.28053296962322,-3.8809384546076,-34.1345963281644));
#27684=CARTESIAN_POINT('Ctrl Pts',(1.16652070352613,-3.91672408330216,-34.1404086781203));
#27685=CARTESIAN_POINT('Ctrl Pts',(1.05107302712988,-3.94746380498163,-34.1462210280761));
#27686=CARTESIAN_POINT('Ctrl Pts',(0.931725940637991,-3.97924180464811,
-34.15222969845));
#27687=CARTESIAN_POINT('Ctrl Pts',(0.81084516407094,-4.00562681086514,-34.158238368824));
#27688=CARTESIAN_POINT('Ctrl Pts',(0.68895965546336,-4.0264822852142,-34.1642470391979));
#27689=CARTESIAN_POINT('Ctrl Pts',(0.571187816215797,-4.0466338815814,-34.170052915298));
#27690=CARTESIAN_POINT('Ctrl Pts',(0.452478404756792,-4.06162309540167,
-34.1758587913981));
#27691=CARTESIAN_POINT('Ctrl Pts',(0.333320071698919,-4.07137848029419,
-34.1816646674982));
#27692=CARTESIAN_POINT('Ctrl Pts',(0.214179004332095,-4.0811324516602,-34.1874697023439));
#27693=CARTESIAN_POINT('Ctrl Pts',(0.0945895512791576,-4.08565406902207,
-34.1932747371897));
#27694=CARTESIAN_POINT('Ctrl Pts',(-0.0249546731795135,-4.08492377704732,
-34.1990797720354));
#27695=CARTESIAN_POINT('Ctrl Pts',(-0.144509733714166,-4.08419341887531,
-34.204885333078));
#27696=CARTESIAN_POINT('Ctrl Pts',(-0.264019149476858,-4.07821020733982,
-34.2106908941207));
#27697=CARTESIAN_POINT('Ctrl Pts',(-0.382990104713468,-4.06700671006227,
-34.2164964551633));
#27698=CARTESIAN_POINT('Ctrl Pts',(-0.501999866499577,-4.05579955837118,
-34.2223039098933));
#27699=CARTESIAN_POINT('Ctrl Pts',(-0.620470412446873,-4.03936877268701,
-34.2281113646233));
#27700=CARTESIAN_POINT('Ctrl Pts',(-0.737915476155763,-4.01779861989745,
-34.2339188193533));
#27701=CARTESIAN_POINT('Ctrl Pts',(-0.855489993040401,-3.99620469152556,
-34.2397326753183));
#27702=CARTESIAN_POINT('Ctrl Pts',(-0.972036369967927,-3.96946016251569,
-34.2455465312833));
#27703=CARTESIAN_POINT('Ctrl Pts',(-1.08707978970347,-3.93770015755622,
-34.2513603872483));
#27704=CARTESIAN_POINT('Ctrl Pts',(-1.20219889923479,-3.90591925693584,
-34.2571780682872));
#27705=CARTESIAN_POINT('Ctrl Pts',(-1.31581269501042,-3.86911643407099,
-34.262995749326));
#27706=CARTESIAN_POINT('Ctrl Pts',(-1.4274643074096,-3.82747575447208,-34.2688134303648));
#27707=CARTESIAN_POINT('Ctrl Pts',(-1.5392741297167,-3.78577607018938,-34.2746393550354));
#27708=CARTESIAN_POINT('Ctrl Pts',(-1.64911584502968,-3.73922500567654,
-34.280465279706));
#27709=CARTESIAN_POINT('Ctrl Pts',(-1.75655511782045,-3.68805356767751,
-34.2862912043767));
#27710=CARTESIAN_POINT('Ctrl Pts',(-1.78199167102502,-3.67593858428822,
-34.2876705086013));
#27711=CARTESIAN_POINT('Ctrl Pts',(-1.80729368388432,-3.66356481564983,
-34.2890498128259));
#27712=CARTESIAN_POINT('Ctrl Pts',(-1.83245562620588,-3.65093568527116,
-34.2904291170505));
#27713=CARTESIAN_POINT('Ctrl Pts',(-1.93872635511457,-3.59759692176587,
-34.2962545681808));
#27714=CARTESIAN_POINT('Ctrl Pts',(-2.04283629197228,-3.53952902162373,
-34.302080019311));
#27715=CARTESIAN_POINT('Ctrl Pts',(-2.14433631617764,-3.47693065261902,
-34.3079054704413));
#27716=CARTESIAN_POINT('Ctrl Pts',(-2.24570894087504,-3.41441085503803,
-34.313723609656));
#27717=CARTESIAN_POINT('Ctrl Pts',(-2.3444778244325,-3.34737211145425,-34.3195417488707));
#27718=CARTESIAN_POINT('Ctrl Pts',(-2.44021648497874,-3.27605990580728,
-34.3253598880854));
#27719=CARTESIAN_POINT('Ctrl Pts',(-2.53585988201199,-3.20481865844602,
-34.3311722380361));
#27720=CARTESIAN_POINT('Ctrl Pts',(-2.62847872912805,-3.12931265088252,
-34.3369845879868));
#27721=CARTESIAN_POINT('Ctrl Pts',(-2.71767421543167,-3.04983144760131,
-34.3427969379375));
#27722=CARTESIAN_POINT('Ctrl Pts',(-2.8098824067416,-2.96766565310414,-34.3488056083133));
#27723=CARTESIAN_POINT('Ctrl Pts',(-2.89843150791676,-2.88125160684509,
-34.3548142786892));
#27724=CARTESIAN_POINT('Ctrl Pts',(-2.9829164376061,-2.79095584455565,-34.3608229490651));
#27725=CARTESIAN_POINT('Ctrl Pts',(-3.06454997763867,-2.7037075891244,-34.3666288251601));
#27726=CARTESIAN_POINT('Ctrl Pts',(-3.14238895228346,-2.61283572932098,
-34.3724347012551));
#27727=CARTESIAN_POINT('Ctrl Pts',(-3.21610481112445,-2.51870896370782,
-34.3782405773501));
#27728=CARTESIAN_POINT('Ctrl Pts',(-3.28980998875537,-2.42459583678481,
-34.3840456121908));
#27729=CARTESIAN_POINT('Ctrl Pts',(-3.35939298721425,-2.32722906314811,
-34.3898506470315));
#27730=CARTESIAN_POINT('Ctrl Pts',(-3.42456585272475,-2.22701004046942,
-34.3956556818722));
#27731=CARTESIAN_POINT('Ctrl Pts',(-3.48974462582455,-2.12678193344525,
-34.4014612429098));
#27732=CARTESIAN_POINT('Ctrl Pts',(-3.55051224871766,-2.0237014054016,-34.4072668039475));
#27733=CARTESIAN_POINT('Ctrl Pts',(-3.60662472871704,-1.9181978694094,-34.4130723649851));
#27734=CARTESIAN_POINT('Ctrl Pts',(-3.6627555117701,-1.81265991973804,-34.4188798197101));
#27735=CARTESIAN_POINT('Ctrl Pts',(-3.71422794057079,-1.70469775031853,
-34.4246872744352));
#27736=CARTESIAN_POINT('Ctrl Pts',(-3.76084479430878,-1.59476375464222,
-34.4304947291602));
#27737=CARTESIAN_POINT('Ctrl Pts',(-3.80751303121828,-1.48470858482176,
-34.4363085851204));
#27738=CARTESIAN_POINT('Ctrl Pts',(-3.84931485079231,-1.37267762631494,
-34.4421224410805));
#27739=CARTESIAN_POINT('Ctrl Pts',(-3.88610179775092,-1.25914169874445,
-34.4479362970407));
#27740=CARTESIAN_POINT('Ctrl Pts',(-3.92291294771529,-1.14553107319179,
-34.4537539780747));
#27741=CARTESIAN_POINT('Ctrl Pts',(-3.95470254576335,-1.03041389900235,
-34.4595716591087));
#27742=CARTESIAN_POINT('Ctrl Pts',(-3.98137287746323,-0.914272940975595,
-34.4653893401428));
#27743=CARTESIAN_POINT('Ctrl Pts',(-4.00808100092164,-0.797967411653265,
-34.4712152648087));
#27744=CARTESIAN_POINT('Ctrl Pts',(-4.02965530652827,-0.680635602909504,
-34.4770411894746));
#27745=CARTESIAN_POINT('Ctrl Pts',(-4.04604967492253,-0.562767294766934,
-34.4828671141405));
#27746=CARTESIAN_POINT('Ctrl Pts',(-4.04993108837527,-0.534861636807215,
-34.4842464184131));
#27747=CARTESIAN_POINT('Ctrl Pts',(-4.05352238634429,-0.506925913458926,
-34.4856257226857));
#27748=CARTESIAN_POINT('Ctrl Pts',(-4.05682338424715,-0.478966626212638,
-34.4870050269583));
#27749=CARTESIAN_POINT('Ctrl Pts',(-4.07547461035645,-0.320991673294925,
-34.4947983417737));
#27750=CARTESIAN_POINT('Ctrl Pts',(-4.08490059976322,-0.161906717262808,
-34.5025916565891));
#27751=CARTESIAN_POINT('Ctrl Pts',(-4.08499921798737,-0.00252765554147077,
-34.5103849714045));
#27752=CARTESIAN_POINT('Origin',(0.,0.,-25.2396150285955));
#27753=CARTESIAN_POINT('',(2.48705727606859,3.24064362520075,-32.4530286559313));
#27754=CARTESIAN_POINT('',(2.48705727606861,3.24064362520074,-32.5574517732253));
#27755=CARTESIAN_POINT('',(2.4870572760686,3.24064362520075,-25.2396150285955));
#27756=CARTESIAN_POINT('',(-4.08393919123128,-0.00301203127919971,-33.3646149993214));
#27757=CARTESIAN_POINT('Ctrl Pts',(2.48705727606861,3.24064362520074,-32.5574517732253));
#27758=CARTESIAN_POINT('Ctrl Pts',(2.58172320530517,3.16799151798577,-32.5632616020185));
#27759=CARTESIAN_POINT('Ctrl Pts',(2.67328514414928,3.09112485577708,-32.5690714308118));
#27760=CARTESIAN_POINT('Ctrl Pts',(2.76135115698028,3.01034296847447,-32.5748812596051));
#27761=CARTESIAN_POINT('Ctrl Pts',(2.84937101736654,2.92960341625062,-32.5806880436619));
#27762=CARTESIAN_POINT('Ctrl Pts',(2.9338982955662,2.84495299497576,-32.5864948277187));
#27763=CARTESIAN_POINT('Ctrl Pts',(3.01457442907343,2.75673103722082,-32.5923016117755));
#27764=CARTESIAN_POINT('Ctrl Pts',(3.09522959340846,2.66853200993298,-32.5981068865451));
#27765=CARTESIAN_POINT('Ctrl Pts',(3.17203532837339,2.57676359299807,-32.6039121613148));
#27766=CARTESIAN_POINT('Ctrl Pts',(3.24467064842198,2.48180123766366,-32.6097174360844));
#27767=CARTESIAN_POINT('Ctrl Pts',(3.31730419799415,2.38684119702424,-32.6155225693512));
#27768=CARTESIAN_POINT('Ctrl Pts',(3.38576728708351,2.28868769701797,-32.621327702618));
#27769=CARTESIAN_POINT('Ctrl Pts',(3.4497802746404,2.18774794176615,-32.6271328358848));
#27770=CARTESIAN_POINT('Ctrl Pts',(3.51380677956652,2.08678687146571,-32.6329391949986));
#27771=CARTESIAN_POINT('Ctrl Pts',(3.57338109574889,1.98303872041235,-32.6387455541124));
#27772=CARTESIAN_POINT('Ctrl Pts',(3.62826817427027,1.87693768025938,-32.6445519132262));
#27773=CARTESIAN_POINT('Ctrl Pts',(3.68321269754718,1.77072559487543,-32.650364349269));
#27774=CARTESIAN_POINT('Ctrl Pts',(3.73345999844513,1.66215606547514,-32.6561767853119));
#27775=CARTESIAN_POINT('Ctrl Pts',(3.77882198208528,1.55168599520299,-32.6619892213547));
#27776=CARTESIAN_POINT('Ctrl Pts',(3.82420913072869,1.44115464058092,-32.6678048819032));
#27777=CARTESIAN_POINT('Ctrl Pts',(3.86470542475532,1.32872102830188,-32.6736205424516));
#27778=CARTESIAN_POINT('Ctrl Pts',(3.90017230377922,1.21485842830903,-32.6794362030001));
#27779=CARTESIAN_POINT('Ctrl Pts',(3.93569417491232,1.10081928206499,-32.6852608808472));
#27780=CARTESIAN_POINT('Ctrl Pts',(3.9661709492188,0.985347116488283,-32.6910855586943));
#27781=CARTESIAN_POINT('Ctrl Pts',(3.99151484202714,0.868927077421931,-32.6969102365414));
#27782=CARTESIAN_POINT('Ctrl Pts',(4.00987752083801,0.784576034719471,-32.7011304520108));
#27783=CARTESIAN_POINT('Ctrl Pts',(4.02554672280569,0.699727619360669,-32.7053506674801));
#27784=CARTESIAN_POINT('Ctrl Pts',(4.03850610398736,0.614567692005377,-32.7095708829494));
#27785=CARTESIAN_POINT('Ctrl Pts',(4.05639482136825,0.497015638301612,-32.7153963340847));
#27786=CARTESIAN_POINT('Ctrl Pts',(4.06917537424636,0.378493836629278,-32.72122178522));
#27787=CARTESIAN_POINT('Ctrl Pts',(4.07675032949716,0.259483623654406,-32.7270472363553));
#27788=CARTESIAN_POINT('Ctrl Pts',(4.08431577691211,0.140622788402665,-32.7328653755751));
#27789=CARTESIAN_POINT('Ctrl Pts',(4.08668859704055,0.0212751648462426,
-32.7386835147948));
#27790=CARTESIAN_POINT('Ctrl Pts',(4.08382264634036,-0.0980693287305154,
-32.7445016540146));
#27791=CARTESIAN_POINT('Ctrl Pts',(4.08095954736724,-0.217295070116563,
-32.7503140039703));
#27792=CARTESIAN_POINT('Ctrl Pts',(4.07286805768413,-0.336517282128182,
-32.7561263539261));
#27793=CARTESIAN_POINT('Ctrl Pts',(4.0595539991492,-0.455243152602845,-32.7619387038819));
#27794=CARTESIAN_POINT('Ctrl Pts',(4.04579023927839,-0.57797915886101,-32.7679473742558));
#27795=CARTESIAN_POINT('Ctrl Pts',(4.02644483800421,-0.700184257555691,
-32.7739560446298));
#27796=CARTESIAN_POINT('Ctrl Pts',(4.00158280818318,-0.821316034941986,
-32.7799647150038));
#27797=CARTESIAN_POINT('Ctrl Pts',(3.97755987869073,-0.938359581602993,
-32.7857705911039));
#27798=CARTESIAN_POINT('Ctrl Pts',(3.9483867759184,-1.05440065611912,-32.7915764672039));
#27799=CARTESIAN_POINT('Ctrl Pts',(3.91417450767327,-1.16895805035113,-32.797382343304));
#27800=CARTESIAN_POINT('Ctrl Pts',(3.87996719668473,-1.28349884555519,-32.8031873781498));
#27801=CARTESIAN_POINT('Ctrl Pts',(3.84072228906231,-1.39655599716866,-32.8089924129956));
#27802=CARTESIAN_POINT('Ctrl Pts',(3.79660094001163,-1.50766252931577,-32.8147974478414));
#27803=CARTESIAN_POINT('Ctrl Pts',(3.7524755915848,-1.61877913270556,-32.8206030088841));
#27804=CARTESIAN_POINT('Ctrl Pts',(3.70347307347273,-1.72794438585373,-32.8264085699268));
#27805=CARTESIAN_POINT('Ctrl Pts',(3.6498028104171,-1.8347109976973,-32.8322141309695));
#27806=CARTESIAN_POINT('Ctrl Pts',(3.59611504092265,-1.94151243521623,-32.8380215856996));
#27807=CARTESIAN_POINT('Ctrl Pts',(3.53775668159944,-2.04591331103718,-32.8438290404296));
#27808=CARTESIAN_POINT('Ctrl Pts',(3.47498294221769,-2.14749122263541,-32.8496364951597));
#27809=CARTESIAN_POINT('Ctrl Pts',(3.4121400108264,-2.2491810979289,-32.8554503511249));
#27810=CARTESIAN_POINT('Ctrl Pts',(3.34487219957761,-2.34804145083341,-32.86126420709));
#27811=CARTESIAN_POINT('Ctrl Pts',(3.27347793879498,-2.44367902643177,-32.8670780630552));
#27812=CARTESIAN_POINT('Ctrl Pts',(3.20203670603364,-2.53937952426109,-32.8728957440942));
#27813=CARTESIAN_POINT('Ctrl Pts',(3.12646387447464,-2.63185270681192,-32.8787134251331));
#27814=CARTESIAN_POINT('Ctrl Pts',(3.04709694760438,-2.72073982436765,-32.8845311061721));
#27815=CARTESIAN_POINT('Ctrl Pts',(2.96761755810181,-2.80975289462953,-32.8903570308429));
#27816=CARTESIAN_POINT('Ctrl Pts',(2.88433362686235,-2.89516946694921,-32.8961829555137));
#27817=CARTESIAN_POINT('Ctrl Pts',(2.79761820097002,-2.97666884311998,-32.9020088801845));
#27818=CARTESIAN_POINT('Ctrl Pts',(2.7770880774276,-2.99596405206578,-32.9033881844088));
#27819=CARTESIAN_POINT('Ctrl Pts',(2.75636575017673,-3.01503987859658,-32.904767488633));
#27820=CARTESIAN_POINT('Ctrl Pts',(2.73545641829513,-3.03389241463965,-32.9061467928573));
#27821=CARTESIAN_POINT('Ctrl Pts',(2.64714646539456,-3.11351555034991,-32.9119722439893));
#27822=CARTESIAN_POINT('Ctrl Pts',(2.5552158770103,-3.18940709734534,-32.9177976951212));
#27823=CARTESIAN_POINT('Ctrl Pts',(2.46001294474537,-3.26122083148094,-32.9236231462532));
#27824=CARTESIAN_POINT('Ctrl Pts',(2.36492950808498,-3.33294442736795,-32.9294412854696));
#27825=CARTESIAN_POINT('Ctrl Pts',(2.26658222001921,-3.40060014728236,-32.935259424686));
#27826=CARTESIAN_POINT('Ctrl Pts',(2.16535476120644,-3.46387987062493,-32.9410775639024));
#27827=CARTESIAN_POINT('Ctrl Pts',(2.06422802746459,-3.52709662829894,-32.9468899138548));
#27828=CARTESIAN_POINT('Ctrl Pts',(1.96022716842146,-3.58594583682477,-32.9527022638071));
#27829=CARTESIAN_POINT('Ctrl Pts',(1.85376687652398,-3.6401611732865,-32.9585146137595));
#27830=CARTESIAN_POINT('Ctrl Pts',(1.74371073618401,-3.69620771018643,-32.9645232841347));
#27831=CARTESIAN_POINT('Ctrl Pts',(1.63102643496968,-3.74730153529941,-32.97053195451));
#27832=CARTESIAN_POINT('Ctrl Pts',(1.5162026532571,-3.79319845437279,-32.9765406248852));
#27833=CARTESIAN_POINT('Ctrl Pts',(1.40525420577434,-3.83754633979761,-32.9823465009818));
#27834=CARTESIAN_POINT('Ctrl Pts',(1.2923087726332,-3.87704228917243,-32.9881523770784));
#27835=CARTESIAN_POINT('Ctrl Pts',(1.17782923873314,-3.91151419329974,-32.9939582531751));
#27836=CARTESIAN_POINT('Ctrl Pts',(1.0633662925797,-3.94598110254987,-32.9997632880174));
#27837=CARTESIAN_POINT('Ctrl Pts',(0.947370078327658,-3.97542529669491,
-33.0055683228597));
#27838=CARTESIAN_POINT('Ctrl Pts',(0.830319192253988,-3.99972437037537,
-33.011373357702));
#27839=CARTESIAN_POINT('Ctrl Pts',(0.713257696112499,-4.02402564664335,
-33.0171789187412));
#27840=CARTESIAN_POINT('Ctrl Pts',(0.595141737588523,-4.04318079223594,
-33.0229844797804));
#27841=CARTESIAN_POINT('Ctrl Pts',(0.4764600382136,-4.05711853807422,-33.0287900408196));
#27842=CARTESIAN_POINT('Ctrl Pts',(0.357739626639744,-4.07106083019716,
-33.0345974955461));
#27843=CARTESIAN_POINT('Ctrl Pts',(0.238453512227109,-4.07978229038899,
-33.0404049502727));
#27844=CARTESIAN_POINT('Ctrl Pts',(0.119094829578062,-4.0832635748342,-33.0462124049992));
#27845=CARTESIAN_POINT('Ctrl Pts',(-0.00039541552347408,-4.08674869650607,
-33.0520262609609));
#27846=CARTESIAN_POINT('Ctrl Pts',(-0.119957980454486,-4.08498210146,-33.0578401169225));
#27847=CARTESIAN_POINT('Ctrl Pts',(-0.239100284959963,-4.07799657353118,
-33.0636539728842));
#27848=CARTESIAN_POINT('Ctrl Pts',(-0.358320976015313,-4.07100644965774,
-33.0694716539196));
#27849=CARTESIAN_POINT('Ctrl Pts',(-0.47712045105476,-4.05879059621428,
-33.0752893349551));
#27850=CARTESIAN_POINT('Ctrl Pts',(-0.595013439880053,-4.04143340986365,
-33.0811070159906));
#27851=CARTESIAN_POINT('Ctrl Pts',(-0.713073482620973,-4.02405162844614,
-33.0869329406579));
#27852=CARTESIAN_POINT('Ctrl Pts',(-0.830224076280858,-4.00151405052528,
-33.0927588653252));
#27853=CARTESIAN_POINT('Ctrl Pts',(-0.945992164063851,-3.97395568993035,
-33.0985847899925));
#27854=CARTESIAN_POINT('Ctrl Pts',(-0.973400588560486,-3.96743116957174,
-33.09996409425));
#27855=CARTESIAN_POINT('Ctrl Pts',(-1.00073159851543,-3.96062544127137,
-33.1013433985076));
#27856=CARTESIAN_POINT('Ctrl Pts',(-1.02797906981974,-3.95354069563126,
-33.1027227027651));
#27857=CARTESIAN_POINT('Ctrl Pts',(-1.14305796681636,-3.92361847992695,
-33.1085481538981));
#27858=CARTESIAN_POINT('Ctrl Pts',(-1.25701341679574,-3.88861968836278,
-33.1143736050311));
#27859=CARTESIAN_POINT('Ctrl Pts',(-1.36936467170234,-3.84864461803029,
-33.1201990561641));
#27860=CARTESIAN_POINT('Ctrl Pts',(-1.4815749069912,-3.80871972309764,-33.1260171953815));
#27861=CARTESIAN_POINT('Ctrl Pts',(-1.59218457109093,-3.76383110851015,
-33.1318353345989));
#27862=CARTESIAN_POINT('Ctrl Pts',(-1.70072525783867,-3.71412958812015,
-33.1376534738164));
#27863=CARTESIAN_POINT('Ctrl Pts',(-1.80915794258291,-3.66447752258382,
-33.1434658237698));
#27864=CARTESIAN_POINT('Ctrl Pts',(-1.91552537673333,-3.61002224751509,
-33.1492781737232));
#27865=CARTESIAN_POINT('Ctrl Pts',(-2.01937698927143,-3.55096347139774,
-33.1550905236766));
#27866=CARTESIAN_POINT('Ctrl Pts',(-2.1267363383542,-3.48990990076341,-33.1610991940514));
#27867=CARTESIAN_POINT('Ctrl Pts',(-2.23140648815104,-3.42393649366664,
-33.1671078644263));
#27868=CARTESIAN_POINT('Ctrl Pts',(-2.33291463067306,-3.35331691404072,
-33.1731165348011));
#27869=CARTESIAN_POINT('Ctrl Pts',(-2.43099684547556,-3.28508076464384,
-33.1789224108987));
#27870=CARTESIAN_POINT('Ctrl Pts',(-2.5261266845148,-3.21250725285454,-33.1847282869964));
#27871=CARTESIAN_POINT('Ctrl Pts',(-2.61790572415689,-3.1358881707463,-33.190534163094));
#27872=CARTESIAN_POINT('Ctrl Pts',(-2.70967146528695,-3.05928019051699,
-33.1963391979373));
#27873=CARTESIAN_POINT('Ctrl Pts',(-2.79808705946827,-2.9786280671734,-33.2021442327806));
#27874=CARTESIAN_POINT('Ctrl Pts',(-2.88278693919141,-2.89426406245654,
-33.2079492676239));
#27875=CARTESIAN_POINT('Ctrl Pts',(-2.96749449652806,-2.80989241057152,
-33.2137548286642));
#27876=CARTESIAN_POINT('Ctrl Pts',(-3.04848538064976,-2.7218084962934,-33.2195603897044));
#27877=CARTESIAN_POINT('Ctrl Pts',(-3.12543115015846,-2.6303811749667,-33.2253659507446));
#27878=CARTESIAN_POINT('Ctrl Pts',(-3.20240201822857,-2.53892403141254,
-33.2311734054721));
#27879=CARTESIAN_POINT('Ctrl Pts',(-3.27532488496593,-2.44412162389534,
-33.2369808601997));
#27880=CARTESIAN_POINT('Ctrl Pts',(-3.34391223716288,-2.34637506595863,
-33.2427883149273));
#27881=CARTESIAN_POINT('Ctrl Pts',(-3.41257518939194,-2.24852076741549,
-33.2486021708899));
#27882=CARTESIAN_POINT('Ctrl Pts',(-3.47689285389555,-2.14771617511677,
-33.2544160268525));
#27883=CARTESIAN_POINT('Ctrl Pts',(-3.53662154811065,-2.04439062447456,
-33.2602298828152));
#27884=CARTESIAN_POINT('Ctrl Pts',(-3.59638953925116,-1.94099709350043,
-33.2660475638516));
#27885=CARTESIAN_POINT('Ctrl Pts',(-3.65156235915723,-1.83507966201013,
-33.271865244888));
#27886=CARTESIAN_POINT('Ctrl Pts',(-3.70194344356619,-1.72708996309899,
-33.2776829259245));
#27887=CARTESIAN_POINT('Ctrl Pts',(-3.75239591777952,-1.61894724319656,
-33.2835088505928));
#27888=CARTESIAN_POINT('Ctrl Pts',(-3.79804294926478,-1.5087267708014,-33.289334775261));
#27889=CARTESIAN_POINT('Ctrl Pts',(-3.83873695890835,-1.39689783460032,
-33.2951606999293));
#27890=CARTESIAN_POINT('Ctrl Pts',(-3.84837138152122,-1.37042201564943,
-33.2965400041772));
#27891=CARTESIAN_POINT('Ctrl Pts',(-3.85772840126692,-1.34385609362042,
-33.2979193084251));
#27892=CARTESIAN_POINT('Ctrl Pts',(-3.86680647728966,-1.31720638746962,
-33.2992986126729));
#27893=CARTESIAN_POINT('Ctrl Pts',(-3.91171149104778,-1.18538270386582,
-33.306121388344));
#27894=CARTESIAN_POINT('Ctrl Pts',(-3.94990424892378,-1.05116500701228,
-33.3129441640151));
#27895=CARTESIAN_POINT('Ctrl Pts',(-3.98116232529437,-0.91518934634136,
-33.3197669396861));
#27896=CARTESIAN_POINT('Ctrl Pts',(-4.01227614441052,-0.779841218703709,
-33.3265582279785));
#27897=CARTESIAN_POINT('Ctrl Pts',(-4.03651905423974,-0.642751411539236,
-33.333349516271));
#27898=CARTESIAN_POINT('Ctrl Pts',(-4.05371878773402,-0.504568122231469,
-33.3401408045634));
#27899=CARTESIAN_POINT('Ctrl Pts',(-4.0707767280463,-0.367524004545033,
-33.3468761060362));
#27900=CARTESIAN_POINT('Ctrl Pts',(-4.08090705786169,-0.229404471212952,
-33.353611407509));
#27901=CARTESIAN_POINT('Ctrl Pts',(-4.08398938536452,-0.0908608839378785,
-33.3603467089818));
#27902=CARTESIAN_POINT('Ctrl Pts',(-4.08464049359338,-0.0615950549015332,
-33.3617694683119));
#27903=CARTESIAN_POINT('Ctrl Pts',(-4.08497727930409,-0.0323103685043114,
-33.3631922276419));
#27904=CARTESIAN_POINT('Ctrl Pts',(-4.08499888879145,-0.00301306698060582,
-33.3646149869719));
#27905=CARTESIAN_POINT('Ctrl Pts',(-4.08142719209529,-0.00300957616263146,
-33.3646150285955));
#27906=CARTESIAN_POINT('Ctrl Pts',(-4.07512000112023,0.897168111157932,
-33.4083681932572));
#27907=CARTESIAN_POINT('Ctrl Pts',(-3.3405993134047,3.15482004326997,-33.5176466612216));
#27908=CARTESIAN_POINT('Ctrl Pts',(-0.208040431483893,4.54234690697773,
-33.6651940846335));
#27909=CARTESIAN_POINT('Ctrl Pts',(1.8561899212011,3.7134471707538,-33.7689883433836));
#27910=CARTESIAN_POINT('Ctrl Pts',(2.48364276907218,3.23615213332547,-33.8072572988311));
#27911=CARTESIAN_POINT('',(-4.0849984546357,0.00355325540345546,-33.2603849714311));
#27912=CARTESIAN_POINT('Ctrl Pts',(-4.0849984546357,0.00355325540344558,
-33.2603849714311));
#27913=CARTESIAN_POINT('Ctrl Pts',(-4.08485806388176,0.16495342166653,-33.2682457374445));
#27914=CARTESIAN_POINT('Ctrl Pts',(-4.07514796326737,0.325942653816538,
-33.2761065034578));
#27915=CARTESIAN_POINT('Ctrl Pts',(-4.0560388768652,0.485565267866275,-33.2839672694712));
#27916=CARTESIAN_POINT('Ctrl Pts',(-4.03692979046304,0.645187881916002,
-33.2918280354846));
#27917=CARTESIAN_POINT('Ctrl Pts',(-4.0084218836177,0.803444375325491,-33.299688801498));
#27918=CARTESIAN_POINT('Ctrl Pts',(-3.9707387557445,0.959405406295278,-33.3075495675114));
#27919=CARTESIAN_POINT('Ctrl Pts',(-3.94281256896416,1.07498490107533,-33.3133750186434));
#27920=CARTESIAN_POINT('Ctrl Pts',(-3.90979112428803,1.18952897197209,-33.3192004697754));
#27921=CARTESIAN_POINT('Ctrl Pts',(-3.87176638399298,1.3025552071916,-33.3250259209074));
#27922=CARTESIAN_POINT('Ctrl Pts',(-3.83378937110738,1.41543957558005,-33.3308440601238));
#27923=CARTESIAN_POINT('Ctrl Pts',(-3.79082168255022,1.52680951428498,-33.3366621993402));
#27924=CARTESIAN_POINT('Ctrl Pts',(-3.74300600338184,1.63619407731708,-33.3424803385566));
#27925=CARTESIAN_POINT('Ctrl Pts',(-3.6952379025852,1.74546979865763,-33.348292688509));
#27926=CARTESIAN_POINT('Ctrl Pts',(-3.64263157049037,1.85276370272238,-33.3541050384614));
#27927=CARTESIAN_POINT('Ctrl Pts',(-3.58537888812054,1.9576218298281,-33.3599173884137));
#27928=CARTESIAN_POINT('Ctrl Pts',(-3.52619241461574,2.06602168997119,-33.365926058789));
#27929=CARTESIAN_POINT('Ctrl Pts',(-3.46204030233133,2.17181789592515,-33.3719347291642));
#27930=CARTESIAN_POINT('Ctrl Pts',(-3.39318799183319,2.27453297449807,-33.3779433995394));
#27931=CARTESIAN_POINT('Ctrl Pts',(-3.32665946576081,2.3737813909045,-33.3837492756361));
#27932=CARTESIAN_POINT('Ctrl Pts',(-3.25574313323563,2.47015293580079,-33.3895551517327));
#27933=CARTESIAN_POINT('Ctrl Pts',(-3.18072384753942,2.56324419548626,-33.3953610278293));
#27934=CARTESIAN_POINT('Ctrl Pts',(-3.10571543191632,2.65632196652293,-33.4011660626716));
#27935=CARTESIAN_POINT('Ctrl Pts',(-3.02660550140437,2.74612008000037,-33.4069710975139));
#27936=CARTESIAN_POINT('Ctrl Pts',(-2.94371994149808,2.83226727305644,-33.4127761323563));
#27937=CARTESIAN_POINT('Ctrl Pts',(-2.86082686843711,2.91842227491765,-33.4185816933955));
#27938=CARTESIAN_POINT('Ctrl Pts',(-2.77415776842686,3.00092540433822,-33.4243872544347));
#27939=CARTESIAN_POINT('Ctrl Pts',(-2.68407575758724,3.07944188572093,-33.4301928154739));
#27940=CARTESIAN_POINT('Ctrl Pts',(-2.59396436334027,3.15798397800791,-33.4360002702005));
#27941=CARTESIAN_POINT('Ctrl Pts',(-2.50043815167015,3.23253656810522,-33.441807724927));
#27942=CARTESIAN_POINT('Ctrl Pts',(-2.4038932003654,3.30280524421847,-33.4476151796536));
#27943=CARTESIAN_POINT('Ctrl Pts',(-2.30724183291824,3.37315137359408,-33.4534290356153));
#27944=CARTESIAN_POINT('Ctrl Pts',(-2.20756541428628,3.43920392358034,-33.4592428915769));
#27945=CARTESIAN_POINT('Ctrl Pts',(-2.10528899843033,3.50071181805761,-33.4650567475385));
#27946=CARTESIAN_POINT('Ctrl Pts',(-2.002945292493,3.56226018003846,-33.470874428574));
#27947=CARTESIAN_POINT('Ctrl Pts',(-1.89799854028645,3.61925773741008,-33.4766921096095));
#27948=CARTESIAN_POINT('Ctrl Pts',(-1.79089690554167,3.67150013941458,-33.482509790645));
#27949=CARTESIAN_POINT('Ctrl Pts',(-1.68364350818876,3.72381656870356,-33.4883357153123));
#27950=CARTESIAN_POINT('Ctrl Pts',(-1.57422950683071,3.77136423237152,-33.4941616399796));
#27951=CARTESIAN_POINT('Ctrl Pts',(-1.46312156587967,3.81398745192716,-33.4999875646469));
#27952=CARTESIAN_POINT('Ctrl Pts',(-1.43681644442011,3.82407862054941,-33.5013668689043));
#27953=CARTESIAN_POINT('Ctrl Pts',(-1.41041643265913,3.83389398716217,-33.5027461731618));
#27954=CARTESIAN_POINT('Ctrl Pts',(-1.38392782194091,3.8434319017849,-33.5041254774192));
#27955=CARTESIAN_POINT('Ctrl Pts',(-1.2720539503939,3.88371500483929,-33.5099509285522));
#27956=CARTESIAN_POINT('Ctrl Pts',(-1.15824082603233,3.91917389249815,-33.5157763796852));
#27957=CARTESIAN_POINT('Ctrl Pts',(-1.04294185843482,3.94961989056219,-33.5216018308182));
#27958=CARTESIAN_POINT('Ctrl Pts',(-0.927787610327543,3.98002767380601,
-33.5274199700356));
#27959=CARTESIAN_POINT('Ctrl Pts',(-0.811151619532936,4.00543497911748,
-33.533238109253));
#27960=CARTESIAN_POINT('Ctrl Pts',(-0.693505633569845,4.02570179424742,
-33.5390562484704));
#27961=CARTESIAN_POINT('Ctrl Pts',(-0.575976709720327,4.04594844314563,
-33.5448685984238));
#27962=CARTESIAN_POINT('Ctrl Pts',(-0.457440189850825,4.06106470881374,
-33.5506809483772));
#27963=CARTESIAN_POINT('Ctrl Pts',(-0.338380709729531,4.07096100390104,
-33.5564932983306));
#27964=CARTESIAN_POINT('Ctrl Pts',(-0.215299825614357,4.08119156048979,
-33.5625019687055));
#27965=CARTESIAN_POINT('Ctrl Pts',(-0.091660457871997,4.08584316738755,
-33.5685106390803));
#27966=CARTESIAN_POINT('Ctrl Pts',(0.0319926461436455,4.08487471908169,
-33.5745193094552));
#27967=CARTESIAN_POINT('Ctrl Pts',(0.15147242390054,4.08393895617243,-33.5803251855528));
#27968=CARTESIAN_POINT('Ctrl Pts',(0.270964585161165,4.07775637691233,-33.5861310616504));
#27969=CARTESIAN_POINT('Ctrl Pts',(0.389975538435989,4.06634283840179,-33.591936937748));
#27970=CARTESIAN_POINT('Ctrl Pts',(0.508969247374796,4.05493095367932,-33.5977419725913));
#27971=CARTESIAN_POINT('Ctrl Pts',(0.627481480948872,4.03828965602805,-33.6035470074346));
#27972=CARTESIAN_POINT('Ctrl Pts',(0.745022913854255,4.01648675559028,-33.609352042278));
#27973=CARTESIAN_POINT('Ctrl Pts',(0.862575001292974,3.99468187883042,-33.6151576033182));
#27974=CARTESIAN_POINT('Ctrl Pts',(0.979155711911009,3.96771454345726,-33.6209631643584));
#27975=CARTESIAN_POINT('Ctrl Pts',(1.09428569935645,3.93570372464493,-33.6267687253986));
#27976=CARTESIAN_POINT('Ctrl Pts',(1.20945324048528,3.90368246438132,-33.6325761801261));
#27977=CARTESIAN_POINT('Ctrl Pts',(1.32316872443695,3.86661455812985,-33.6383836348537));
#27978=CARTESIAN_POINT('Ctrl Pts',(1.43496836976327,3.82466871477504,-33.6441910895812));
#27979=CARTESIAN_POINT('Ctrl Pts',(1.54689124563445,3.78267663684482,-33.6500049455439));
#27980=CARTESIAN_POINT('Ctrl Pts',(1.65689368556221,3.73579603311961,-33.6558188015065));
#27981=CARTESIAN_POINT('Ctrl Pts',(1.76453214759268,3.68424365373844,-33.6616326574691));
#27982=CARTESIAN_POINT('Ctrl Pts',(1.87224142752183,3.63265735682342,-33.6674503385056));
#27983=CARTESIAN_POINT('Ctrl Pts',(1.97758327299647,3.5763933546384,-33.673268019542));
#27984=CARTESIAN_POINT('Ctrl Pts',(2.08014044003778,3.51571340551522,-33.6790857005784));
#27985=CARTESIAN_POINT('Ctrl Pts',(2.18284293019341,3.4549474731357,-33.6849116252467));
#27986=CARTESIAN_POINT('Ctrl Pts',(2.28275252601363,3.38975332706837,-33.690737549915));
#27987=CARTESIAN_POINT('Ctrl Pts',(2.3794824434069,3.32043495667636,-33.6965634745832));
#27988=CARTESIAN_POINT('Ctrl Pts',(2.40238352667851,3.30402363518059,-33.6979427788312));
#27989=CARTESIAN_POINT('Ctrl Pts',(2.4251065366247,3.28738131410434,-33.6993220830791));
#27990=CARTESIAN_POINT('Ctrl Pts',(2.44764663355019,3.2705123386513,-33.700701387327));
#27991=CARTESIAN_POINT('Ctrl Pts',(2.4608407229129,3.2606379015395,-33.7015087779769));
#27992=CARTESIAN_POINT('Ctrl Pts',(2.47397797477153,3.25068143719705,-33.7023161686268));
#27993=CARTESIAN_POINT('Ctrl Pts',(2.4870572760686,3.24064362520074,-33.7031235592767));
#27994=CARTESIAN_POINT('Ctrl Pts',(2.48705727606859,3.24064362520075,-32.4530286559312));
#27995=CARTESIAN_POINT('Ctrl Pts',(2.58193246648303,3.16783091885943,-32.4588406338953));
#27996=CARTESIAN_POINT('Ctrl Pts',(2.67356128451973,3.09088376133001,-32.4646526118594));
#27997=CARTESIAN_POINT('Ctrl Pts',(2.76157813222159,3.01013475107602,-32.4704645898235));
#27998=CARTESIAN_POINT('Ctrl Pts',(2.84964039440292,2.92934407636387,-32.476279566622));
#27999=CARTESIAN_POINT('Ctrl Pts',(2.9340866845969,2.84474792911086,-32.4820945434205));
#28000=CARTESIAN_POINT('Ctrl Pts',(3.01458914627439,2.75671494339996,-32.487909520219));
#28001=CARTESIAN_POINT('Ctrl Pts',(3.09522071278122,2.66854077587476,-32.4937338227148));
#28002=CARTESIAN_POINT('Ctrl Pts',(3.17189555031696,2.57691906946114,-32.4995581252106));
#28003=CARTESIAN_POINT('Ctrl Pts',(3.24432651836811,2.48225108363627,-32.5053824277063));
#28004=CARTESIAN_POINT('Ctrl Pts',(3.31008596195785,2.39630284573328,-32.5106702610976));
#28005=CARTESIAN_POINT('Ctrl Pts',(3.37234774091624,2.30784423322459,-32.5159580944888));
#28006=CARTESIAN_POINT('Ctrl Pts',(3.43092935719941,2.21719389001215,-32.5212459278801));
#28007=CARTESIAN_POINT('Ctrl Pts',(3.49546700783304,2.11732706230663,-32.5270713790312));
#28008=CARTESIAN_POINT('Ctrl Pts',(3.55574392599387,2.01448031600678,-32.5328968301824));
#28009=CARTESIAN_POINT('Ctrl Pts',(3.6114737953513,1.90905265131449,-32.5387222813335));
#28010=CARTESIAN_POINT('Ctrl Pts',(3.66713371440342,1.80375731597123,-32.5445404205693));
#28011=CARTESIAN_POINT('Ctrl Pts',(3.71825774756252,1.69588786321235,-32.5503585598051));
#28012=CARTESIAN_POINT('Ctrl Pts',(3.76460283321834,1.5858721600824,-32.5561766990409));
#28013=CARTESIAN_POINT('Ctrl Pts',(3.81090180379914,1.47596592664773,-32.5619890490129));
#28014=CARTESIAN_POINT('Ctrl Pts',(3.85243112951132,1.36391806532641,-32.5678013989849));
#28015=CARTESIAN_POINT('Ctrl Pts',(3.88899395308434,1.2501804001317,-32.5736137489569));
#28016=CARTESIAN_POINT('Ctrl Pts',(3.92679173808193,1.13260108335458,-32.5796224193248));
#28017=CARTESIAN_POINT('Ctrl Pts',(3.95928137331307,1.01321618370378,-32.5856310896928));
#28018=CARTESIAN_POINT('Ctrl Pts',(3.98629963452622,0.892547042892467,-32.5916397600608));
#28019=CARTESIAN_POINT('Ctrl Pts',(4.01240602211043,0.775950518244885,-32.5974456361774));
#28020=CARTESIAN_POINT('Ctrl Pts',(4.03340430066207,0.658155470498375,-32.6032515122941));
#28021=CARTESIAN_POINT('Ctrl Pts',(4.04919830090484,0.539646291518178,-32.6090573884108));
#28022=CARTESIAN_POINT('Ctrl Pts',(4.06499001264393,0.42115428416572,-32.6148624232733));
#28023=CARTESIAN_POINT('Ctrl Pts',(4.07557889187928,0.301948755701678,-32.6206674581358));
#28024=CARTESIAN_POINT('Ctrl Pts',(4.08092034135956,0.182521690430972,-32.6264724929983));
#28025=CARTESIAN_POINT('Ctrl Pts',(4.08626227501516,0.0630837997020384,
-32.6322780540577));
#28026=CARTESIAN_POINT('Ctrl Pts',(4.08635581497202,-0.0565752601332626,
-32.6380836151172));
#28027=CARTESIAN_POINT('Ctrl Pts',(4.08120846023082,-0.175961655312674,
-32.6438891761767));
#28028=CARTESIAN_POINT('Ctrl Pts',(4.07605942649925,-0.29538699255423,-32.6496966309236));
#28029=CARTESIAN_POINT('Ctrl Pts',(4.06566611578164,-0.414539080835525,
-32.6555040856706));
#28030=CARTESIAN_POINT('Ctrl Pts',(4.0500879922333,-0.53292800186111,-32.6613115404175));
#28031=CARTESIAN_POINT('Ctrl Pts',(4.03449269778387,-0.65144741642437,-32.6671253963996));
#28032=CARTESIAN_POINT('Ctrl Pts',(4.01370123649887,-0.769201579913466,
-32.6729392523816));
#28033=CARTESIAN_POINT('Ctrl Pts',(3.9878244461349,-0.885709425719769,-32.6787531083636));
#28034=CARTESIAN_POINT('Ctrl Pts',(3.96193063081623,-1.00229392480375,-32.6845707894195));
#28035=CARTESIAN_POINT('Ctrl Pts',(3.93094492876804,-1.11763008004322,-32.6903884704754));
#28036=CARTESIAN_POINT('Ctrl Pts',(3.89502796685284,-1.23125226393062,-32.6962061515313));
#28037=CARTESIAN_POINT('Ctrl Pts',(3.8590601107404,-1.34503545001664,-32.7020320762189));
#28038=CARTESIAN_POINT('Ctrl Pts',(3.81814718789577,-1.45709943553806,-32.7078580009066));
#28039=CARTESIAN_POINT('Ctrl Pts',(3.77249785019351,-1.56699871419391,-32.7136839255942));
#28040=CARTESIAN_POINT('Ctrl Pts',(3.76169024103059,-1.5930176776835,-32.7150632296588));
#28041=CARTESIAN_POINT('Ctrl Pts',(3.75061734824109,-1.61891541630945,-32.7164425337233));
#28042=CARTESIAN_POINT('Ctrl Pts',(3.73928231007638,-1.64468623316116,-32.7178218377879));
#28043=CARTESIAN_POINT('Ctrl Pts',(3.69140910172012,-1.75352853847376,-32.7236472889164));
#28044=CARTESIAN_POINT('Ctrl Pts',(3.63870312742187,-1.86045299892141,-32.7294727400449));
#28045=CARTESIAN_POINT('Ctrl Pts',(3.58133999098287,-1.96500098447477,-32.7352981911735));
#28046=CARTESIAN_POINT('Ctrl Pts',(3.5240488548755,-2.06941774481803,-32.7411163303864));
#28047=CARTESIAN_POINT('Ctrl Pts',(3.46211237802662,-2.17146360865253,-32.7469344695993));
#28048=CARTESIAN_POINT('Ctrl Pts',(3.39575406965653,-2.27070017800922,-32.7527526088123));
#28049=CARTESIAN_POINT('Ctrl Pts',(3.32946179026127,-2.36983800330355,-32.7585649587611));
#28050=CARTESIAN_POINT('Ctrl Pts',(3.25875665807394,-2.46617175798871,-32.7643773087101));
#28051=CARTESIAN_POINT('Ctrl Pts',(3.18390761119513,-2.5592884408315,-32.7701896586589));
#28052=CARTESIAN_POINT('Ctrl Pts',(3.10653043076955,-2.65555027273732,-32.7761983290355));
#28053=CARTESIAN_POINT('Ctrl Pts',(3.02472466091164,-2.74837347420396,-32.782206999412));
#28054=CARTESIAN_POINT('Ctrl Pts',(2.938835793223,-2.83733487281134,-32.7882156697885));
#28055=CARTESIAN_POINT('Ctrl Pts',(2.85584569852113,-2.92329379966553,-32.7940215458817));
#28056=CARTESIAN_POINT('Ctrl Pts',(2.76904397598569,-3.00564707424169,-32.7998274219748));
#28057=CARTESIAN_POINT('Ctrl Pts',(2.678782163719,-3.08404784647401,-32.805633298068));
#28058=CARTESIAN_POINT('Ctrl Pts',(2.58853343012276,-3.1624372586656,-32.8114383329068));
#28059=CARTESIAN_POINT('Ctrl Pts',(2.49482591183162,-3.23687503999613,-32.8172433677456));
#28060=CARTESIAN_POINT('Ctrl Pts',(2.39804586548011,-3.30705322410356,-32.8230484025844));
#28061=CARTESIAN_POINT('Ctrl Pts',(2.30125704650927,-3.37723776950671,-32.8288539636202));
#28062=CARTESIAN_POINT('Ctrl Pts',(2.2013954760632,-3.44316171047454,-32.8346595246559));
#28063=CARTESIAN_POINT('Ctrl Pts',(2.09887762249836,-3.5045595623096,-32.8404650856916));
#28064=CARTESIAN_POINT('Ctrl Pts',(1.9963263291404,-3.56597744120718,-32.8462725404147));
#28065=CARTESIAN_POINT('Ctrl Pts',(1.89111737934565,-3.62286608529565,-32.8520799951377));
#28066=CARTESIAN_POINT('Ctrl Pts',(1.78369256745013,-3.67500555439351,-32.8578874498608));
#28067=CARTESIAN_POINT('Ctrl Pts',(1.67614934714406,-3.72720249393562,-32.863701305819));
#28068=CARTESIAN_POINT('Ctrl Pts',(1.5663857568185,-3.77463963142747,-32.8695151617772));
#28069=CARTESIAN_POINT('Ctrl Pts',(1.45486446961969,-3.81714479356472,-32.8753290177354));
#28070=CARTESIAN_POINT('Ctrl Pts',(1.34326980991886,-3.85967792085707,-32.8811466987674));
#28071=CARTESIAN_POINT('Ctrl Pts',(1.22991553661569,-3.89727248232742,-32.8869643797995));
#28072=CARTESIAN_POINT('Ctrl Pts',(1.11527882938665,-3.92980637343902,-32.8927820608315));
#28073=CARTESIAN_POINT('Ctrl Pts',(1.00047968237937,-3.96238636495062,-32.8986079854955));
#28074=CARTESIAN_POINT('Ctrl Pts',(0.884394870114934,-3.98989128010835,
-32.9044339101594));
#28075=CARTESIAN_POINT('Ctrl Pts',(0.76751119858735,-4.01225018662134,-32.9102598348234));
#28076=CARTESIAN_POINT('Ctrl Pts',(0.739838655778987,-4.01754372154836,
-32.9116391391142));
#28077=CARTESIAN_POINT('Ctrl Pts',(0.712121353475551,-4.02254904212186,
-32.913018443405));
#28078=CARTESIAN_POINT('Ctrl Pts',(0.6843657754055,-4.02726563383316,-32.9143977476958));
#28079=CARTESIAN_POINT('Ctrl Pts',(0.567140907239768,-4.04718602029217,
-32.9202231988263));
#28080=CARTESIAN_POINT('Ctrl Pts',(0.448858034774041,-4.06201578964598,
-32.9260486499569));
#28081=CARTESIAN_POINT('Ctrl Pts',(0.32999673641773,-4.0716491933802,-32.9318741010875));
#28082=CARTESIAN_POINT('Ctrl Pts',(0.211284628873984,-4.08127050558126,
-32.9376922403025));
#28083=CARTESIAN_POINT('Ctrl Pts',(0.0919959426583443,-4.08570839247379,
-32.9435103795174));
#28084=CARTESIAN_POINT('Ctrl Pts',(-0.0273802758723824,-4.08490823893183,
-32.9493285187323));
#28085=CARTESIAN_POINT('Ctrl Pts',(-0.146637710644032,-4.08410888157228,
-32.9551408686833));
#28086=CARTESIAN_POINT('Ctrl Pts',(-0.265982098758161,-4.07808185543052,
-32.9609532186342));
#28087=CARTESIAN_POINT('Ctrl Pts',(-0.384920601103282,-4.06682445291732,
-32.9667655685851));
#28088=CARTESIAN_POINT('Ctrl Pts',(-0.507876421316165,-4.05518681554856,
-32.9727742389609));
#28089=CARTESIAN_POINT('Ctrl Pts',(-0.630398008995281,-4.03795918482162,
-32.9787829093366));
#28090=CARTESIAN_POINT('Ctrl Pts',(-0.751941906517641,-4.01519717687969,
-32.9847915797124));
#28091=CARTESIAN_POINT('Ctrl Pts',(-0.869383664010096,-3.99320339297733,
-32.9905974558074));
#28092=CARTESIAN_POINT('Ctrl Pts',(-0.985912228050297,-3.96604285837032,
-32.9964033319025));
#28093=CARTESIAN_POINT('Ctrl Pts',(-1.10104454147099,-3.93381823648436,
-33.0022092079975));
#28094=CARTESIAN_POINT('Ctrl Pts',(-1.21616017255858,-3.9015982838512,-33.0080142428382));
#28095=CARTESIAN_POINT('Ctrl Pts',(-1.3298795625645,-3.86431581317818,-33.0138192776789));
#28096=CARTESIAN_POINT('Ctrl Pts',(-1.44173301660593,-3.8221238740821,-33.0196243125196));
#28097=CARTESIAN_POINT('Ctrl Pts',(-1.5535966095935,-3.77992811050155,-33.0254298735572));
#28098=CARTESIAN_POINT('Ctrl Pts',(-1.66359354855399,-3.73282213770339,
-33.0312354345947));
#28099=CARTESIAN_POINT('Ctrl Pts',(-1.77127298511989,-3.68100760827582,
-33.0370409956323));
#28100=CARTESIAN_POINT('Ctrl Pts',(-1.87898754511049,-3.62917617772227,
-33.0428484503571));
#28101=CARTESIAN_POINT('Ctrl Pts',(-1.98438273183416,-3.572633312846,-33.048655905082));
#28102=CARTESIAN_POINT('Ctrl Pts',(-2.08703178938166,-3.51162687512645,
-33.0544633598069));
#28103=CARTESIAN_POINT('Ctrl Pts',(-2.18979399128881,-3.45055319339614,
-33.0602772157669));
#28104=CARTESIAN_POINT('Ctrl Pts',(-2.28980367123861,-3.38500632695112,
-33.0660910717268));
#28105=CARTESIAN_POINT('Ctrl Pts',(-2.38666246859223,-3.31527785577819,
-33.0719049276868));
#28106=CARTESIAN_POINT('Ctrl Pts',(-2.48358499164677,-3.24550350858965,
-33.0777226087205));
#28107=CARTESIAN_POINT('Ctrl Pts',(-2.57735218392528,-3.17154232964677,
-33.0835402897542));
#28108=CARTESIAN_POINT('Ctrl Pts',(-2.66759950862442,-3.09372556339226,
-33.089357970788));
#28109=CARTESIAN_POINT('Ctrl Pts',(-2.75797471343884,-3.01579853107643,
-33.0951838954536));
#28110=CARTESIAN_POINT('Ctrl Pts',(-2.84481980007433,-2.93400528603584,
-33.1010098201192));
#28111=CARTESIAN_POINT('Ctrl Pts',(-2.92780766242373,-2.84871326950482,
-33.1068357447847));
#28112=CARTESIAN_POINT('Ctrl Pts',(-2.94745527541399,-2.82852014144347,
-33.1082150490577));
#28113=CARTESIAN_POINT('Ctrl Pts',(-2.96688686509319,-2.80813104182631,
-33.1095943533306));
#28114=CARTESIAN_POINT('Ctrl Pts',(-2.98609843399859,-2.78755110132015,
-33.1109736576035));
#28115=CARTESIAN_POINT('Ctrl Pts',(-3.06626583517473,-2.70167366180113,
-33.1167293165784));
#28116=CARTESIAN_POINT('Ctrl Pts',(-3.14286955276453,-2.61218061687391,
-33.1224849755533));
#28117=CARTESIAN_POINT('Ctrl Pts',(-3.21556074940212,-2.51940351410895,
-33.1282406345282));
#28118=CARTESIAN_POINT('Ctrl Pts',(-3.28813850960451,-2.42677119233938,
-33.1339873116529));
#28119=CARTESIAN_POINT('Ctrl Pts',(-3.35681564336712,-2.3308653382591,-33.1397339887777));
#28120=CARTESIAN_POINT('Ctrl Pts',(-3.42128067654142,-2.23205365802982,
-33.1454806659024));
#28121=CARTESIAN_POINT('Ctrl Pts',(-3.48568814733276,-2.13333020913306,
-33.1512222116805));
#28122=CARTESIAN_POINT('Ctrl Pts',(-3.54589076438995,-2.03170643895666,
-33.1569637574586));
#28123=CARTESIAN_POINT('Ctrl Pts',(-3.60161793196347,-1.92758223486293,
-33.1627053032367));
#28124=CARTESIAN_POINT('Ctrl Pts',(-3.65730926590799,-1.82352498461347,
-33.1684431570917));
#28125=CARTESIAN_POINT('Ctrl Pts',(-3.70853067401423,-1.71697086465564,
-33.1741810109466));
#28126=CARTESIAN_POINT('Ctrl Pts',(-3.75505586227218,-1.60834712398018,
-33.1799188648016));
#28127=CARTESIAN_POINT('Ctrl Pts',(-3.80156275802397,-1.49976609136288,
-33.1856544626801));
#28128=CARTESIAN_POINT('Ctrl Pts',(-3.84337694153011,-1.38911744095059,
-33.1913900605586));
#28129=CARTESIAN_POINT('Ctrl Pts',(-3.88031925962283,-1.27685059556712,
-33.1971256584372));
#28130=CARTESIAN_POINT('Ctrl Pts',(-3.91726724257214,-1.16456653481628,
-33.2028621358312));
#28131=CARTESIAN_POINT('Ctrl Pts',(-3.94934172727531,-1.05066417837745,
-33.2085986132252));
#28132=CARTESIAN_POINT('Ctrl Pts',(-3.97641280845001,-0.935610055949977,
-33.2143350906191));
#28133=CARTESIAN_POINT('Ctrl Pts',(-4.00348552924101,-0.82054896503038,
-33.2200719154548));
#28134=CARTESIAN_POINT('Ctrl Pts',(-4.02555415539019,-0.704336379157422,
-33.2258087402905));
#28135=CARTESIAN_POINT('Ctrl Pts',(-4.04253976856566,-0.587449759183785,
-33.2315455651261));
#28136=CARTESIAN_POINT('Ctrl Pts',(-4.05953874277468,-0.47047119516113,
-33.237286902599));
#28137=CARTESIAN_POINT('Ctrl Pts',(-4.07144666714239,-0.352817954335272,
-33.2430282400718));
#28138=CARTESIAN_POINT('Ctrl Pts',(-4.0782364528454,-0.234973263761964,
-33.2487695775446));
#28139=CARTESIAN_POINT('Ctrl Pts',(-4.08281529505991,-0.155502089331045,
-33.2526413754979));
#28140=CARTESIAN_POINT('Ctrl Pts',(-4.08506760369229,-0.0759439382077033,
-33.2565131734512));
#28141=CARTESIAN_POINT('Ctrl Pts',(-4.08499845463617,0.00355325485717703,
-33.2603849714045));
#28142=CARTESIAN_POINT('Origin',(0.,0.,-25.2396150285955));
#28143=CARTESIAN_POINT('',(2.48705727606859,3.24064362520075,-31.2032093449099));
#28144=CARTESIAN_POINT('',(2.4870572760686,3.24064362520075,-31.3072405360316));
#28145=CARTESIAN_POINT('',(2.4870572760686,3.24064362520075,-25.2396150285955));
#28146=CARTESIAN_POINT('',(-4.08499995078438,0.000634106917209552,-32.1146150285602));
#28147=CARTESIAN_POINT('Ctrl Pts',(2.4870572760686,3.24064362520075,-31.3072405360316));
#28148=CARTESIAN_POINT('Ctrl Pts',(2.58177343908692,3.16795296567738,-31.3130657305817));
#28149=CARTESIAN_POINT('Ctrl Pts',(2.6731893400469,3.09119144240212,-31.3188909251318));
#28150=CARTESIAN_POINT('Ctrl Pts',(2.76095535213861,3.01070598755461,-31.3247161196819));
#28151=CARTESIAN_POINT('Ctrl Pts',(2.80526826965443,2.97006901161277,-31.3276572509862));
#28152=CARTESIAN_POINT('Ctrl Pts',(2.84865135640308,2.92848328490921,-31.3305983822904));
#28153=CARTESIAN_POINT('Ctrl Pts',(2.89106349316248,2.88599668719546,-31.3335395135947));
#28154=CARTESIAN_POINT('Ctrl Pts',(2.97506852242191,2.80184417433516,-31.3393649645186));
#28155=CARTESIAN_POINT('Ctrl Pts',(3.05553064445705,2.71388619702605,-31.3451904154425));
#28156=CARTESIAN_POINT('Ctrl Pts',(3.13208639459978,2.62245301516785,-31.3510158663664));
#28157=CARTESIAN_POINT('Ctrl Pts',(3.20854605442018,2.53113459730713,-31.3568340053711));
#28158=CARTESIAN_POINT('Ctrl Pts',(3.28110883514576,2.43634996104282,-31.3626521443759));
#28159=CARTESIAN_POINT('Ctrl Pts',(3.34944752932834,2.338466644679,-31.3684702833806));
#28160=CARTESIAN_POINT('Ctrl Pts',(3.4177182239378,2.24068072589948,-31.374282633118));
#28161=CARTESIAN_POINT('Ctrl Pts',(3.48177296152747,2.13980259365382,-31.3800949828554));
#28162=CARTESIAN_POINT('Ctrl Pts',(3.54132470353108,2.03623288063043,-31.3859073325929));
#28163=CARTESIAN_POINT('Ctrl Pts',(3.60288789378296,1.92916494722211,-31.3919160030474));
#28164=CARTESIAN_POINT('Ctrl Pts',(3.65963822815731,1.8192207308402,-31.397924673502));
#28165=CARTESIAN_POINT('Ctrl Pts',(3.71130701083638,1.70687588046606,-31.4039333439566));
#28166=CARTESIAN_POINT('Ctrl Pts',(3.7612319553154,1.5983227052873,-31.4097392198314));
#28167=CARTESIAN_POINT('Ctrl Pts',(3.80641263717735,1.48752872590933,-31.4155450957062));
#28168=CARTESIAN_POINT('Ctrl Pts',(3.84665366265959,1.3749474897419,-31.421350971581));
#28169=CARTESIAN_POINT('Ctrl Pts',(3.88688885732084,1.26238256630575,-31.4271560061993));
#28170=CARTESIAN_POINT('Ctrl Pts',(3.92218568174725,1.1480312852159,-31.4329610408177));
#28171=CARTESIAN_POINT('Ctrl Pts',(3.95239758401236,1.03236540909374,-31.438766075436));
#28172=CARTESIAN_POINT('Ctrl Pts',(3.98261222482297,0.916689048485613,-31.4445716362493));
#28173=CARTESIAN_POINT('Ctrl Pts',(4.00774092393238,0.799698250713554,-31.4503771970627));
#28174=CARTESIAN_POINT('Ctrl Pts',(4.02768768552435,0.681877487438528,-31.456182757876));
#28175=CARTESIAN_POINT('Ctrl Pts',(4.04764095344671,0.564018292821727,-31.461990212375));
#28176=CARTESIAN_POINT('Ctrl Pts',(4.06240885417604,0.44532899636973,-31.467797666874));
#28177=CARTESIAN_POINT('Ctrl Pts',(4.07194702605262,0.326301114036093,-31.473605121373));
#28178=CARTESIAN_POINT('Ctrl Pts',(4.08149571132497,0.207142033895291,-31.4794189771057));
#28179=CARTESIAN_POINT('Ctrl Pts',(4.08580312905233,0.0876440298755329,
-31.4852328328385));
#28180=CARTESIAN_POINT('Ctrl Pts',(4.08487700611757,-0.0316992885084958,
-31.4910466885712));
#28181=CARTESIAN_POINT('Ctrl Pts',(4.0839502738647,-0.151121125675586,-31.4968643693767));
#28182=CARTESIAN_POINT('Ctrl Pts',(4.07778316450658,-0.270387668005049,
-31.5026820501822));
#28183=CARTESIAN_POINT('Ctrl Pts',(4.06643532238445,-0.389009985558321,
-31.5084997309877));
#28184=CARTESIAN_POINT('Ctrl Pts',(4.05507140041231,-0.507800390493599,
-31.5143256554252));
#28185=CARTESIAN_POINT('Ctrl Pts',(4.03851215027927,-0.625944346112009,
-31.5201515798628));
#28186=CARTESIAN_POINT('Ctrl Pts',(4.01686838841442,-0.742962549632821,
-31.5259775043003));
#28187=CARTESIAN_POINT('Ctrl Pts',(4.01174415798604,-0.770666986731162,
-31.527356810701));
#28188=CARTESIAN_POINT('Ctrl Pts',(4.006335150232,-0.79830838953125,-31.5287361171018));
#28189=CARTESIAN_POINT('Ctrl Pts',(4.00064324193696,-0.825880530551567,
-31.5301154235025));
#28190=CARTESIAN_POINT('Ctrl Pts',(3.97660367076272,-0.942330482329761,
-31.53594087477));
#28191=CARTESIAN_POINT('Ctrl Pts',(3.94743702183402,-1.05791623962973,-31.5417663260374));
#28192=CARTESIAN_POINT('Ctrl Pts',(3.91321904908743,-1.17215258130468,-31.5475917773049));
#28193=CARTESIAN_POINT('Ctrl Pts',(3.87904402560938,-1.28624553729893,-31.5534099166584));
#28194=CARTESIAN_POINT('Ctrl Pts',(3.83983040525071,-1.39899205908764,-31.559228056012));
#28195=CARTESIAN_POINT('Ctrl Pts',(3.79570502028427,-1.50991668610847,-31.5650461953655));
#28196=CARTESIAN_POINT('Ctrl Pts',(3.75162354169778,-1.62073093904817,-31.5708585454566));
#28197=CARTESIAN_POINT('Ctrl Pts',(3.70264017151582,-1.72972652676446,-31.5766708955476));
#28198=CARTESIAN_POINT('Ctrl Pts',(3.64893147927402,-1.83644331781929,-31.5824832456386));
#28199=CARTESIAN_POINT('Ctrl Pts',(3.59340870102602,-1.9467646173661,-31.5884919159625));
#28200=CARTESIAN_POINT('Ctrl Pts',(3.53283586916301,-2.0546500308498,-31.5945005862863));
#28201=CARTESIAN_POINT('Ctrl Pts',(3.46746228396593,-2.15961346293122,-31.6005092566101));
#28202=CARTESIAN_POINT('Ctrl Pts',(3.40429507317844,-2.2610343536362,-31.6063151328482));
#28203=CARTESIAN_POINT('Ctrl Pts',(3.33664616612951,-2.35972694152215,-31.6121210090864));
#28204=CARTESIAN_POINT('Ctrl Pts',(3.26478674532157,-2.45527849898389,-31.6179268853245));
#28205=CARTESIAN_POINT('Ctrl Pts',(3.19293773672137,-2.55081621132059,-31.6237319203091));
#28206=CARTESIAN_POINT('Ctrl Pts',(3.11687967285738,-2.64321347236129,-31.6295369552937));
#28207=CARTESIAN_POINT('Ctrl Pts',(3.03692582220991,-2.73208831306652,-31.6353419902784));
#28208=CARTESIAN_POINT('Ctrl Pts',(2.9569647241434,-2.82097120983418,-31.6411475514606));
#28209=CARTESIAN_POINT('Ctrl Pts',(2.87310741007591,-2.90633074809517,-31.6469531126428));
#28210=CARTESIAN_POINT('Ctrl Pts',(2.78570558024516,-2.98782017869064,-31.6527586738249));
#28211=CARTESIAN_POINT('Ctrl Pts',(2.69827524123529,-3.06933618992839,-31.658566128695));
#28212=CARTESIAN_POINT('Ctrl Pts',(2.60729838534707,-3.14697930480428,-31.664373583565));
#28213=CARTESIAN_POINT('Ctrl Pts',(2.51316100784573,-3.2204420113773,-31.6701810384351));
#28214=CARTESIAN_POINT('Ctrl Pts',(2.41891986793911,-3.29398569181356,-31.6759948945402));
#28215=CARTESIAN_POINT('Ctrl Pts',(2.3215115746994,-3.36333951534805,-31.6818087506454));
#28216=CARTESIAN_POINT('Ctrl Pts',(2.22135253469191,-3.42823831094308,-31.6876226067505));
#28217=CARTESIAN_POINT('Ctrl Pts',(2.12112759767327,-3.49317980499704,-31.6934402879297));
#28218=CARTESIAN_POINT('Ctrl Pts',(2.01814866060833,-3.55366022757815,-31.6992579691088));
#28219=CARTESIAN_POINT('Ctrl Pts',(1.91285679177796,-3.60946033281278,-31.705075650288));
#28220=CARTESIAN_POINT('Ctrl Pts',(1.80741572478954,-3.6653395065739,-31.7109015750982));
#28221=CARTESIAN_POINT('Ctrl Pts',(1.69965555194913,-3.71652495199247,-31.7167274999084));
#28222=CARTESIAN_POINT('Ctrl Pts',(1.59003746195505,-3.76284544853752,-31.7225534247185));
#28223=CARTESIAN_POINT('Ctrl Pts',(1.56408509318158,-3.77381194693366,-31.7239327276158));
#28224=CARTESIAN_POINT('Ctrl Pts',(1.53802865048042,-3.78450597661719,-31.725312030513));
#28225=CARTESIAN_POINT('Ctrl Pts',(1.51187436638704,-3.7949256778311,-31.7266913334103));
#28226=CARTESIAN_POINT('Ctrl Pts',(1.40141240502279,-3.83893302396254,-31.7325167845219));
#28227=CARTESIAN_POINT('Ctrl Pts',(1.28885070777441,-3.87818380994179,-31.7383422356336));
#28228=CARTESIAN_POINT('Ctrl Pts',(1.1746361108397,-3.91247428197444,-31.7441676867452));
#28229=CARTESIAN_POINT('Ctrl Pts',(1.06056487232927,-3.94672171372878,-31.7499858259413));
#28230=CARTESIAN_POINT('Ctrl Pts',(0.944845248067957,-3.97602109890178,
-31.7558039651373));
#28231=CARTESIAN_POINT('Ctrl Pts',(0.827944031676047,-4.00021670418141,
-31.7616221043334));
#28232=CARTESIAN_POINT('Ctrl Pts',(0.711159136324298,-4.02438823393762,
-31.7674344542655));
#28233=CARTESIAN_POINT('Ctrl Pts',(0.593195385143151,-4.04346600473028,
-31.7732468041975));
#28234=CARTESIAN_POINT('Ctrl Pts',(0.474534141585862,-4.05734424820835,
-31.7790591541296));
#28235=CARTESIAN_POINT('Ctrl Pts',(0.351864944429789,-4.07169124925397,
-31.7850678245124));
#28236=CARTESIAN_POINT('Ctrl Pts',(0.228450728635298,-4.08048113494708,
-31.7910764948953));
#28237=CARTESIAN_POINT('Ctrl Pts',(0.104834559263976,-4.08365457833837,
-31.7970851652781));
#28238=CARTESIAN_POINT('Ctrl Pts',(-0.014609529809033,-4.08672091712742,
-31.8028910413546));
#28239=CARTESIAN_POINT('Ctrl Pts',(-0.134241720055493,-4.08454379782612,
-31.8086969174311));
#28240=CARTESIAN_POINT('Ctrl Pts',(-0.253568165814577,-4.07712253743807,
-31.8145027935076));
#28241=CARTESIAN_POINT('Ctrl Pts',(-0.372877321525938,-4.06970235236862,
-31.8203078283299));
#28242=CARTESIAN_POINT('Ctrl Pts',(-0.491880413732094,-4.05703956271141,
-31.8261128631522));
#28243=CARTESIAN_POINT('Ctrl Pts',(-0.610086120570589,-4.03918555224777,
-31.8319178979745));
#28244=CARTESIAN_POINT('Ctrl Pts',(-0.728302542158392,-4.02132992340841,
-31.8377234589938));
#28245=CARTESIAN_POINT('Ctrl Pts',(-0.845721031212787,-3.99828219911942,
-31.8435290200131));
#28246=CARTESIAN_POINT('Ctrl Pts',(-0.961858525623113,-3.97014523370193,
-31.8493345810324));
#28247=CARTESIAN_POINT('Ctrl Pts',(-1.07803390235364,-3.94199909042557,
-31.8551420357393));
#28248=CARTESIAN_POINT('Ctrl Pts',(-1.19292705710286,-3.90876050056796,
-31.8609494904461));
#28249=CARTESIAN_POINT('Ctrl Pts',(-1.30606881826721,-3.87058254555436,
-31.8667569451529));
#28250=CARTESIAN_POINT('Ctrl Pts',(-1.41933528932348,-3.83236250909714,
-31.8725708010951));
#28251=CARTESIAN_POINT('Ctrl Pts',(-1.53084612668865,-3.78919237076018,
-31.8783846570374));
#28252=CARTESIAN_POINT('Ctrl Pts',(-1.64015077791753,-3.74127390412631,
-31.8841985129796));
#28253=CARTESIAN_POINT('Ctrl Pts',(-1.74952734327411,-3.69332391079444,
-31.8900161939959));
#28254=CARTESIAN_POINT('Ctrl Pts',(-1.85669446646886,-3.64061954711204,
-31.8958338750121));
#28255=CARTESIAN_POINT('Ctrl Pts',(-1.96122637087928,-3.58340845036784,
-31.9016515560283));
#28256=CARTESIAN_POINT('Ctrl Pts',(-2.06590639660719,-3.5261162857136,-31.9074774806768));
#28257=CARTESIAN_POINT('Ctrl Pts',(-2.16794340309138,-3.46430485296478,
-31.9133034053253));
#28258=CARTESIAN_POINT('Ctrl Pts',(-2.26694064212117,-3.3982650169019,-31.9191293299737));
#28259=CARTESIAN_POINT('Ctrl Pts',(-2.29037852372566,-3.38262989541779,
-31.9205086344219));
#28260=CARTESIAN_POINT('Ctrl Pts',(-2.31364616841575,-3.36675793990398,
-31.92188793887));
#28261=CARTESIAN_POINT('Ctrl Pts',(-2.33673859368093,-3.3506533310389,-31.9232672433182));
#28262=CARTESIAN_POINT('Ctrl Pts',(-2.43384640131928,-3.28293055000565,
-31.9290674669623));
#28263=CARTESIAN_POINT('Ctrl Pts',(-2.52816984019052,-3.21086960220254,
-31.9348676906065));
#28264=CARTESIAN_POINT('Ctrl Pts',(-2.61929494263886,-3.13472789943027,
-31.9406679142507));
#28265=CARTESIAN_POINT('Ctrl Pts',(-2.71030537162278,-3.05868201474334,
-31.9464608387894));
#28266=CARTESIAN_POINT('Ctrl Pts',(-2.7981251548425,-2.97856584921579,-31.952253763328));
#28267=CARTESIAN_POINT('Ctrl Pts',(-2.88236925872762,-2.89468002659051,
-31.9580466878667));
#28268=CARTESIAN_POINT('Ctrl Pts',(-2.96652979121779,-2.81087741993986,
-31.9638338657387));
#28269=CARTESIAN_POINT('Ctrl Pts',(-3.04712140956654,-2.72331288349971,
-31.9696210436106));
#28270=CARTESIAN_POINT('Ctrl Pts',(-3.12379265800122,-2.63232680908311,
-31.9754082214826));
#28271=CARTESIAN_POINT('Ctrl Pts',(-3.20063753764538,-2.541134685822,-31.9812085051108));
#28272=CARTESIAN_POINT('Ctrl Pts',(-3.27354395713333,-2.44650578476795,
-31.9870087887391));
#28273=CARTESIAN_POINT('Ctrl Pts',(-3.34219549847513,-2.34881975680821,
-31.9928090723673));
#28274=CARTESIAN_POINT('Ctrl Pts',(-3.41061798646001,-2.25145965470812,
-31.9985900035613));
#28275=CARTESIAN_POINT('Ctrl Pts',(-3.47481370569665,-2.15106313236277,
-32.0043709347554));
#28276=CARTESIAN_POINT('Ctrl Pts',(-3.53451060025972,-2.04803804082143,
-32.0101518659494));
#28277=CARTESIAN_POINT('Ctrl Pts',(-3.59419958651706,-1.94502659745942,
-32.0159320313185));
#28278=CARTESIAN_POINT('Ctrl Pts',(-3.64939072674739,-1.83938763382505,
-32.0217121966876));
#28279=CARTESIAN_POINT('Ctrl Pts',(-3.69985673480307,-1.73155569992199,
-32.0274923620567));
#28280=CARTESIAN_POINT('Ctrl Pts',(-3.75032822749171,-1.62371204687171,
-32.0332731556127));
#28281=CARTESIAN_POINT('Ctrl Pts',(-3.79607339270388,-1.51367532307134,
-32.0390539491687));
#28282=CARTESIAN_POINT('Ctrl Pts',(-3.83691241130101,-1.40190161851833,
-32.0448347427246));
#28283=CARTESIAN_POINT('Ctrl Pts',(-3.87799325316331,-1.28946605961315,
-32.0506497665443));
#28284=CARTESIAN_POINT('Ctrl Pts',(-3.91410950446023,-1.17527327558181,
-32.0564647903639));
#28285=CARTESIAN_POINT('Ctrl Pts',(-3.94512885569573,-1.05980343081013,
-32.0622798141835));
#28286=CARTESIAN_POINT('Ctrl Pts',(-3.97601037479555,-0.94484666754007,
-32.0680689993856));
#28287=CARTESIAN_POINT('Ctrl Pts',(-4.00184016039536,-0.828624585574513,
-32.0738581845877));
#28288=CARTESIAN_POINT('Ctrl Pts',(-4.02253913335644,-0.711620629700959,
-32.0796473697899));
#28289=CARTESIAN_POINT('Ctrl Pts',(-4.04337668355074,-0.593833345856952,
-32.0854753129182));
#28290=CARTESIAN_POINT('Ctrl Pts',(-4.05901441865793,-0.475254101590422,
-32.0913032560466));
#28291=CARTESIAN_POINT('Ctrl Pts',(-4.0694248419718,-0.356379650854012,
-32.097131199175));
#28292=CARTESIAN_POINT('Ctrl Pts',(-4.07983526528566,-0.237505200117603,
-32.1029591423034));
#28293=CARTESIAN_POINT('Ctrl Pts',(-4.08501841828653,-0.118335964697111,
-32.1087870854318));
#28294=CARTESIAN_POINT('Ctrl Pts',(-4.08499995078438,0.000634106917214494,
-32.1146150285602));
#28295=CARTESIAN_POINT('Ctrl Pts',(-4.08499995078427,0.000634107638191378,
-32.1146150285955));
#28296=CARTESIAN_POINT('Ctrl Pts',(-4.08499442850935,0.0362092867362075,
-32.1163577368056));
#28297=CARTESIAN_POINT('Ctrl Pts',(-4.08452419335079,0.0717803130156109,
-32.1181004450158));
#28298=CARTESIAN_POINT('Ctrl Pts',(-4.08358951442185,0.107339078177262,
-32.1198431532259));
#28299=CARTESIAN_POINT('Ctrl Pts',(-4.08046510930863,0.226203411426466,
-32.1256686043772));
#28300=CARTESIAN_POINT('Ctrl Pts',(-4.07214158107509,0.345121361988938,
-32.1314940555285));
#28301=CARTESIAN_POINT('Ctrl Pts',(-4.0586079174886,0.463601954373402,-32.1373195066798));
#28302=CARTESIAN_POINT('Ctrl Pts',(-4.04509124091304,0.581933833801863,
-32.1431376459158));
#28303=CARTESIAN_POINT('Ctrl Pts',(-4.02637748224907,0.699829045080311,
-32.1489557851517));
#28304=CARTESIAN_POINT('Ctrl Pts',(-4.00250762836785,0.816797211587529,
-32.1547739243877));
#28305=CARTESIAN_POINT('Ctrl Pts',(-3.97866152587439,0.933648990441425,
-32.1605862743599));
#28306=CARTESIAN_POINT('Ctrl Pts',(-3.94966961600344,1.04957516213541,-32.166398624332));
#28307=CARTESIAN_POINT('Ctrl Pts',(-3.91562454680484,1.16409166669097,-32.1722109743042));
#28308=CARTESIAN_POINT('Ctrl Pts',(-3.88042955692181,1.28247612923273,-32.1782196446721));
#28309=CARTESIAN_POINT('Ctrl Pts',(-3.83983406048606,1.39935357072967,-32.18422831504));
#28310=CARTESIAN_POINT('Ctrl Pts',(-3.79399771690724,1.51420154672442,-32.1902369854079));
#28311=CARTESIAN_POINT('Ctrl Pts',(-3.74970836232903,1.62517337244771,-32.1960428615247));
#28312=CARTESIAN_POINT('Ctrl Pts',(-3.70052637554683,1.73425010302123,-32.2018487376416));
#28313=CARTESIAN_POINT('Ctrl Pts',(-3.64664589504588,1.8409776522666,-32.2076546137584));
#28314=CARTESIAN_POINT('Ctrl Pts',(-3.5927732216664,1.94768973700732,-32.2134596486211));
#28315=CARTESIAN_POINT('Ctrl Pts',(-3.53420359234195,2.05205295323479,-32.2192646834837));
#28316=CARTESIAN_POINT('Ctrl Pts',(-3.47117799669026,2.15363606844179,-32.2250697183464));
#28317=CARTESIAN_POINT('Ctrl Pts',(-3.40814668808747,2.25522839164378,-32.230875279406));
#28318=CARTESIAN_POINT('Ctrl Pts',(-3.34065882520363,2.35403976606273,-32.2366808404657));
#28319=CARTESIAN_POINT('Ctrl Pts',(-3.26899943869611,2.44966684873771,-32.2424864015253));
#28320=CARTESIAN_POINT('Ctrl Pts',(-3.19731667796541,2.54532512354091,-32.2482938562724));
#28321=CARTESIAN_POINT('Ctrl Pts',(-3.12145993202294,2.6377967145576,-32.2541013110195));
#28322=CARTESIAN_POINT('Ctrl Pts',(-3.04175490922273,2.72671085233095,-32.2599087657666));
#28323=CARTESIAN_POINT('Ctrl Pts',(-2.9619620319989,2.81572299522433,-32.2657226217488));
#28324=CARTESIAN_POINT('Ctrl Pts',(-2.8783126837044,2.9011695540318,-32.271536477731));
#28325=CARTESIAN_POINT('Ctrl Pts',(-2.79116997494235,2.98271607280685,-32.2773503337132));
#28326=CARTESIAN_POINT('Ctrl Pts',(-2.70396993292371,3.06431624297226,-32.2831680147693));
#28327=CARTESIAN_POINT('Ctrl Pts',(-2.61327226225792,3.1420109980932,-32.2889856958253));
#28328=CARTESIAN_POINT('Ctrl Pts',(-2.51947244850089,3.2155067378634,-32.2948033768814));
#28329=CARTESIAN_POINT('Ctrl Pts',(-2.4255397207676,3.28910662081492,-32.3006293015692));
#28330=CARTESIAN_POINT('Ctrl Pts',(-2.32849640733948,3.35849537657707,-32.306455226257));
#28331=CARTESIAN_POINT('Ctrl Pts',(-2.22876626902628,3.42342312869016,-32.3122811509447));
#28332=CARTESIAN_POINT('Ctrl Pts',(-2.20515487815661,3.43879495669882,-32.3136604550078));
#28333=CARTESIAN_POINT('Ctrl Pts',(-2.18139298917573,3.45391694238073,-32.3150397590708));
#28334=CARTESIAN_POINT('Ctrl Pts',(-2.15748640892605,3.46878615589076,-32.3164190631338));
#28335=CARTESIAN_POINT('Ctrl Pts',(-2.05651765328459,3.53158585245109,-32.3222445142623));
#28336=CARTESIAN_POINT('Ctrl Pts',(-1.9526431612848,3.59007388439192,-32.3280699653908));
#28337=CARTESIAN_POINT('Ctrl Pts',(-1.84626682834135,3.64397088333131,-32.3338954165193));
#28338=CARTESIAN_POINT('Ctrl Pts',(-1.74002401548954,3.69780023252157,-32.3397135557322));
#28339=CARTESIAN_POINT('Ctrl Pts',(-1.63128596846802,3.74704982764663,-32.3455316949451));
#28340=CARTESIAN_POINT('Ctrl Pts',(-1.52048469664809,3.79148404813458,-32.351349834158));
#28341=CARTESIAN_POINT('Ctrl Pts',(-1.409793676198,3.83587405492718,-32.3571621841068));
#28342=CARTESIAN_POINT('Ctrl Pts',(-1.29704389175103,3.87545806832089,-32.3629745340557));
#28343=CARTESIAN_POINT('Ctrl Pts',(-1.18269050645048,3.91004707976156,-32.3687868840046));
#28344=CARTESIAN_POINT('Ctrl Pts',(-1.06447467210484,3.94580438450512,-32.3747955543811));
#28345=CARTESIAN_POINT('Ctrl Pts',(-0.944545387756902,3.97622308711449,
-32.3808042247577));
#28346=CARTESIAN_POINT('Ctrl Pts',(-0.823426741796678,4.00114901008374,
-32.3868128951342));
#28347=CARTESIAN_POINT('Ctrl Pts',(-0.706395883563465,4.02523367627382,
-32.3926187712273));
#28348=CARTESIAN_POINT('Ctrl Pts',(-0.588255082315933,4.04419025689563,
-32.3984246473204));
#28349=CARTESIAN_POINT('Ctrl Pts',(-0.469490321672897,4.05793097992751,
-32.4042305234135));
#28350=CARTESIAN_POINT('Ctrl Pts',(-0.350742769693217,4.07166971196918,
-32.4100355582522));
#28351=CARTESIAN_POINT('Ctrl Pts',(-0.231371843327783,4.08019404256848,
-32.415840593091));
#28352=CARTESIAN_POINT('Ctrl Pts',(-0.111870224996192,4.08346789539961,
-32.4216456279298));
#28353=CARTESIAN_POINT('Ctrl Pts',(0.00764222554980037,4.08674204498885,
-32.4274511889655));
#28354=CARTESIAN_POINT('Ctrl Pts',(0.127284983734767,4.08476475937415,-32.4332567500012));
#28355=CARTESIAN_POINT('Ctrl Pts',(0.246564419532909,4.07755208268642,-32.4390623110368));
#28356=CARTESIAN_POINT('Ctrl Pts',(0.365882762502919,4.0703370533312,-32.4448697657599));
#28357=CARTESIAN_POINT('Ctrl Pts',(0.484837140335601,4.0578832612336,-32.4506772204829));
#28358=CARTESIAN_POINT('Ctrl Pts',(0.602938737191007,4.04025864013611,-32.456484675206));
#28359=CARTESIAN_POINT('Ctrl Pts',(0.721170510883805,4.02261459239669,-32.4622985311642));
#28360=CARTESIAN_POINT('Ctrl Pts',(0.838547223601299,3.99978839941529,-32.4681123871223));
#28361=CARTESIAN_POINT('Ctrl Pts',(0.954589798932851,3.97189920765537,-32.4739262430805));
#28362=CARTESIAN_POINT('Ctrl Pts',(1.07070872142917,3.94399166693419,-32.4797439241125));
#28363=CARTESIAN_POINT('Ctrl Pts',(1.18549136719503,3.9110146058307,-32.4855616051445));
#28364=CARTESIAN_POINT('Ctrl Pts',(1.29847495825567,3.87313668526983,-32.4913792861765));
#28365=CARTESIAN_POINT('Ctrl Pts',(1.41161864663505,3.83520509183961,-32.4972052108404));
#28366=CARTESIAN_POINT('Ctrl Pts',(1.52295781293906,3.7923589246507,-32.5030311355043));
#28367=CARTESIAN_POINT('Ctrl Pts',(1.63205062850394,3.74481451423163,-32.5088570601682));
#28368=CARTESIAN_POINT('Ctrl Pts',(1.65787866393587,3.73355823937489,-32.5102363644594));
#28369=CARTESIAN_POINT('Ctrl Pts',(1.68358090163677,3.72203881844289,-32.5116156687505));
#28370=CARTESIAN_POINT('Ctrl Pts',(1.7091516998568,3.71025948780899,-32.5129949730417));
#28371=CARTESIAN_POINT('Ctrl Pts',(1.81715610775104,3.66050665570897,-32.5188207959976));
#28372=CARTESIAN_POINT('Ctrl Pts',(1.92315906681105,3.60595435836731,-32.5246466189536));
#28373=CARTESIAN_POINT('Ctrl Pts',(2.02670496799447,3.54678614702191,-32.5304724419095));
#28374=CARTESIAN_POINT('Ctrl Pts',(2.13010585702929,3.48770079853596,-32.5362901060191));
#28375=CARTESIAN_POINT('Ctrl Pts',(2.23105618476815,3.424012601285,-32.5421077701286));
#28376=CARTESIAN_POINT('Ctrl Pts',(2.32912159384625,3.3559525624,-32.5479254342381));
#28377=CARTESIAN_POINT('Ctrl Pts',(2.38264847979213,3.31880345984571,-32.5511008805672));
#28378=CARTESIAN_POINT('Ctrl Pts',(2.43531623718868,3.2803526898498,-32.5542763268962));
#28379=CARTESIAN_POINT('Ctrl Pts',(2.48705727606861,3.24064362520074,-32.5574517732253));
#28380=CARTESIAN_POINT('',(-4.08499951611116,-0.00198830873281907,-32.010384971366));
#28381=CARTESIAN_POINT('Ctrl Pts',(-4.08499951611154,-0.00198830793933937,
-32.0103849714045));
#28382=CARTESIAN_POINT('Ctrl Pts',(-4.08505857983268,0.119358726635596,
-32.0162687995861));
#28383=CARTESIAN_POINT('Ctrl Pts',(-4.07970628193321,0.240701121345341,
-32.0221526277676));
#28384=CARTESIAN_POINT('Ctrl Pts',(-4.06897033272945,0.361532061327329,
-32.0280364559492));
#28385=CARTESIAN_POINT('Ctrl Pts',(-4.05823134250943,0.482397227333078,
-32.0339219507573));
#28386=CARTESIAN_POINT('Ctrl Pts',(-4.0421056992771,0.602750259327652,-32.0398074455653));
#28387=CARTESIAN_POINT('Ctrl Pts',(-4.02067294073167,0.72209009387204,-32.0456929403733));
#28388=CARTESIAN_POINT('Ctrl Pts',(-3.99922962856903,0.84148869205761,-32.0515813332339));
#28389=CARTESIAN_POINT('Ctrl Pts',(-3.97247406722256,0.959872713557851,
-32.0574697260944));
#28390=CARTESIAN_POINT('Ctrl Pts',(-3.94053669152283,1.07675233120822,-32.0633581189549));
#28391=CARTESIAN_POINT('Ctrl Pts',(-3.90855498480322,1.19379418487639,-32.0692546852629));
#28392=CARTESIAN_POINT('Ctrl Pts',(-3.87137720107183,1.3093270849135,-32.0751512515708));
#28393=CARTESIAN_POINT('Ctrl Pts',(-3.82918353551356,1.42287682226955,-32.0810478178788));
#28394=CARTESIAN_POINT('Ctrl Pts',(-3.78695819284858,1.53651180766219,-32.0869488110635));
#28395=CARTESIAN_POINT('Ctrl Pts',(-3.73970961600701,1.64816030227053,-32.0928498042483));
#28396=CARTESIAN_POINT('Ctrl Pts',(-3.68766529048739,1.75737011051586,-32.098750797433));
#28397=CARTESIAN_POINT('Ctrl Pts',(-3.63552985940311,1.86677109467034,-32.1046621205301));
#28398=CARTESIAN_POINT('Ctrl Pts',(-3.57858209089098,1.9737245171403,-32.1105734436271));
#28399=CARTESIAN_POINT('Ctrl Pts',(-3.51709471612082,2.07780407108924,-32.1164847667241));
#28400=CARTESIAN_POINT('Ctrl Pts',(-3.47684270541128,2.14593856757502,-32.1203545471709));
#28401=CARTESIAN_POINT('Ctrl Pts',(-3.43464613454845,2.21284205347598,-32.1242243276177));
#28402=CARTESIAN_POINT('Ctrl Pts',(-3.39059098493886,2.27840246068409,-32.1280941080644));
#28403=CARTESIAN_POINT('Ctrl Pts',(-3.32427168755066,2.37709512615128,-32.1339195591763));
#28404=CARTESIAN_POINT('Ctrl Pts',(-3.25353363423184,2.47304765452436,-32.1397450102882));
#28405=CARTESIAN_POINT('Ctrl Pts',(-3.17863056473336,2.56583957661871,-32.1455704614));
#28406=CARTESIAN_POINT('Ctrl Pts',(-3.10382151111628,2.65851502932935,-32.1513886005963));
#28407=CARTESIAN_POINT('Ctrl Pts',(-3.02485809354326,2.74803745164358,-32.1572067397926));
#28408=CARTESIAN_POINT('Ctrl Pts',(-2.94203763787773,2.8340147383722,-32.1630248789889));
#28409=CARTESIAN_POINT('Ctrl Pts',(-2.85929959163333,2.91990647451585,-32.1688372289212));
#28410=CARTESIAN_POINT('Ctrl Pts',(-2.77271242393837,3.00225980063408,-32.1746495788534));
#28411=CARTESIAN_POINT('Ctrl Pts',(-2.68261369815691,3.08071562245867,-32.1804619287857));
#28412=CARTESIAN_POINT('Ctrl Pts',(-2.58947175876295,3.16182140212545,-32.1864705991685));
#28413=CARTESIAN_POINT('Ctrl Pts',(-2.492577125476,3.23876138386672,-32.1924792695512));
#28414=CARTESIAN_POINT('Ctrl Pts',(-2.39234450899972,3.31117996343582,-32.198487939934));
#28415=CARTESIAN_POINT('Ctrl Pts',(-2.29549477136494,3.38115439568874,-32.2042938160107));
#28416=CARTESIAN_POINT('Ctrl Pts',(-2.19552908759903,3.44690744019488,-32.2100996920874));
#28417=CARTESIAN_POINT('Ctrl Pts',(-2.09285465911595,3.50815968505093,-32.2159055681641));
#28418=CARTESIAN_POINT('Ctrl Pts',(-1.99019510785271,3.56940305463857,-32.2217106029866));
#28419=CARTESIAN_POINT('Ctrl Pts',(-1.88482794274692,3.62614671256697,-32.2275156378091));
#28420=CARTESIAN_POINT('Ctrl Pts',(-1.7771876815604,3.67815564441065,-32.2333206726316));
#28421=CARTESIAN_POINT('Ctrl Pts',(-1.66953766332881,3.73016929060087,-32.2391262336512));
#28422=CARTESIAN_POINT('Ctrl Pts',(-1.5596145067462,3.77744717987937,-32.2449317946707));
#28423=CARTESIAN_POINT('Ctrl Pts',(-1.44787497518768,3.81980144198953,-32.2507373556902));
#28424=CARTESIAN_POINT('Ctrl Pts',(-1.33609899585901,3.86216951942886,-32.2565448103973));
#28425=CARTESIAN_POINT('Ctrl Pts',(-1.22250584456867,3.89961063112266,-32.2623522651043));
#28426=CARTESIAN_POINT('Ctrl Pts',(-1.10756918095594,3.93198620412084,-32.2681597198113));
#28427=CARTESIAN_POINT('Ctrl Pts',(-0.99250582902963,3.96439746291862,-32.2739735757538));
#28428=CARTESIAN_POINT('Ctrl Pts',(-0.876096401827009,3.99173192748857,
-32.2797874316963));
#28429=CARTESIAN_POINT('Ctrl Pts',(-0.758826685837961,4.01390172536152,
-32.2856012876387));
#28430=CARTESIAN_POINT('Ctrl Pts',(-0.641479815316192,4.03608610927128,
-32.2914189686552));
#28431=CARTESIAN_POINT('Ctrl Pts',(-0.523271931688789,4.0530990012752,-32.2972366496716));
#28432=CARTESIAN_POINT('Ctrl Pts',(-0.404694269923536,4.0649043713095,-32.303054330688));
#28433=CARTESIAN_POINT('Ctrl Pts',(-0.285948584055017,4.07672646950898,
-32.3088802553367));
#28434=CARTESIAN_POINT('Ctrl Pts',(-0.166832480162451,4.08332629566224,
-32.3147061799854));
#28435=CARTESIAN_POINT('Ctrl Pts',(-0.0478376433608585,4.08471988756606,
-32.3205321046341));
#28436=CARTESIAN_POINT('Ctrl Pts',(-0.0196652729037597,4.08504982446446,
-32.3219114090801));
#28437=CARTESIAN_POINT('Ctrl Pts',(0.00850032292552177,4.08508817077907,
-32.3232907135262));
#28438=CARTESIAN_POINT('Ctrl Pts',(0.0366526712919777,4.08483556360439,
-32.3246700179722));
#28439=CARTESIAN_POINT('Ctrl Pts',(0.155532688907448,4.08376886945208,-32.3304944605626));
#28440=CARTESIAN_POINT('Ctrl Pts',(0.274556241674694,4.0775065597022,-32.3363189031529));
#28441=CARTESIAN_POINT('Ctrl Pts',(0.393232873428394,4.06602913261271,-32.3421433457433));
#28442=CARTESIAN_POINT('Ctrl Pts',(0.511770058277997,4.0545651916801,-32.3479609445222));
#28443=CARTESIAN_POINT('Ctrl Pts',(0.629960730346802,4.03789835645692,-32.3537785433011));
#28444=CARTESIAN_POINT('Ctrl Pts',(0.747314013723899,4.01606110074185,-32.35959614208));
#28445=CARTESIAN_POINT('Ctrl Pts',(0.864557058872457,3.9942443583036,-32.3654082759775));
#28446=CARTESIAN_POINT('Ctrl Pts',(0.98096388104933,3.96726692908919,-32.371220409875));
#28447=CARTESIAN_POINT('Ctrl Pts',(1.09604894154684,3.93521304604135,-32.3770325437724));
#28448=CARTESIAN_POINT('Ctrl Pts',(1.21105300878,3.90318172151337,-32.3828405872719));
#28449=CARTESIAN_POINT('Ctrl Pts',(1.32473677325709,3.86608115981677,-32.3886486307714));
#28450=CARTESIAN_POINT('Ctrl Pts',(1.43662573038736,3.82404648386875,-32.3944566742709));
#28451=CARTESIAN_POINT('Ctrl Pts',(1.54847062998495,3.78202835954618,-32.4002624307881));
#28452=CARTESIAN_POINT('Ctrl Pts',(1.65852174623152,3.73508012760712,-32.4060681873053));
#28453=CARTESIAN_POINT('Ctrl Pts',(1.76632106908059,3.68338633337884,-32.4118739438224));
#28454=CARTESIAN_POINT('Ctrl Pts',(1.87409602925729,3.63170422196024,-32.4176783882373));
#28455=CARTESIAN_POINT('Ctrl Pts',(1.97961984251812,3.57527886181049,-32.4234828326521));
#28456=CARTESIAN_POINT('Ctrl Pts',(2.08245644740712,3.5143420642636,-32.4292872770669));
#28457=CARTESIAN_POINT('Ctrl Pts',(2.18531388380867,3.45339292280799,-32.4350928972825));
#28458=CARTESIAN_POINT('Ctrl Pts',(2.28548267412948,3.38793072753696,-32.4408985174981));
#28459=CARTESIAN_POINT('Ctrl Pts',(2.38255355088111,3.31823199568442,-32.4467041377137));
#28460=CARTESIAN_POINT('Ctrl Pts',(2.41780252834394,3.29292256086244,-32.4488123104529));
#28461=CARTESIAN_POINT('Ctrl Pts',(2.45264329664656,3.2670549026564,-32.4509204831921));
#28462=CARTESIAN_POINT('Ctrl Pts',(2.48705727606859,3.24064362520075,-32.4530286559312));
#28463=CARTESIAN_POINT('Ctrl Pts',(2.48705727606859,3.24064362520075,-31.2032093449099));
#28464=CARTESIAN_POINT('Ctrl Pts',(2.58179338776476,3.16793765590868,-31.209016651121));
#28465=CARTESIAN_POINT('Ctrl Pts',(2.67340003593691,3.09102689829715,-31.2148239573321));
#28466=CARTESIAN_POINT('Ctrl Pts',(2.76148917095052,3.01021636410458,-31.2206312635432));
#28467=CARTESIAN_POINT('Ctrl Pts',(2.84955077592288,2.92943108520984,-31.2264367548269));
#28468=CARTESIAN_POINT('Ctrl Pts',(2.93409675328447,2.84474872873737,-31.2322422461106));
#28469=CARTESIAN_POINT('Ctrl Pts',(3.01477311734607,2.75651374945373,-31.2380477373943));
#28470=CARTESIAN_POINT('Ctrl Pts',(3.09544327087232,2.66828556257409,-31.2438527817664));
#28471=CARTESIAN_POINT('Ctrl Pts',(3.17224412831572,2.57650559795978,-31.2496578261384));
#28472=CARTESIAN_POINT('Ctrl Pts',(3.24485992657571,2.48155375861638,-31.2554628705105));
#28473=CARTESIAN_POINT('Ctrl Pts',(3.31748723886432,2.38658686362088,-31.2612688353358));
#28474=CARTESIAN_POINT('Ctrl Pts',(3.38592792457097,2.28844741789956,-31.2670748001611));
#28475=CARTESIAN_POINT('Ctrl Pts',(3.44990812167822,2.18754633139019,-31.2728807649864));
#28476=CARTESIAN_POINT('Ctrl Pts',(3.51395352814054,2.08654240532928,-31.278692647318));
#28477=CARTESIAN_POINT('Ctrl Pts',(3.57352914577614,1.98277156114108,-31.2845045296497));
#28478=CARTESIAN_POINT('Ctrl Pts',(3.62840574929162,1.87667171303548,-31.2903164119813));
#28479=CARTESIAN_POINT('Ctrl Pts',(3.68331020688576,1.77051801113196,-31.2961312442883));
#28480=CARTESIAN_POINT('Ctrl Pts',(3.73351072648581,1.66203332015816,-31.3019460765953));
#28481=CARTESIAN_POINT('Ctrl Pts',(3.77882589874646,1.55167645692102,-31.3077609089023));
#28482=CARTESIAN_POINT('Ctrl Pts',(3.82421427666205,1.44114131462091,-31.3135851349418));
#28483=CARTESIAN_POINT('Ctrl Pts',(3.86470139769733,1.32872834058064,-31.3194093609813));
#28484=CARTESIAN_POINT('Ctrl Pts',(3.90015528637214,1.2149130595164,-31.3252335870208));
#28485=CARTESIAN_POINT('Ctrl Pts',(3.93375092788814,1.10706318677746,-31.3307525474915));
#28486=CARTESIAN_POINT('Ctrl Pts',(3.96282747733818,0.99795455533443,-31.3362715079623));
#28487=CARTESIAN_POINT('Ctrl Pts',(3.9873152681288,0.887998847154075,-31.3417904684331));
#28488=CARTESIAN_POINT('Ctrl Pts',(4.01316297123626,0.771936825703536,-31.3476159205096));
#28489=CARTESIAN_POINT('Ctrl Pts',(4.03398035212741,0.654559649078143,-31.3534413725861));
#28490=CARTESIAN_POINT('Ctrl Pts',(4.04963744446642,0.536340906863787,-31.3592668246626));
#28491=CARTESIAN_POINT('Ctrl Pts',(4.06527488456825,0.418270548698773,-31.3650849648345));
#28492=CARTESIAN_POINT('Ctrl Pts',(4.07576486590849,0.299361126921743,-31.3709031050064));
#28493=CARTESIAN_POINT('Ctrl Pts',(4.08102800875816,0.180098283532682,-31.3767212451783));
#28494=CARTESIAN_POINT('Ctrl Pts',(4.08628591459541,0.0609541108712847,
-31.3825335960959));
#28495=CARTESIAN_POINT('Ctrl Pts',(4.08632731079461,-0.0585423784766985,
-31.3883459470134));
#28496=CARTESIAN_POINT('Ctrl Pts',(4.08112446558333,-0.177899118652157,
-31.394158297931));
#28497=CARTESIAN_POINT('Ctrl Pts',(4.0757458880563,-0.30128727538888,-31.4001669679481));
#28498=CARTESIAN_POINT('Ctrl Pts',(4.06476247903152,-0.424525635170655,
-31.4061756379652));
#28499=CARTESIAN_POINT('Ctrl Pts',(4.04820218464763,-0.547068617464195,
-31.4121843079823));
#28500=CARTESIAN_POINT('Ctrl Pts',(4.03220080109268,-0.665475767493723,
-31.4179901850621));
#28501=CARTESIAN_POINT('Ctrl Pts',(4.01099295722774,-0.783233284119383,
-31.4237960621419));
#28502=CARTESIAN_POINT('Ctrl Pts',(3.98465665307939,-0.899853519785383,
-31.4296019392217));
#28503=CARTESIAN_POINT('Ctrl Pts',(3.95832416496072,-1.01645685762555,-31.4354069750522));
#28504=CARTESIAN_POINT('Ctrl Pts',(3.92686478424874,-1.13192284433952,-31.4412120108826));
#28505=CARTESIAN_POINT('Ctrl Pts',(3.89040751072223,-1.24577461866745,-31.4470170467131));
#28506=CARTESIAN_POINT('Ctrl Pts',(3.85394693250546,-1.35963671315413,-31.4528226087443));
#28507=CARTESIAN_POINT('Ctrl Pts',(3.81248768516331,-1.47188391573622,-31.4586281707755));
#28508=CARTESIAN_POINT('Ctrl Pts',(3.76620826581264,-1.58205571915927,-31.4644337328067));
#28509=CARTESIAN_POINT('Ctrl Pts',(3.71991375078668,-1.69226345902648,-31.470241188528));
#28510=CARTESIAN_POINT('Ctrl Pts',(3.66879609475868,-1.80039407741151,-31.4760486442494));
#28511=CARTESIAN_POINT('Ctrl Pts',(3.61308116759669,-1.90600878181559,-31.4818560999707));
#28512=CARTESIAN_POINT('Ctrl Pts',(3.55730482898067,-2.01173989941258,-31.4876699569263));
#28513=CARTESIAN_POINT('Ctrl Pts',(3.4969212951177,-2.11494920661366,-31.4934838138819));
#28514=CARTESIAN_POINT('Ctrl Pts',(3.43220153996603,-2.21522404940331,-31.4992976708375));
#28515=CARTESIAN_POINT('Ctrl Pts',(3.36743920415105,-2.31556486539249,-31.5051153528676));
#28516=CARTESIAN_POINT('Ctrl Pts',(3.29833520087221,-2.41296703997161,-31.5109330348977));
#28517=CARTESIAN_POINT('Ctrl Pts',(3.2252018350368,-2.50704968504321,-31.5167507169277));
#28518=CARTESIAN_POINT('Ctrl Pts',(3.15196483960127,-2.60126564473496,-31.5225766425831));
#28519=CARTESIAN_POINT('Ctrl Pts',(3.07468734935894,-2.69215237714021,-31.5284025682385));
#28520=CARTESIAN_POINT('Ctrl Pts',(2.99371972014326,-2.7793645383838,-31.5342284938938));
#28521=CARTESIAN_POINT('Ctrl Pts',(2.97455053779819,-2.80001212110025,-31.5356077887095));
#28522=CARTESIAN_POINT('Ctrl Pts',(2.95517466932275,-2.82045391404605,-31.5369870835252));
#28523=CARTESIAN_POINT('Ctrl Pts',(2.93559703565821,-2.84068566445404,-31.5383663783409));
#28524=CARTESIAN_POINT('Ctrl Pts',(2.85291090821357,-2.92613445368613,-31.5441918294076));
#28525=CARTESIAN_POINT('Ctrl Pts',(2.76635857277787,-3.00810672305135,-31.5500172804743));
#28526=CARTESIAN_POINT('Ctrl Pts',(2.67626394974318,-3.08623334686557,-31.555842731541));
#28527=CARTESIAN_POINT('Ctrl Pts',(2.58628241051181,-3.16426190871488,-31.5616608706934));
#28528=CARTESIAN_POINT('Ctrl Pts',(2.49276773275701,-3.23845416086974,-31.5674790098458));
#28529=CARTESIAN_POINT('Ctrl Pts',(2.39608173715407,-3.30847658430232,-31.5732971489982));
#28530=CARTESIAN_POINT('Ctrl Pts',(2.2994919476763,-3.37842933284566,-31.5791094988879));
#28531=CARTESIAN_POINT('Ctrl Pts',(2.19973744669917,-3.44422026905515,-31.5849218487777));
#28532=CARTESIAN_POINT('Ctrl Pts',(2.09721383948261,-3.50555546404312,-31.5907341986674));
#28533=CARTESIAN_POINT('Ctrl Pts',(1.99122734940714,-3.56896234379852,-31.5967428690666));
#28534=CARTESIAN_POINT('Ctrl Pts',(1.88228171634488,-3.6276068652051,-31.6027515394658));
#28535=CARTESIAN_POINT('Ctrl Pts',(1.77084786800124,-3.68121214118331,-31.6087602098651));
#28536=CARTESIAN_POINT('Ctrl Pts',(1.6631749442234,-3.73300822361506,-31.6145660859029));
#28537=CARTESIAN_POINT('Ctrl Pts',(1.55317944793754,-3.7800995328266,-31.6203719619407));
#28538=CARTESIAN_POINT('Ctrl Pts',(1.44131147719164,-3.82228285527323,-31.6261778379786));
#28539=CARTESIAN_POINT('Ctrl Pts',(1.32945971575516,-3.86446006549201,-31.6319828727636));
#28540=CARTESIAN_POINT('Ctrl Pts',(1.21573640111529,-3.90173055933158,-31.6377879075487));
#28541=CARTESIAN_POINT('Ctrl Pts',(1.10061068905402,-3.93393964253902,-31.6435929423337));
#28542=CARTESIAN_POINT('Ctrl Pts',(0.985474541399795,-3.96615164534518,
-31.6493985033173));
#28543=CARTESIAN_POINT('Ctrl Pts',(0.868936136523122,-3.99330121539376,
-31.6552040643009));
#28544=CARTESIAN_POINT('Ctrl Pts',(0.751478212259808,-4.01528398702991,
-31.6610096252845));
#28545=CARTESIAN_POINT('Ctrl Pts',(0.633981974941117,-4.03727392912434,
-31.6668170799571));
#28546=CARTESIAN_POINT('Ctrl Pts',(0.515566022569239,-4.05409364599779,
-31.6726245346297));
#28547=CARTESIAN_POINT('Ctrl Pts',(0.396721029792019,-4.06569027651157,
-31.6784319893022));
#28548=CARTESIAN_POINT('Ctrl Pts',(0.277745040715636,-4.07729968935337,
-31.6842458452127));
#28549=CARTESIAN_POINT('Ctrl Pts',(0.158339473599013,-4.08367448471301,
-31.6900597011232));
#28550=CARTESIAN_POINT('Ctrl Pts',(0.0389979977760629,-4.08481384596281,
-31.6958735570336));
#28551=CARTESIAN_POINT('Ctrl Pts',(-0.0804219956687229,-4.08595395682572,
-31.7016912380195));
#28552=CARTESIAN_POINT('Ctrl Pts',(-0.199777407019994,-4.0818517876119,
-31.7075089190053));
#28553=CARTESIAN_POINT('Ctrl Pts',(-0.318578347341432,-4.07255851236114,
-31.7133265999911));
#28554=CARTESIAN_POINT('Ctrl Pts',(-0.437547628198452,-4.06325206857039,
-31.7191525246115));
#28555=CARTESIAN_POINT('Ctrl Pts',(-0.555960466404257,-4.04873988702924,
-31.7249784492319));
#28556=CARTESIAN_POINT('Ctrl Pts',(-0.673335713159881,-4.02912447280839,
-31.7308043738522));
#28557=CARTESIAN_POINT('Ctrl Pts',(-0.701124648250158,-4.02448046576585,
-31.7321836786511));
#28558=CARTESIAN_POINT('Ctrl Pts',(-0.728855486948905,-4.01955063384845,
-31.7335629834499));
#28559=CARTESIAN_POINT('Ctrl Pts',(-0.756521970249876,-4.01433674578121,
-31.7349422882488));
#28560=CARTESIAN_POINT('Ctrl Pts',(-0.873370502116339,-3.99231605166746,
-31.7407677391739));
#28561=CARTESIAN_POINT('Ctrl Pts',(-0.989443698158363,-3.96515409256765,
-31.7465931900991));
#28562=CARTESIAN_POINT('Ctrl Pts',(-1.1042550989485,-3.93291821380082,-31.7524186410243));
#28563=CARTESIAN_POINT('Ctrl Pts',(-1.21892239215086,-3.90072279647508,
-31.7582367800303));
#28564=CARTESIAN_POINT('Ctrl Pts',(-1.33233065082415,-3.86346623611826,
-31.7640549190363));
#28565=CARTESIAN_POINT('Ctrl Pts',(-1.44400229069796,-3.82126711765339,
-31.7698730580423));
#28566=CARTESIAN_POINT('Ctrl Pts',(-1.55556281308672,-3.77910998889978,
-31.775685407781));
#28567=CARTESIAN_POINT('Ctrl Pts',(-1.66538977487724,-3.7320202294698,-31.7814977575197));
#28568=CARTESIAN_POINT('Ctrl Pts',(-1.77302005787152,-3.68016641938721,
-31.7873101072584));
#28569=CARTESIAN_POINT('Ctrl Pts',(-1.88428571297945,-3.62656117011932,
-31.7933187777125));
#28570=CARTESIAN_POINT('Ctrl Pts',(-1.99320324284419,-3.56786446788854,
-31.7993274481666));
#28571=CARTESIAN_POINT('Ctrl Pts',(-2.09928231045757,-3.50431716330014,
-31.8053361186207));
#28572=CARTESIAN_POINT('Ctrl Pts',(-2.20178117511103,-3.44291460086588,
-31.8111419944968));
#28573=CARTESIAN_POINT('Ctrl Pts',(-2.30162970595371,-3.37698379793955,
-31.816947870373));
#28574=CARTESIAN_POINT('Ctrl Pts',(-2.39841054414801,-3.30678875371858,
-31.8227537462491));
#28575=CARTESIAN_POINT('Ctrl Pts',(-2.49517735904853,-3.23660388057842,
-31.8285587808688));
#28576=CARTESIAN_POINT('Ctrl Pts',(-2.58887703510446,-3.16215623444704,
-31.8343638154885));
#28577=CARTESIAN_POINT('Ctrl Pts',(-2.67912223909719,-3.0837524265049,-31.8401688501082));
#28578=CARTESIAN_POINT('Ctrl Pts',(-2.76937562332888,-3.00534151168222,
-31.8459744109229));
#28579=CARTESIAN_POINT('Ctrl Pts',(-2.85617360489777,-2.92297398966321,
-31.8517799717376));
#28580=CARTESIAN_POINT('Ctrl Pts',(-2.93916340009146,-2.83699550714534,
-31.8575855325522));
#28581=CARTESIAN_POINT('Ctrl Pts',(-3.02218026529552,-2.75098897975269,
-31.8633929870526));
#28582=CARTESIAN_POINT('Ctrl Pts',(-3.10138619047977,-2.66136944278746,
-31.869200441553));
#28583=CARTESIAN_POINT('Ctrl Pts',(-3.17646702976446,-2.56851751187711,
-31.8750078960534));
#28584=CARTESIAN_POINT('Ctrl Pts',(-3.25163062647782,-2.47556323545327,
-31.8808217517875));
#28585=CARTESIAN_POINT('Ctrl Pts',(-3.32265980487839,-2.37936977084228,
-31.8866356075217));
#28586=CARTESIAN_POINT('Ctrl Pts',(-3.38928222735186,-2.28034887316762,
-31.8924494632558));
#28587=CARTESIAN_POINT('Ctrl Pts',(-3.45594848228769,-2.18126282730998,
-31.8982671440627));
#28588=CARTESIAN_POINT('Ctrl Pts',(-3.51820199497138,-2.07934599100962,
-31.9040848248696));
#28589=CARTESIAN_POINT('Ctrl Pts',(-3.57581591928054,-1.975035572191,-31.9099025056765));
#28590=CARTESIAN_POINT('Ctrl Pts',(-3.63351148230604,-1.8705773458971,-31.9157284301154));
#28591=CARTESIAN_POINT('Ctrl Pts',(-3.68655415481689,-1.76371913183232,
-31.9215543545543));
#28592=CARTESIAN_POINT('Ctrl Pts',(-3.7347647606383,-1.65491908644935,-31.9273802789933));
#28593=CARTESIAN_POINT('Ctrl Pts',(-3.74617877694831,-1.62916032504463,
-31.928759585381));
#28594=CARTESIAN_POINT('Ctrl Pts',(-3.7573221650775,-1.60329278941273,-31.9301388917688));
#28595=CARTESIAN_POINT('Ctrl Pts',(-3.76819295767263,-1.57732267901859,
-31.9315181981565));
#28596=CARTESIAN_POINT('Ctrl Pts',(-3.8199909931333,-1.4535781877737,-31.9380904292573));
#28597=CARTESIAN_POINT('Ctrl Pts',(-3.86573903894072,-1.3271614817197,-31.9446626603581));
#28598=CARTESIAN_POINT('Ctrl Pts',(-3.90518392162653,-1.19865071570898,
-31.9512348914589));
#28599=CARTESIAN_POINT('Ctrl Pts',(-3.94380032604224,-1.07283911800259,
-31.9576690830909));
#28600=CARTESIAN_POINT('Ctrl Pts',(-3.97637557280735,-0.945020799958586,
-31.9641032747229));
#28601=CARTESIAN_POINT('Ctrl Pts',(-4.00271890358611,-0.815761226630919,
-31.9705374663549));
#28602=CARTESIAN_POINT('Ctrl Pts',(-4.02990999106734,-0.682341941284823,
-31.97717871719));
#28603=CARTESIAN_POINT('Ctrl Pts',(-4.05046116507769,-0.547387282983328,
-31.9838199680252));
#28604=CARTESIAN_POINT('Ctrl Pts',(-4.06421691951732,-0.411540801269059,
-31.9904612188604));
#28605=CARTESIAN_POINT('Ctrl Pts',(-4.07797267395695,-0.275694319554789,
-31.9971024696956));
#28606=CARTESIAN_POINT('Ctrl Pts',(-4.08493284911617,-0.138956294514414,
-32.0037437205308));
#28607=CARTESIAN_POINT('Ctrl Pts',(-4.08499951611116,-0.00198830873280959,
-32.010384971366));
#28608=CARTESIAN_POINT('Origin',(0.,0.,-25.2396150285955));
#28609=CARTESIAN_POINT('',(2.4870572760686,3.24064362520075,-29.953048263356));
#28610=CARTESIAN_POINT('',(2.48705727606859,3.24064362520075,-30.0573351590495));
#28611=CARTESIAN_POINT('',(2.4870572760686,3.24064362520075,-25.2396150285955));
#28612=CARTESIAN_POINT('',(-4.08499937550907,0.002258780766463,-30.8646150286367));
#28613=CARTESIAN_POINT('Ctrl Pts',(2.48705727606859,3.24064362520075,-30.0573351590495));
#28614=CARTESIAN_POINT('Ctrl Pts',(2.5819015155267,3.16785467241275,-30.0631404188983));
#28615=CARTESIAN_POINT('Ctrl Pts',(2.67354511593237,3.09090048087354,-30.0689456787472));
#28616=CARTESIAN_POINT('Ctrl Pts',(2.76161314187302,3.01010263191045,-30.074750938596));
#28617=CARTESIAN_POINT('Ctrl Pts',(2.8497034648523,2.92928432657014,-30.0805576682189));
#28618=CARTESIAN_POINT('Ctrl Pts',(2.93421611250136,2.84462070430025,-30.0863643978418));
#28619=CARTESIAN_POINT('Ctrl Pts',(3.0148123336213,2.75647085837034,-30.0921711274647));
#28620=CARTESIAN_POINT('Ctrl Pts',(3.09549460057924,2.66822690222957,-30.0979840564467));
#28621=CARTESIAN_POINT('Ctrl Pts',(3.17225181671804,2.57648959232832,-30.1037969854287));
#28622=CARTESIAN_POINT('Ctrl Pts',(3.24478480929274,2.48165197829653,-30.1096099144107));
#28623=CARTESIAN_POINT('Ctrl Pts',(3.31736077328321,2.38675817870836,-30.1154262872019));
#28624=CARTESIAN_POINT('Ctrl Pts',(3.38570729559298,2.28876075060164,-30.1212426599931));
#28625=CARTESIAN_POINT('Ctrl Pts',(3.44956888102454,2.18808124507915,-30.1270590327844));
#28626=CARTESIAN_POINT('Ctrl Pts',(3.51352628694766,2.08725067597682,-30.1328841326953));
#28627=CARTESIAN_POINT('Ctrl Pts',(3.57298511452915,1.98373034625041,-30.1387092326062));
#28628=CARTESIAN_POINT('Ctrl Pts',(3.62773594424741,1.877966165514,-30.1445343325171));
#28629=CARTESIAN_POINT('Ctrl Pts',(3.65765561320019,1.8201692464357,-30.1477175730606));
#28630=CARTESIAN_POINT('Ctrl Pts',(3.68617017732957,1.76170260746799,-30.1509008136042));
#28631=CARTESIAN_POINT('Ctrl Pts',(3.71325165581724,1.70264122485347,-30.1540840541477));
#28632=CARTESIAN_POINT('Ctrl Pts',(3.76281166486531,1.59455692443023,-30.1599094905326));
#28633=CARTESIAN_POINT('Ctrl Pts',(3.80772791300253,1.48413404864421,-30.1657349269176));
#28634=CARTESIAN_POINT('Ctrl Pts',(3.84777421648458,1.37180850666428,-30.1715603633025));
#28635=CARTESIAN_POINT('Ctrl Pts',(3.88777025349365,1.25962395669434,-30.1773784875483));
#28636=CARTESIAN_POINT('Ctrl Pts',(3.92290836847849,1.14554187177275,-30.1831966117942));
#28637=CARTESIAN_POINT('Ctrl Pts',(3.95300932257877,1.03002053164261,-30.1890147360401));
#28638=CARTESIAN_POINT('Ctrl Pts',(3.98308032398347,0.914614143866526,-30.1948270708181));
#28639=CARTESIAN_POINT('Ctrl Pts',(4.00812403386335,0.797771742659466,-30.2006394055962));
#28640=CARTESIAN_POINT('Ctrl Pts',(4.02801037385384,0.679968696430837,-30.2064517403742));
#28641=CARTESIAN_POINT('Ctrl Pts',(4.04856847625628,0.558186252358891,-30.2124604163609));
#28642=CARTESIAN_POINT('Ctrl Pts',(4.06361445849569,0.435377531316219,-30.2184690923477));
#28643=CARTESIAN_POINT('Ctrl Pts',(4.07306148925245,0.312081887921398,-30.2244777683344));
#28644=CARTESIAN_POINT('Ctrl Pts',(4.08218964709338,0.192947937478719,-30.2302836288459));
#28645=CARTESIAN_POINT('Ctrl Pts',(4.08609069153235,0.0733598444011744,
-30.2360894893574));
#28646=CARTESIAN_POINT('Ctrl Pts',(4.08473886019349,-0.0461892197937499,
-30.2418953498689));
#28647=CARTESIAN_POINT('Ctrl Pts',(4.08338722476066,-0.165720959060078,
-30.2477003690011));
#28648=CARTESIAN_POINT('Ctrl Pts',(4.07678423208726,-0.285213272806567,
-30.2535053881332));
#28649=CARTESIAN_POINT('Ctrl Pts',(4.06495624755798,-0.404172865788039,
-30.2593104072653));
#28650=CARTESIAN_POINT('Ctrl Pts',(4.05312719109958,-0.523143239664004,
-30.2651159524862));
#28651=CARTESIAN_POINT('Ctrl Pts',(4.0360722416797,-0.641580390751066,-30.270921497707));
#28652=CARTESIAN_POINT('Ctrl Pts',(4.01386958827962,-0.758996658941261,
-30.2767270429278));
#28653=CARTESIAN_POINT('Ctrl Pts',(3.99165969303522,-0.876451224821353,
-30.2825344817446));
#28654=CARTESIAN_POINT('Ctrl Pts',(3.96429883033393,-0.992883844869048,
-30.2883419205614));
#28655=CARTESIAN_POINT('Ctrl Pts',(3.93191605687673,-1.10781818078371,-30.2941493593782));
#28656=CARTESIAN_POINT('Ctrl Pts',(3.89949758990046,-1.22287920167539,-30.2999631993739));
#28657=CARTESIAN_POINT('Ctrl Pts',(3.8620462740892,-1.33643824908993,-30.3057770393697));
#28658=CARTESIAN_POINT('Ctrl Pts',(3.81974074103337,-1.44803510706399,-30.3115908793655));
#28659=CARTESIAN_POINT('Ctrl Pts',(3.77740737445923,-1.55970538647885,-30.3174085443839));
#28660=CARTESIAN_POINT('Ctrl Pts',(3.73021359112887,-1.66941053150841,-30.3232262094023));
#28661=CARTESIAN_POINT('Ctrl Pts',(3.67838508536788,-1.77671274091879,-30.3290438744207));
#28662=CARTESIAN_POINT('Ctrl Pts',(3.62648313820408,-1.88416699840903,-30.3348697831164));
#28663=CARTESIAN_POINT('Ctrl Pts',(3.5699335535695,-1.98921116644357,-30.3406956918122));
#28664=CARTESIAN_POINT('Ctrl Pts',(3.50900667166786,-2.09143423950896,-30.346521600508));
#28665=CARTESIAN_POINT('Ctrl Pts',(3.49458044792067,-2.11563854601767,-30.3479010550238));
#28666=CARTESIAN_POINT('Ctrl Pts',(3.4799089969373,-2.13968482824368,-30.3492805095397));
#28667=CARTESIAN_POINT('Ctrl Pts',(3.4649962422784,-2.16356789609122,-30.3506599640555));
#28668=CARTESIAN_POINT('Ctrl Pts',(3.40201945063289,-2.26442645791249,-30.356485421633));
#28669=CARTESIAN_POINT('Ctrl Pts',(3.33453460157875,-2.36269440139011,-30.3623108792105));
#28670=CARTESIAN_POINT('Ctrl Pts',(3.26278121164091,-2.45794299465286,-30.368136336788));
#28671=CARTESIAN_POINT('Ctrl Pts',(3.19111788326781,-2.55307203624906,-30.3739544825183));
#28672=CARTESIAN_POINT('Ctrl Pts',(3.11519691389463,-2.64518894245019,-30.3797726282486));
#28673=CARTESIAN_POINT('Ctrl Pts',(3.03530233160536,-2.73389186979864,-30.3855907739789));
#28674=CARTESIAN_POINT('Ctrl Pts',(2.95548724647239,-2.82250653546177,-30.3914031305051));
#28675=CARTESIAN_POINT('Ctrl Pts',(2.87170668579596,-2.9077136788627,-30.3972154870313));
#28676=CARTESIAN_POINT('Ctrl Pts',(2.7842859981162,-2.98914310140784,-30.4030278435576));
#28677=CARTESIAN_POINT('Ctrl Pts',(2.69391269076265,-3.07332278960993,-30.4090365114911));
#28678=CARTESIAN_POINT('Ctrl Pts',(2.59964928194172,-3.15346470158736,-30.4150451794247));
#28679=CARTESIAN_POINT('Ctrl Pts',(2.50189833929529,-3.22919954475276,-30.4210538473583));
#28680=CARTESIAN_POINT('Ctrl Pts',(2.40744637079887,-3.30237843006147,-30.4268597301355));
#28681=CARTESIAN_POINT('Ctrl Pts',(2.30973881837302,-3.37144264327577,-30.4326656129127));
#28682=CARTESIAN_POINT('Ctrl Pts',(2.20917329806707,-3.4360992912178,-30.4384714956899));
#28683=CARTESIAN_POINT('Ctrl Pts',(2.10862234890972,-3.50074657092286,-30.4442765372407));
#28684=CARTESIAN_POINT('Ctrl Pts',(2.00521459852327,-3.56098733482191,-30.4500815787914));
#28685=CARTESIAN_POINT('Ctrl Pts',(1.89937645088224,-3.61657214746699,-30.4558866203421));
#28686=CARTESIAN_POINT('Ctrl Pts',(1.79352870918881,-3.67216199878307,-30.4616921881102));
#28687=CARTESIAN_POINT('Ctrl Pts',(1.68525049345233,-3.72309486997931,-30.4674977558783));
#28688=CARTESIAN_POINT('Ctrl Pts',(1.5749920196836,-3.7691676983033,-30.4733033236464));
#28689=CARTESIAN_POINT('Ctrl Pts',(1.46469758103843,-3.81525555498312,-30.479110785115));
#28690=CARTESIAN_POINT('Ctrl Pts',(1.35242197599852,-3.85648005875395,-30.4849182465836));
#28691=CARTESIAN_POINT('Ctrl Pts',(1.2386339583867,-3.89268685063817,-30.4907257080522));
#28692=CARTESIAN_POINT('Ctrl Pts',(1.12472051898372,-3.92893355112424,-30.4965395707415));
#28693=CARTESIAN_POINT('Ctrl Pts',(1.00929172853534,-3.96015137635691,-30.5023534334309));
#28694=CARTESIAN_POINT('Ctrl Pts',(0.892830158941835,-3.9862362332511,-30.5081672961202));
#28695=CARTESIAN_POINT('Ctrl Pts',(0.776291966619323,-4.01233825196895,
-30.5139849838828));
#28696=CARTESIAN_POINT('Ctrl Pts',(0.658720042652412,-4.03330050522126,
-30.5198026716453));
#28697=CARTESIAN_POINT('Ctrl Pts',(0.540604140656138,-4.04907053076449,
-30.5256203594078));
#28698=CARTESIAN_POINT('Ctrl Pts',(0.422320870117633,-4.06486290220816,
-30.5314462907506));
#28699=CARTESIAN_POINT('Ctrl Pts',(0.3034924880319,-4.07544832564865,-30.5372722220934));
#28700=CARTESIAN_POINT('Ctrl Pts',(0.184610941756973,-4.08082636241529,
-30.5430981534362));
#28701=CARTESIAN_POINT('Ctrl Pts',(0.156466736972135,-4.08209956732256,
-30.5444773936119));
#28702=CARTESIAN_POINT('Ctrl Pts',(0.128319537569869,-4.08308114553061,
-30.5458566337877));
#28703=CARTESIAN_POINT('Ctrl Pts',(0.100175833174998,-4.08377151692497,
-30.5472358739634));
#28704=CARTESIAN_POINT('Ctrl Pts',(-0.0186938050359793,-4.08668741586732,
-30.553061325311));
#28705=CARTESIAN_POINT('Ctrl Pts',(-0.137881017317987,-4.08441362222163,
-30.5588867766586));
#28706=CARTESIAN_POINT('Ctrl Pts',(-0.256896020854348,-4.07691420494339,
-30.5647122280062));
#28707=CARTESIAN_POINT('Ctrl Pts',(-0.375761641061523,-4.06942420066256,
-30.5705303674579));
#28708=CARTESIAN_POINT('Ctrl Pts',(-0.494455078778615,-4.05672164417915,
-30.5763485069096));
#28709=CARTESIAN_POINT('Ctrl Pts',(-0.612484508638743,-4.03882256687237,
-30.5821666463614));
#28710=CARTESIAN_POINT('Ctrl Pts',(-0.73039649524063,-4.02094129975041,
-30.5879789965684));
#28711=CARTESIAN_POINT('Ctrl Pts',(-0.847645387292645,-3.99787385934325,
-30.5937913467753));
#28712=CARTESIAN_POINT('Ctrl Pts',(-0.96374304443309,-3.96968819232781,
-30.5996036969823));
#28713=CARTESIAN_POINT('Ctrl Pts',(-1.08376205877522,-3.94055051584846,
-30.6056123672694));
#28714=CARTESIAN_POINT('Ctrl Pts',(-1.20255024929556,-3.90594277036763,
-30.6116210375564));
#28715=CARTESIAN_POINT('Ctrl Pts',(-1.31957773775598,-3.8659978781705,-30.6176297078434));
#28716=CARTESIAN_POINT('Ctrl Pts',(-1.43265552380764,-3.82740113450671,
-30.6234355842415));
#28717=CARTESIAN_POINT('Ctrl Pts',(-1.54408912124532,-3.7838218328427,-30.6292414606395));
#28718=CARTESIAN_POINT('Ctrl Pts',(-1.65341517088357,-3.73543080148623,
-30.6350473370375));
#28719=CARTESIAN_POINT('Ctrl Pts',(-1.7627253798184,-3.6870467817064,-30.6408523721981));
#28720=CARTESIAN_POINT('Ctrl Pts',(-1.86992827526061,-3.63385258388174,
-30.6466574073587));
#28721=CARTESIAN_POINT('Ctrl Pts',(-1.97458094298633,-3.57606698757101,
-30.6524624425193));
#28722=CARTESIAN_POINT('Ctrl Pts',(-2.0792430972436,-3.51827615312451,-30.6582680038934));
#28723=CARTESIAN_POINT('Ctrl Pts',(-2.18135420695917,-3.455893289919,-30.6640735652675));
#28724=CARTESIAN_POINT('Ctrl Pts',(-2.28049697495161,-3.38918257803214,
-30.6698791266416));
#28725=CARTESIAN_POINT('Ctrl Pts',(-2.37967208211172,-3.32245010592069,
-30.6756865817194));
#28726=CARTESIAN_POINT('Ctrl Pts',(-2.47587658358236,-3.25138720521719,
-30.6814940367971));
#28727=CARTESIAN_POINT('Ctrl Pts',(-2.56872364793758,-3.17630033537861,
-30.6873014918749));
#28728=CARTESIAN_POINT('Ctrl Pts',(-2.66167305281528,-3.10113070116245,
-30.6931153482104));
#28729=CARTESIAN_POINT('Ctrl Pts',(-2.75125731632493,-3.0219285012329,-30.6989292045459));
#28730=CARTESIAN_POINT('Ctrl Pts',(-2.83712397431085,-2.93903939313352,
-30.7047430608813));
#28731=CARTESIAN_POINT('Ctrl Pts',(-2.92304712620692,-2.85609575013158,
-30.7105607423043));
#28732=CARTESIAN_POINT('Ctrl Pts',(-3.00524752123524,-2.76946066331204,
-30.7163784237272));
#28733=CARTESIAN_POINT('Ctrl Pts',(-3.0834118540804,-2.67951419815542,-30.7221961051502));
#28734=CARTESIAN_POINT('Ctrl Pts',(-3.16168694570897,-2.58944027894539,
-30.7280220302221));
#28735=CARTESIAN_POINT('Ctrl Pts',(-3.23591430765873,-2.49604593459566,
-30.7338479552939));
#28736=CARTESIAN_POINT('Ctrl Pts',(-3.30582286615256,-2.39974168977057,
-30.7396738803658));
#28737=CARTESIAN_POINT('Ctrl Pts',(-3.32237387826253,-2.376941438175,-30.7410531815342));
#28738=CARTESIAN_POINT('Ctrl Pts',(-3.33868301416142,-2.3539781956605,-30.7424324827027));
#28739=CARTESIAN_POINT('Ctrl Pts',(-3.35474705291792,-2.33085761275512,
-30.7438117838712));
#28740=CARTESIAN_POINT('Ctrl Pts',(-3.42331240557961,-2.23217315707866,
-30.7496989877354));
#28741=CARTESIAN_POINT('Ctrl Pts',(-3.48762617031097,-2.13030776213689,
-30.7555861915996));
#28742=CARTESIAN_POINT('Ctrl Pts',(-3.54738393391391,-2.02565846711864,
-30.7614733954638));
#28743=CARTESIAN_POINT('Ctrl Pts',(-3.60706316142376,-1.9211467064772,-30.7673528621243));
#28744=CARTESIAN_POINT('Ctrl Pts',(-3.66219810464387,-1.81385866534241,
-30.7732323287848));
#28745=CARTESIAN_POINT('Ctrl Pts',(-3.71252654954439,-1.70422170474619,
-30.7791117954454));
#28746=CARTESIAN_POINT('Ctrl Pts',(-3.76279980455952,-1.59470497141514,
-30.7849848147163));
#28747=CARTESIAN_POINT('Ctrl Pts',(-3.80827688453195,-1.48284480201287,
-30.7908578339872));
#28748=CARTESIAN_POINT('Ctrl Pts',(-3.84874084897415,-1.36909418136144,
-30.7967308532581));
#28749=CARTESIAN_POINT('Ctrl Pts',(-3.88916423668627,-1.25545762833275,
-30.8025979831428));
#28750=CARTESIAN_POINT('Ctrl Pts',(-3.92458438771809,-1.13993477134696,
-30.8084651130274));
#28751=CARTESIAN_POINT('Ctrl Pts',(-3.95483223170249,-1.02299903181141,
-30.814332242912));
#28752=CARTESIAN_POINT('Ctrl Pts',(-3.98506197191538,-0.906133280004967,
-30.8201958612347));
#28753=CARTESIAN_POINT('Ctrl Pts',(-4.01012546641762,-0.787856711325189,
-30.8260594795573));
#28754=CARTESIAN_POINT('Ctrl Pts',(-4.02990337715007,-0.668658186844704,
-30.83192309788));
#28755=CARTESIAN_POINT('Ctrl Pts',(-4.04967567644589,-0.54949348165766,
-30.8377850525627));
#28756=CARTESIAN_POINT('Ctrl Pts',(-4.06416530707864,-0.429407731267402,
-30.8436470072454));
#28757=CARTESIAN_POINT('Ctrl Pts',(-4.07330404263058,-0.308899945434376,
-30.8495089619281));
#28758=CARTESIAN_POINT('Ctrl Pts',(-4.08115411744783,-0.205385063153964,
-30.8545443174839));
#28759=CARTESIAN_POINT('Ctrl Pts',(-4.08505678108027,-0.101559090407424,
-30.8595796730397));
#28760=CARTESIAN_POINT('Ctrl Pts',(-4.08499937550953,0.00225877991778599,
-30.8646150285955));
#28761=CARTESIAN_POINT('Ctrl Pts',(-4.08499937550906,0.00225878076645493,
-30.8646150286367));
#28762=CARTESIAN_POINT('Ctrl Pts',(-4.08492561213899,0.135659651349435,
-30.8710852135166));
#28763=CARTESIAN_POINT('Ctrl Pts',(-4.07831318027114,0.268830275595934,
-30.8775553983965));
#28764=CARTESIAN_POINT('Ctrl Pts',(-4.06525415584447,0.401165362898193,
-30.8840255832764));
#28765=CARTESIAN_POINT('Ctrl Pts',(-4.05215046831583,0.533953048748885,
-30.8905178968022));
#28766=CARTESIAN_POINT('Ctrl Pts',(-4.03255612843008,0.66589925285231,-30.897010210328));
#28767=CARTESIAN_POINT('Ctrl Pts',(-4.00661426767472,0.796408883718279,
-30.9035025238538));
#28768=CARTESIAN_POINT('Ctrl Pts',(-3.98054550005077,0.927556964105285,
-30.9100265975987));
#28769=CARTESIAN_POINT('Ctrl Pts',(-3.94806706131849,1.05725416485448,-30.9165506713435));
#28770=CARTESIAN_POINT('Ctrl Pts',(-3.90937308787973,1.18491647796868,-30.9230747450883));
#28771=CARTESIAN_POINT('Ctrl Pts',(-3.87514566071344,1.29784239732178,-30.9288457279852));
#28772=CARTESIAN_POINT('Ctrl Pts',(-3.83605559115198,1.4091762978872,-30.9346167108821));
#28773=CARTESIAN_POINT('Ctrl Pts',(-3.79226783004088,1.51852879631472,-30.9403876937791));
#28774=CARTESIAN_POINT('Ctrl Pts',(-3.74806677993901,1.62891341382224,-30.9462131458618));
#28775=CARTESIAN_POINT('Ctrl Pts',(-3.69897144175243,1.73754311851044,-30.9520385979445));
#28776=CARTESIAN_POINT('Ctrl Pts',(-3.64514196067406,1.84395365628674,-30.9578640500273));
#28777=CARTESIAN_POINT('Ctrl Pts',(-3.5913800444854,1.95023063126244,-30.9636821902055));
#28778=CARTESIAN_POINT('Ctrl Pts',(-3.53289598698534,2.05429361865815,-30.9695003303837));
#28779=CARTESIAN_POINT('Ctrl Pts',(-3.46989848950998,2.15569698067617,-30.9753184705619));
#28780=CARTESIAN_POINT('Ctrl Pts',(-3.40696367676164,2.25699944278035,-30.9811308214858));
#28781=CARTESIAN_POINT('Ctrl Pts',(-3.33952457267184,2.35564719972549,-30.9869431724098));
#28782=CARTESIAN_POINT('Ctrl Pts',(-3.26783613254311,2.45121847472756,-30.9927555233338));
#28783=CARTESIAN_POINT('Ctrl Pts',(-3.19372632977344,2.55001778362771,-30.9987641933485));
#28784=CARTESIAN_POINT('Ctrl Pts',(-3.11507525756464,2.64552871191254,-31.0047728633632));
#28785=CARTESIAN_POINT('Ctrl Pts',(-3.03221404090021,2.73731675371477,-31.0107815333779));
#28786=CARTESIAN_POINT('Ctrl Pts',(-2.95214939464771,2.82600694428811,-31.0165874104642));
#28787=CARTESIAN_POINT('Ctrl Pts',(-2.8681544986675,2.91122116165802,-31.0223932875505));
#28788=CARTESIAN_POINT('Ctrl Pts',(-2.78056907741362,2.99260097669755,-31.0281991646368));
#28789=CARTESIAN_POINT('Ctrl Pts',(-2.69299634695159,3.0739690001138,-31.0340042004738));
#28790=CARTESIAN_POINT('Ctrl Pts',(-2.60183442470136,3.15150344847954,-31.0398092363108));
#28791=CARTESIAN_POINT('Ctrl Pts',(-2.50745903644586,3.22488359178219,-31.0456142721478));
#28792=CARTESIAN_POINT('Ctrl Pts',(-2.41307509347945,3.2982703866698,-31.0514198341855));
#28793=CARTESIAN_POINT('Ctrl Pts',(-2.31547742748063,3.36750187732411,-31.0572253962233));
#28794=CARTESIAN_POINT('Ctrl Pts',(-2.21507338178205,3.43229877972776,-31.063030958261));
#28795=CARTESIAN_POINT('Ctrl Pts',(-2.11463658573953,3.49711681794146,-31.068838413989));
#28796=CARTESIAN_POINT('Ctrl Pts',(-2.01139193209287,3.55749716998283,-31.0746458697169));
#28797=CARTESIAN_POINT('Ctrl Pts',(-1.90577360130433,3.61320522259275,-31.0804533254448));
#28798=CARTESIAN_POINT('Ctrl Pts',(-1.80003885332598,3.66897467907912,-31.086267182407));
#28799=CARTESIAN_POINT('Ctrl Pts',(-1.69192556689879,3.72006136601361,-31.0920810393691));
#28800=CARTESIAN_POINT('Ctrl Pts',(-1.58189038937199,3.76627771095183,-31.0978948963313));
#28801=CARTESIAN_POINT('Ctrl Pts',(-1.47178281709053,3.81252446272019,-31.1037125783679));
#28802=CARTESIAN_POINT('Ctrl Pts',(-1.35975121732951,3.85389434991448,-31.1095302604046));
#28803=CARTESIAN_POINT('Ctrl Pts',(-1.24626841271652,3.89024935492123,-31.1153479424412));
#28804=CARTESIAN_POINT('Ctrl Pts',(-1.13262480355803,3.9266558747815,-31.1211738681031));
#28805=CARTESIAN_POINT('Ctrl Pts',(-1.0175262775519,3.95803322277259,-31.126999793765));
#28806=CARTESIAN_POINT('Ctrl Pts',(-0.90145699208723,3.98429420241742,-31.1328257194269));
#28807=CARTESIAN_POINT('Ctrl Pts',(-0.87397745222479,3.9905115202383,-31.1342050141802));
#28808=CARTESIAN_POINT('Ctrl Pts',(-0.846443525971942,3.99644228842767,
-31.1355843089335));
#28809=CARTESIAN_POINT('Ctrl Pts',(-0.818861676052402,4.00208577562908,
-31.1369636036868));
#28810=CARTESIAN_POINT('Ctrl Pts',(-0.702359155593036,4.02592320803711,
-31.1427895840212));
#28811=CARTESIAN_POINT('Ctrl Pts',(-0.584628507797557,4.04470739476196,
-31.1486155643556));
#28812=CARTESIAN_POINT('Ctrl Pts',(-0.466145630715787,4.05831655381447,
-31.15444154469));
#28813=CARTESIAN_POINT('Ctrl Pts',(-0.34781401136114,4.07190833912897,-31.1602600874556));
#28814=CARTESIAN_POINT('Ctrl Pts',(-0.228732474960152,4.08033819224685,
-31.1660786302213));
#28815=CARTESIAN_POINT('Ctrl Pts',(-0.109388066938815,4.08353514137094,
-31.1718971729869));
#28816=CARTESIAN_POINT('Ctrl Pts',(0.00981731446799178,4.08672836630702,
-31.1777089376193));
#28817=CARTESIAN_POINT('Ctrl Pts',(0.129284552250609,4.08470081266939,-31.1835207022516));
#28818=CARTESIAN_POINT('Ctrl Pts',(0.248521322754568,4.07743327991229,-31.189332466884));
#28819=CARTESIAN_POINT('Ctrl Pts',(0.367680019558455,4.070170505781,-31.1951404260965));
#28820=CARTESIAN_POINT('Ctrl Pts',(0.486608143423988,4.05767460030551,-31.2009483853091));
#28821=CARTESIAN_POINT('Ctrl Pts',(0.604813442383292,4.0399784281494,-31.2067563445217));
#28822=CARTESIAN_POINT('Ctrl Pts',(0.722969186547713,4.02228967469777,-31.2125618688837));
#28823=CARTESIAN_POINT('Ctrl Pts',(0.840402305801329,3.99940505161285,-31.2183673932458));
#28824=CARTESIAN_POINT('Ctrl Pts',(0.95662637542646,3.97140919294882,-31.2241729176079));
#28825=CARTESIAN_POINT('Ctrl Pts',(1.07282909645558,3.94341847669875,-31.2299773755834));
#28826=CARTESIAN_POINT('Ctrl Pts',(1.18782281360997,3.91031848945809,-31.2357818335588));
#28827=CARTESIAN_POINT('Ctrl Pts',(1.30113261510672,3.87224468724609,-31.2415862915343));
#28828=CARTESIAN_POINT('Ctrl Pts',(1.41449321598884,3.83415381567445,-31.2473933517815));
#28829=CARTESIAN_POINT('Ctrl Pts',(1.52616800452399,3.79108480033464,-31.2532004120287));
#28830=CARTESIAN_POINT('Ctrl Pts',(1.6356985823936,3.7432225618517,-31.259007472276));
#28831=CARTESIAN_POINT('Ctrl Pts',(1.74525281094271,3.69534998858841,-31.264815786428));
#28832=CARTESIAN_POINT('Ctrl Pts',(1.85266153693647,3.64268230381903,-31.2706241005801));
#28833=CARTESIAN_POINT('Ctrl Pts',(1.95748887066811,3.58545148080552,-31.2764324147321));
#28834=CARTESIAN_POINT('Ctrl Pts',(2.06242494028727,3.52816129308138,-31.282246753765));
#28835=CARTESIAN_POINT('Ctrl Pts',(2.16477391544684,3.46629871683843,-31.2880610927979));
#28836=CARTESIAN_POINT('Ctrl Pts',(2.26412673941784,3.40014045413614,-31.2938754318308));
#28837=CARTESIAN_POINT('Ctrl Pts',(2.34025237969557,3.34944899005311,-31.2983304665644));
#28838=CARTESIAN_POINT('Ctrl Pts',(2.41461955876163,3.29623651745497,-31.302785501298));
#28839=CARTESIAN_POINT('Ctrl Pts',(2.4870572760686,3.24064362520075,-31.3072405360316));
#28840=CARTESIAN_POINT('',(-4.0849998777634,-0.000999336289953151,-30.7603849714308));
#28841=CARTESIAN_POINT('Ctrl Pts',(-4.0849998777634,-0.000999336289958593,
-30.7603849714308));
#28842=CARTESIAN_POINT('Ctrl Pts',(-4.08502878140532,0.117150454651573,
-30.7661717510729));
#28843=CARTESIAN_POINT('Ctrl Pts',(-4.07992758781669,0.235499771329081,
-30.771958530715));
#28844=CARTESIAN_POINT('Ctrl Pts',(-4.06967048002941,0.353563550125268,
-30.7777453103571));
#28845=CARTESIAN_POINT('Ctrl Pts',(-4.05942604544232,0.471481454866637,
-30.7835249401264));
#28846=CARTESIAN_POINT('Ctrl Pts',(-4.0440383996604,0.58911411442606,-30.7893045698956));
#28847=CARTESIAN_POINT('Ctrl Pts',(-4.02353372521156,0.70597546847266,-30.7950841996648));
#28848=CARTESIAN_POINT('Ctrl Pts',(-4.00304886281704,0.822723908583459,
-30.8008582450323));
#28849=CARTESIAN_POINT('Ctrl Pts',(-3.97745687652882,0.938702119897351,
-30.8066322903999));
#28850=CARTESIAN_POINT('Ctrl Pts',(-3.94683577764503,1.05342885108637,-30.8124063357674));
#28851=CARTESIAN_POINT('Ctrl Pts',(-3.91623499835199,1.16807945175393,-30.818176549586));
#28852=CARTESIAN_POINT('Ctrl Pts',(-3.88061185040692,1.28147982521651,-30.8239467634046));
#28853=CARTESIAN_POINT('Ctrl Pts',(-3.84009535765694,1.39315923142388,-30.8297169772232));
#28854=CARTESIAN_POINT('Ctrl Pts',(-3.79959285552512,1.50480007397923,-30.835485198548));
#28855=CARTESIAN_POINT('Ctrl Pts',(-3.75420050846812,1.61472074181599,-30.8412534198729));
#28856=CARTESIAN_POINT('Ctrl Pts',(-3.70409691358811,1.7224665612856,-30.8470216411977));
#28857=CARTESIAN_POINT('Ctrl Pts',(-3.65399840620415,1.83020144029411,-30.85278927682));
#28858=CARTESIAN_POINT('Ctrl Pts',(-3.59918977690339,1.93576153470512,-30.8585569124423));
#28859=CARTESIAN_POINT('Ctrl Pts',(-3.539897097881,2.03871369652868,-30.8643245480646));
#28860=CARTESIAN_POINT('Ctrl Pts',(-3.48059598553024,2.14168050146506,-30.8700930040304));
#28861=CARTESIAN_POINT('Ctrl Pts',(-3.41680976255271,2.24203827781851,-30.8758614599962));
#28862=CARTESIAN_POINT('Ctrl Pts',(-3.34880926292386,2.33938058480346,-30.8816299159621));
#28863=CARTESIAN_POINT('Ctrl Pts',(-3.28074086235099,2.43682009158211,-30.8874041319386));
#28864=CARTESIAN_POINT('Ctrl Pts',(-3.20845001801478,2.531237775147,-30.8931783479151));
#28865=CARTESIAN_POINT('Ctrl Pts',(-3.13224961987479,2.62225805724651,-30.8989525638916));
#28866=CARTESIAN_POINT('Ctrl Pts',(-3.05601051015036,2.71332457977812,-30.9047297133049));
#28867=CARTESIAN_POINT('Ctrl Pts',(-2.97585817003844,2.80098995764446,-30.9105068627182));
#28868=CARTESIAN_POINT('Ctrl Pts',(-2.89214309340475,2.88491478683014,-30.9162840121315));
#28869=CARTESIAN_POINT('Ctrl Pts',(-2.80829517133501,2.96897279430314,-30.9220703291638));
#28870=CARTESIAN_POINT('Ctrl Pts',(-2.72087352310968,3.04927811451934,-30.9278566461962));
#28871=CARTESIAN_POINT('Ctrl Pts',(-2.63026287228673,3.1255307105626,-30.9336429632285));
#28872=CARTESIAN_POINT('Ctrl Pts',(-2.55198804997586,3.19140219864728,-30.9386415250248));
#28873=CARTESIAN_POINT('Ctrl Pts',(-2.47133408077662,3.25424990784216,-30.9436400868211));
#28874=CARTESIAN_POINT('Ctrl Pts',(-2.38856553803204,3.31390700993943,-30.9486386486174));
#28875=CARTESIAN_POINT('Ctrl Pts',(-2.29210496822836,3.38343291761305,-30.9544640999675));
#28876=CARTESIAN_POINT('Ctrl Pts',(-2.1924519525515,3.44885491838803,-30.9602895513175));
#28877=CARTESIAN_POINT('Ctrl Pts',(-2.08999043653105,3.50986680305802,-30.9661150026675));
#28878=CARTESIAN_POINT('Ctrl Pts',(-1.98765752650204,3.57080210781565,-30.9719331421215));
#28879=CARTESIAN_POINT('Ctrl Pts',(-1.88252347519659,3.62733809957456,-30.9777512815756));
#28880=CARTESIAN_POINT('Ctrl Pts',(-1.77500325432677,3.67921030210688,-30.9835694210296));
#28881=CARTESIAN_POINT('Ctrl Pts',(-1.66759001969913,3.73103089005007,-30.9893817712389));
#28882=CARTESIAN_POINT('Ctrl Pts',(-1.55779570442558,3.77819674462592,-30.9951941214482));
#28883=CARTESIAN_POINT('Ctrl Pts',(-1.44606155265126,3.82048831773424,-31.0010064716574));
#28884=CARTESIAN_POINT('Ctrl Pts',(-1.33055342710085,3.86420834655934,-31.0070151419436));
#28885=CARTESIAN_POINT('Ctrl Pts',(-1.21297248583528,3.90271876722747,-31.0130238122297));
#28886=CARTESIAN_POINT('Ctrl Pts',(-1.09383110888818,3.93583009100094,-31.0190324825159));
#28887=CARTESIAN_POINT('Ctrl Pts',(-0.978710778472982,3.96782390063249,
-31.024838358916));
#28888=CARTESIAN_POINT('Ctrl Pts',(-0.862134067259083,3.99477705599787,
-31.0306442353162));
#28889=CARTESIAN_POINT('Ctrl Pts',(-0.744579858420503,4.01656891319376,
-31.0364501117163));
#28890=CARTESIAN_POINT('Ctrl Pts',(-0.62704268249851,4.03835761287713,-31.042255146879));
#28891=CARTESIAN_POINT('Ctrl Pts',(-0.508528691703095,4.05498642731745,
-31.0480601820417));
#28892=CARTESIAN_POINT('Ctrl Pts',(-0.389526970813251,4.06638583253103,
-31.0538652172043));
#28893=CARTESIAN_POINT('Ctrl Pts',(-0.270514462684037,4.07778627107515,
-31.0596707785804));
#28894=CARTESIAN_POINT('Ctrl Pts',(-0.151014542731728,4.08395631899025,
-31.0654763399565));
#28895=CARTESIAN_POINT('Ctrl Pts',(-0.0315207883900234,4.08487838740632,
-31.0712819013326));
#28896=CARTESIAN_POINT('Ctrl Pts',(0.0880119433641171,4.08580075658992,
-31.0770893564123));
#28897=CARTESIAN_POINT('Ctrl Pts',(0.207538097719214,4.08147173864878,-31.082896811492));
#28898=CARTESIAN_POINT('Ctrl Pts',(0.326565368729646,4.07192584165607,-31.0887042665718));
#28899=CARTESIAN_POINT('Ctrl Pts',(0.445723837348451,4.06236942271452,-31.0945181229091));
#28900=CARTESIAN_POINT('Ctrl Pts',(0.564381918077031,4.04758467950395,-31.1003319792464));
#28901=CARTESIAN_POINT('Ctrl Pts',(0.682053536347371,4.02765787692501,-31.1061458355837));
#28902=CARTESIAN_POINT('Ctrl Pts',(0.799802573837945,4.00771796398402,-31.1119635170084));
#28903=CARTESIAN_POINT('Ctrl Pts',(0.916563458334111,3.98262933956737,-31.1177811984331));
#28904=CARTESIAN_POINT('Ctrl Pts',(1.03186300602667,3.95252877747824,-31.1235988798578));
#28905=CARTESIAN_POINT('Ctrl Pts',(1.14732593306399,3.92238556292247,-31.1294248049313));
#28906=CARTESIAN_POINT('Ctrl Pts',(1.26132300197495,3.88721635606053,-31.1352507300048));
#28907=CARTESIAN_POINT('Ctrl Pts',(1.37339868535747,3.84720691555034,-31.1410766550783));
#28908=CARTESIAN_POINT('Ctrl Pts',(1.39993286094534,3.83773458856888,-31.1424559562273));
#28909=CARTESIAN_POINT('Ctrl Pts',(1.42635944038976,3.82799116528291,-31.1438352573762));
#28910=CARTESIAN_POINT('Ctrl Pts',(1.45267257479978,3.81797949057149,-31.1452145585252));
#28911=CARTESIAN_POINT('Ctrl Pts',(1.56379356903068,3.77569994946805,-31.1510393801763));
#28912=CARTESIAN_POINT('Ctrl Pts',(1.67324497728437,3.72849754926938,-31.1568642018273));
#28913=CARTESIAN_POINT('Ctrl Pts',(1.78055999398934,3.67652432438637,-31.1626890234784));
#28914=CARTESIAN_POINT('Ctrl Pts',(1.88775658178706,3.62460845524368,-31.1685074170704));
#28915=CARTESIAN_POINT('Ctrl Pts',(1.99282110020167,3.56793240220706,-31.1743258106624));
#28916=CARTESIAN_POINT('Ctrl Pts',(2.09530430566209,3.50669714498898,-31.1801442042544));
#28917=CARTESIAN_POINT('Ctrl Pts',(2.19767752415647,3.44552760663798,-31.1859563534334));
#28918=CARTESIAN_POINT('Ctrl Pts',(2.29747459476058,3.37980881012102,-31.1917685026124));
#28919=CARTESIAN_POINT('Ctrl Pts',(2.39426943353907,3.30978834362871,-31.1975806517915));
#28920=CARTESIAN_POINT('Ctrl Pts',(2.42551596135264,3.28718490235662,-31.199456882831));
#28921=CARTESIAN_POINT('Ctrl Pts',(2.45644982626913,3.2641335517492,-31.2013331138705));
#28922=CARTESIAN_POINT('Ctrl Pts',(2.48705727606859,3.24064362520075,-31.2032093449099));
#28923=CARTESIAN_POINT('Ctrl Pts',(2.4870572760686,3.24064362520074,-29.953048263356));
#28924=CARTESIAN_POINT('Ctrl Pts',(2.55581230516247,3.1878770407962,-29.9572852085968));
#28925=CARTESIAN_POINT('Ctrl Pts',(2.62281785134413,3.1329747184487,-29.9615221538375));
#28926=CARTESIAN_POINT('Ctrl Pts',(2.68793986680533,3.07606961436807,-29.9657590990783));
#28927=CARTESIAN_POINT('Ctrl Pts',(2.77747548878455,2.99783134346125,-29.9715844336405));
#28928=CARTESIAN_POINT('Ctrl Pts',(2.86373562734555,2.91555542942311,-29.9774097682026));
#28929=CARTESIAN_POINT('Ctrl Pts',(2.94633518555609,2.82954660225877,-29.9832351027648));
#28930=CARTESIAN_POINT('Ctrl Pts',(3.0288310416831,2.74364575744655,-29.9890531237366));
#28931=CARTESIAN_POINT('Ctrl Pts',(3.10767517837059,2.6540216129624,-29.9948711447084));
#28932=CARTESIAN_POINT('Ctrl Pts',(3.18251613281278,2.56101855994571,-30.0006891656802));
#28933=CARTESIAN_POINT('Ctrl Pts',(3.25728259667433,2.46810807458094,-30.0065013958686));
#28934=CARTESIAN_POINT('Ctrl Pts',(3.32805355063709,2.37182568735685,-30.0123136260569));
#28935=CARTESIAN_POINT('Ctrl Pts',(3.39451535374224,2.27255154247559,-30.0181258562453));
#28936=CARTESIAN_POINT('Ctrl Pts',(3.46322392174458,2.1699213998107,-30.0241345709428));
#28937=CARTESIAN_POINT('Ctrl Pts',(3.52732652509763,2.06409396154969,-30.0301432856404));
#28938=CARTESIAN_POINT('Ctrl Pts',(3.58652269135608,1.95552550082783,-30.0361520003379));
#28939=CARTESIAN_POINT('Ctrl Pts',(3.64371933917572,1.85062424784606,-30.0419577536514));
#28940=CARTESIAN_POINT('Ctrl Pts',(3.6963354435903,1.74316454032156,-30.047763506965));
#28941=CARTESIAN_POINT('Ctrl Pts',(3.74414519394622,1.63358555535039,-30.0535692602785));
#28942=CARTESIAN_POINT('Ctrl Pts',(3.79194800921432,1.52402246546081,-30.0593741714331));
#28943=CARTESIAN_POINT('Ctrl Pts',(3.83494569383507,1.41234108338631,-30.0651790825877));
#28944=CARTESIAN_POINT('Ctrl Pts',(3.87295992550226,1.29900208446851,-30.0709839937423));
#28945=CARTESIAN_POINT('Ctrl Pts',(3.91097759798832,1.18565282678842,-30.0767894303224));
#28946=CARTESIAN_POINT('Ctrl Pts',(3.94401079092465,1.07064604082764,-30.0825948669025));
#28947=CARTESIAN_POINT('Ctrl Pts',(3.97193075561521,0.954458523246536,-30.0884003034826));
#28948=CARTESIAN_POINT('Ctrl Pts',(3.99985982450558,0.838233118999529,-30.0942076331115));
#28949=CARTESIAN_POINT('Ctrl Pts',(4.02267225388032,0.72082661394739,-30.1000149627404));
#28950=CARTESIAN_POINT('Ctrl Pts',(4.04029032990276,0.602726347602504,-30.1058222923693));
#28951=CARTESIAN_POINT('Ctrl Pts',(4.05792782479383,0.48449590963416,-30.1116360229111));
#28952=CARTESIAN_POINT('Ctrl Pts',(4.07035947817291,0.365570587843263,-30.1174497534529));
#28953=CARTESIAN_POINT('Ctrl Pts',(4.07755940143801,0.246443356056747,-30.1232634839948));
#28954=CARTESIAN_POINT('Ctrl Pts',(4.08476406139379,0.127237752761492,-30.1290810392778));
#28955=CARTESIAN_POINT('Ctrl Pts',(4.08673012989666,0.00783038195283492,
-30.1348985945609));
#28956=CARTESIAN_POINT('Ctrl Pts',(4.08348383393083,-0.111286917584897,
-30.140716149844));
#28957=CARTESIAN_POINT('Ctrl Pts',(4.08023293762059,-0.23057301892339,-30.1465419492176));
#28958=CARTESIAN_POINT('Ctrl Pts',(4.07175496331674,-0.349567823055712,
-30.1523677485913));
#28959=CARTESIAN_POINT('Ctrl Pts',(4.05812784669207,-0.467785613184488,
-30.1581935479649));
#28960=CARTESIAN_POINT('Ctrl Pts',(4.05489875206701,-0.495798614115334,
-30.159574034972));
#28961=CARTESIAN_POINT('Ctrl Pts',(4.05138075511121,-0.523768036727955,
-30.160954521979));
#28962=CARTESIAN_POINT('Ctrl Pts',(4.0475753082676,-0.551687523787168,-30.1623350089861));
#28963=CARTESIAN_POINT('Ctrl Pts',(4.03151677086633,-0.669504470282694,
-30.1681605015356));
#28964=CARTESIAN_POINT('Ctrl Pts',(4.01028415179671,-0.786808135138811,
-30.1739859940851));
#28965=CARTESIAN_POINT('Ctrl Pts',(3.98392001214754,-0.903109260726691,
-30.1798114866346));
#28966=CARTESIAN_POINT('Ctrl Pts',(3.95758896192584,-1.01926441767273,-30.1856296676535));
#28967=CARTESIAN_POINT('Ctrl Pts',(3.92613929087898,-1.1344191436337,-30.1914478486725));
#28968=CARTESIAN_POINT('Ctrl Pts',(3.88966518421875,-1.2480904433079,-30.1972660296914));
#28969=CARTESIAN_POINT('Ctrl Pts',(3.85322736831024,-1.36164864310685,-30.2030784217772));
#28970=CARTESIAN_POINT('Ctrl Pts',(3.81177518619867,-1.47372596663755,-30.2088908138631));
#28971=CARTESIAN_POINT('Ctrl Pts',(3.76545348818231,-1.58385132772482,-30.2147032059489));
#28972=CARTESIAN_POINT('Ctrl Pts',(3.7175676806409,-1.697695208072,-30.220711860655));
#28973=CARTESIAN_POINT('Ctrl Pts',(3.66447778562353,-1.80945253930661,-30.226720515361));
#28974=CARTESIAN_POINT('Ctrl Pts',(3.60639944226682,-1.91862139642442,-30.2327291700671));
#28975=CARTESIAN_POINT('Ctrl Pts',(3.55028070006073,-2.02410682516504,-30.2385350888479));
#28976=CARTESIAN_POINT('Ctrl Pts',(3.48950491311273,-2.12717524673955,-30.2443410076287));
#28977=CARTESIAN_POINT('Ctrl Pts',(3.42431455073011,-2.22739643028762,-30.2501469264095));
#28978=CARTESIAN_POINT('Ctrl Pts',(3.35913363272308,-2.32760309441189,-30.2559520040648));
#28979=CARTESIAN_POINT('Ctrl Pts',(3.28953963361879,-2.42496299892272,-30.2617570817201));
#28980=CARTESIAN_POINT('Ctrl Pts',(3.21581910435427,-2.51907373613201,-30.2675621593754));
#28981=CARTESIAN_POINT('Ctrl Pts',(3.14209189171015,-2.61319300526298,-30.2733677633094));
#28982=CARTESIAN_POINT('Ctrl Pts',(3.06423765671202,-2.70406220021829,-30.2791733672433));
#28983=CARTESIAN_POINT('Ctrl Pts',(2.98258368984066,-2.79131143606307,-30.2849789711772));
#28984=CARTESIAN_POINT('Ctrl Pts',(2.90090308837341,-2.87858913161689,-30.2907864688331));
#28985=CARTESIAN_POINT('Ctrl Pts',(2.81542056870581,-2.96224422196422,-30.296593966489));
#28986=CARTESIAN_POINT('Ctrl Pts',(2.72650030718747,-3.04194363440656,-30.302401464145));
#28987=CARTESIAN_POINT('Ctrl Pts',(2.63748203703935,-3.12173089218444,-30.3082153628717));
#28988=CARTESIAN_POINT('Ctrl Pts',(2.54501876580553,-3.19755349686545,-30.3140292615984));
#28989=CARTESIAN_POINT('Ctrl Pts',(2.44950789225112,-3.26911854875278,-30.3198431603251));
#28990=CARTESIAN_POINT('Ctrl Pts',(2.35393418106028,-3.34073068406155,-30.3256608840786));
#28991=CARTESIAN_POINT('Ctrl Pts',(2.25530921053142,-3.40807945849512,-30.3314786078321));
#28992=CARTESIAN_POINT('Ctrl Pts',(2.15405810963678,-3.47091611254262,-30.3372963315857));
#28993=CARTESIAN_POINT('Ctrl Pts',(2.05266354416293,-3.53384180102089,-30.3431222985809));
#28994=CARTESIAN_POINT('Ctrl Pts',(1.94863577614577,-3.5922424099139,-30.348948265576));
#28995=CARTESIAN_POINT('Ctrl Pts',(1.84242327695448,-3.64591572427783,-30.3547742325712));
#28996=CARTESIAN_POINT('Ctrl Pts',(1.8172848010542,-3.65861917565972,-30.3561531280121));
#28997=CARTESIAN_POINT('Ctrl Pts',(1.79202402162829,-3.67105802936119,-30.3575320234531));
#28998=CARTESIAN_POINT('Ctrl Pts',(1.76664702472144,-3.68323000775717,-30.358910918894));
#28999=CARTESIAN_POINT('Ctrl Pts',(1.65943611569282,-3.73465330552956,-30.3647363770528));
#29000=CARTESIAN_POINT('Ctrl Pts',(1.54980661304529,-3.78147396035117,-30.3705618352116));
#29001=CARTESIAN_POINT('Ctrl Pts',(1.43819045162136,-3.82345828078,-30.3763872933704));
#29002=CARTESIAN_POINT('Ctrl Pts',(1.32671438278899,-3.86538990550438,-30.3822054398324));
#29003=CARTESIAN_POINT('Ctrl Pts',(1.2132569933931,-3.90249712720995,-30.3880235862944));
#29004=CARTESIAN_POINT('Ctrl Pts',(1.09827339743581,-3.93459280542279,-30.3938417327564));
#29005=CARTESIAN_POINT('Ctrl Pts',(0.983404210146548,-3.96665654843859,
-30.3996540901631));
#29006=CARTESIAN_POINT('Ctrl Pts',(0.8670122281456,-3.99371855908819,-30.4054664475699));
#29007=CARTESIAN_POINT('Ctrl Pts',(0.749570501840176,-4.01564055447833,
-30.4112788049767));
#29008=CARTESIAN_POINT('Ctrl Pts',(0.628162224040345,-4.03830295727145,
-30.417287472636));
#29009=CARTESIAN_POINT('Ctrl Pts',(0.505632453066731,-4.05547183861424,
-30.4232961402954));
#29010=CARTESIAN_POINT('Ctrl Pts',(0.382518955690571,-4.06705105064313,
-30.4293048079548));
#29011=CARTESIAN_POINT('Ctrl Pts',(0.263560356499327,-4.07823948141679,
-30.4351106919805));
#29012=CARTESIAN_POINT('Ctrl Pts',(0.144057233575435,-4.08420940007617,
-30.4409165760062));
#29013=CARTESIAN_POINT('Ctrl Pts',(0.024502242208067,-4.08492651587844,
-30.4467224600319));
#29014=CARTESIAN_POINT('Ctrl Pts',(-0.0950354293644703,-4.08564352779297,
-30.4525275029658));
#29015=CARTESIAN_POINT('Ctrl Pts',(-0.214624546535855,-4.08110924778427,
-30.4583325458998));
#29016=CARTESIAN_POINT('Ctrl Pts',(-0.333771428519917,-4.07134150293288,
-30.4641375888337));
#29017=CARTESIAN_POINT('Ctrl Pts',(-0.452929113715939,-4.06157287242661,
-30.4699431581189));
#29018=CARTESIAN_POINT('Ctrl Pts',(-0.571644077331451,-4.04656986694565,
-30.4757487274041));
#29019=CARTESIAN_POINT('Ctrl Pts',(-0.689427376299411,-4.02640222690293,
-30.4815542966892));
#29020=CARTESIAN_POINT('Ctrl Pts',(-0.807249097334082,-4.00622800797834,
-30.487361759808));
#29021=CARTESIAN_POINT('Ctrl Pts',(-0.924138147339345,-3.98088587267945,
-30.4931692229268));
#29022=CARTESIAN_POINT('Ctrl Pts',(-1.03961602327505,-3.95049661740771,
-30.4989766860456));
#29023=CARTESIAN_POINT('Ctrl Pts',(-1.15522118737406,-3.92007386487552,
-30.5047905505751));
#29024=CARTESIAN_POINT('Ctrl Pts',(-1.26941167775888,-3.88459299165533,
-30.5106044151046));
#29025=CARTESIAN_POINT('Ctrl Pts',(-1.38172425354188,-3.84422464057112,
-30.5164182796341));
#29026=CARTESIAN_POINT('Ctrl Pts',(-1.49411072450046,-3.80382972944793,
-30.52223596935));
#29027=CARTESIAN_POINT('Ctrl Pts',(-1.60461644351643,-3.75854109062448,
-30.528053659066));
#29028=CARTESIAN_POINT('Ctrl Pts',(-1.71279976673854,-3.70857681045713,
-30.5338713487819));
#29029=CARTESIAN_POINT('Ctrl Pts',(-1.82113638694164,-3.65854173034503,
-30.5396972822294));
#29030=CARTESIAN_POINT('Ctrl Pts',(-1.92714368200098,-3.60381797186832,
-30.5455232156768));
#29031=CARTESIAN_POINT('Ctrl Pts',(-2.03040602722965,-3.54466872423778,
-30.5513491491242));
#29032=CARTESIAN_POINT('Ctrl Pts',(-2.05485226754216,-3.53066578135789,
-30.5527283756834));
#29033=CARTESIAN_POINT('Ctrl Pts',(-2.07914480153312,-3.51641499580859,
-30.5541076022426));
#29034=CARTESIAN_POINT('Ctrl Pts',(-2.10327837461796,-3.50192019881442,
-30.5554868288017));
#29035=CARTESIAN_POINT('Ctrl Pts',(-2.20521129883434,-3.44069855383277,
-30.5613122652524));
#29036=CARTESIAN_POINT('Ctrl Pts',(-2.30463204263936,-3.374924722447,-30.567137701703));
#29037=CARTESIAN_POINT('Ctrl Pts',(-2.40110779457756,-3.30483076099502,
-30.5729631381536));
#29038=CARTESIAN_POINT('Ctrl Pts',(-2.49746244931989,-3.23482478208795,
-30.5787812624662));
#29039=CARTESIAN_POINT('Ctrl Pts',(-2.59087913752951,-3.16050969663225,
-30.5845993867787));
#29040=CARTESIAN_POINT('Ctrl Pts',(-2.6809511614434,-3.08216253139825,-30.5904175110913));
#29041=CARTESIAN_POINT('Ctrl Pts',(-2.77093355698706,-3.00389332742711,
-30.596229845937));
#29042=CARTESIAN_POINT('Ctrl Pts',(-2.85757760328303,-2.92160029192114,
-30.6020421807826));
#29043=CARTESIAN_POINT('Ctrl Pts',(-2.9405075272883,-2.83560231378817,-30.6078545156283));
#29044=CARTESIAN_POINT('Ctrl Pts',(-3.0262388304751,-2.74669931737037,-30.61386319159));
#29045=CARTESIAN_POINT('Ctrl Pts',(-3.10800028326864,-2.65383690175527,
-30.6198718675517));
#29046=CARTESIAN_POINT('Ctrl Pts',(-3.18541567626639,-2.5574111850456,-30.6258805435135));
#29047=CARTESIAN_POINT('Ctrl Pts',(-3.26021800899849,-2.46424019842466,
-30.6316864040945));
#29048=CARTESIAN_POINT('Ctrl Pts',(-3.33096266304827,-2.36774292183173,
-30.6374922646755));
#29049=CARTESIAN_POINT('Ctrl Pts',(-3.39734990832777,-2.26831183931691,
-30.6432981252565));
#29050=CARTESIAN_POINT('Ctrl Pts',(-3.46372753284194,-2.16889516624336,
-30.6491031444586));
#29051=CARTESIAN_POINT('Ctrl Pts',(-3.52574877792394,-2.06654587204177,
-30.6549081636608));
#29052=CARTESIAN_POINT('Ctrl Pts',(-3.583156866379,-1.96168597663362,-30.660713182863));
#29053=CARTESIAN_POINT('Ctrl Pts',(-3.64057015753436,-1.85681657812889,
-30.6665187281543));
#29054=CARTESIAN_POINT('Ctrl Pts',(-3.69336926488391,-1.74943648394792,
-30.6723242734457));
#29055=CARTESIAN_POINT('Ctrl Pts',(-3.74134336481207,-1.63999232515787,
-30.6781298187371));
#29056=CARTESIAN_POINT('Ctrl Pts',(-3.78933311246614,-1.53051246893521,
-30.6839372576248));
#29057=CARTESIAN_POINT('Ctrl Pts',(-3.83249455906068,-1.41896758266827,
-30.6897446965126));
#29058=CARTESIAN_POINT('Ctrl Pts',(-3.87066525660072,-1.30582367544171,
-30.6955521354003));
#29059=CARTESIAN_POINT('Ctrl Pts',(-3.90887802733028,-1.19255505671236,
-30.7013659754673));
#29060=CARTESIAN_POINT('Ctrl Pts',(-3.94208893827324,-1.07768428581265,
-30.7071798155343));
#29061=CARTESIAN_POINT('Ctrl Pts',(-3.97018556064206,-0.961692057817527,
-30.7129936556013));
#29062=CARTESIAN_POINT('Ctrl Pts',(-3.99830066824993,-0.845623516590301,
-30.7188113206911));
#29063=CARTESIAN_POINT('Ctrl Pts',(-4.02129470776966,-0.728432448295096,
-30.724628985781));
#29064=CARTESIAN_POINT('Ctrl Pts',(-4.03910674923444,-0.610607622200049,
-30.7304466508709));
#29065=CARTESIAN_POINT('Ctrl Pts',(-4.05694403050203,-0.492615837399969,
-30.7362725596379));
#29066=CARTESIAN_POINT('Ctrl Pts',(-4.06958461511904,-0.373988906664999,
-30.742098468405));
#29067=CARTESIAN_POINT('Ctrl Pts',(-4.07701955093888,-0.255218693010852,
-30.747924377172));
#29068=CARTESIAN_POINT('Ctrl Pts',(-4.07877998887574,-0.227096380330193,
-30.7493038310179));
#29069=CARTESIAN_POINT('Ctrl Pts',(-4.08024880514175,-0.198966023605966,
-30.7506832848637));
#29070=CARTESIAN_POINT('Ctrl Pts',(-4.08142630741086,-0.170834121809958,
-30.7520627387096));
#29071=CARTESIAN_POINT('Ctrl Pts',(-4.08379426095805,-0.114260951299124,
-30.7548368162745));
#29072=CARTESIAN_POINT('Ctrl Pts',(-4.08498602187232,-0.0576382110579216,
-30.7576108938395));
#29073=CARTESIAN_POINT('Ctrl Pts',(-4.08499987776327,-0.000999336826385626,
-30.7603849714045));
#29074=CARTESIAN_POINT('Origin',(0.,0.,-25.2396150285955));
#29075=CARTESIAN_POINT('',(2.4870572760686,3.24064362520074,-28.7030585997167));
#29076=CARTESIAN_POINT('',(2.48705727606859,3.24064362520075,-28.807442179994));
#29077=CARTESIAN_POINT('',(2.4870572760686,3.24064362520075,-25.2396150285955));
#29078=CARTESIAN_POINT('',(-4.08246318168416,-0.00445590608020525,-28.2603840116597));
#29079=CARTESIAN_POINT('Ctrl Pts',(-4.08499758825475,-0.00443891347911176,
-28.2603849714045));
#29080=CARTESIAN_POINT('Ctrl Pts',(-4.08512632133835,0.114030243104064,
-28.2661368812369));
#29081=CARTESIAN_POINT('Ctrl Pts',(-4.08009719924304,0.232579851337021,
-28.2718887910694));
#29082=CARTESIAN_POINT('Ctrl Pts',(-4.06991623004305,0.350723367388326,
-28.2776407009018));
#29083=CARTESIAN_POINT('Ctrl Pts',(-4.05973778505935,0.468837591553652,
-28.2833911846358));
#29084=CARTESIAN_POINT('Ctrl Pts',(-4.04441006739671,0.586545509497618,
-28.2891416683697));
#29085=CARTESIAN_POINT('Ctrl Pts',(-4.02399111300928,0.703363719865031,
-28.2948921521037));
#29086=CARTESIAN_POINT('Ctrl Pts',(-4.00357219517005,0.820181721137633,
-28.3006426255448));
#29087=CARTESIAN_POINT('Ctrl Pts',(-3.97806213047916,0.936109608232255,
-28.3063930989858));
#29088=CARTESIAN_POINT('Ctrl Pts',(-3.94757030760067,1.05067295889327,-28.3121435724269));
#29089=CARTESIAN_POINT('Ctrl Pts',(-3.91707103353571,1.16526430502351,-28.3178954510923));
#29090=CARTESIAN_POINT('Ctrl Pts',(-3.8815876883295,1.27849004999528,-28.3236473297576));
#29091=CARTESIAN_POINT('Ctrl Pts',(-3.84127966719592,1.38989046992459,-28.329399208423));
#29092=CARTESIAN_POINT('Ctrl Pts',(-3.80092654050279,1.50141554936666,-28.3351575235667));
#29093=CARTESIAN_POINT('Ctrl Pts',(-3.75573810001732,1.61111083384206,-28.3409158387104));
#29094=CARTESIAN_POINT('Ctrl Pts',(-3.70592215450002,1.7185360004335,-28.3466741538541));
#29095=CARTESIAN_POINT('Ctrl Pts',(-3.65607626045009,1.82602574928012,-28.3524359308029));
#29096=CARTESIAN_POINT('Ctrl Pts',(-3.60159751384272,1.93124229436399,-28.3581977077516));
#29097=CARTESIAN_POINT('Ctrl Pts',(-3.54273911394695,2.03377102214343,-28.3639594847003));
#29098=CARTESIAN_POINT('Ctrl Pts',(-3.48378491100313,2.13646663459273,-28.369730640018));
#29099=CARTESIAN_POINT('Ctrl Pts',(-3.42043704149256,2.23646534248467,-28.3755017953357));
#29100=CARTESIAN_POINT('Ctrl Pts',(-3.35299154004781,2.33338225166127,-28.3812729506534));
#29101=CARTESIAN_POINT('Ctrl Pts',(-3.30671679128229,2.39987750378645,-28.3852325737075));
#29102=CARTESIAN_POINT('Ctrl Pts',(-3.25851398781532,2.4649226912196,-28.3891921967616));
#29103=CARTESIAN_POINT('Ctrl Pts',(-3.20848902628625,2.52840328432802,-28.3931518198157));
#29104=CARTESIAN_POINT('Ctrl Pts',(-3.13480852911598,2.62190224000785,-28.3989838481934));
#29105=CARTESIAN_POINT('Ctrl Pts',(-3.0569211542648,2.71232566598092,-28.4048158765711));
#29106=CARTESIAN_POINT('Ctrl Pts',(-2.97511270936837,2.79927300679208,-28.4106479049488));
#29107=CARTESIAN_POINT('Ctrl Pts',(-2.89340694843843,2.88611121341983,-28.4164726131066));
#29108=CARTESIAN_POINT('Ctrl Pts',(-2.80779018365383,2.96948171979137,-28.4222973212644));
#29109=CARTESIAN_POINT('Ctrl Pts',(-2.71858950157756,3.04901559883059,-28.4281220294222));
#29110=CARTESIAN_POINT('Ctrl Pts',(-2.62947773498685,3.12847019828015,-28.4339409314949));
#29111=CARTESIAN_POINT('Ctrl Pts',(-2.53678946060952,3.20409550973873,-28.4397598335676));
#29112=CARTESIAN_POINT('Ctrl Pts',(-2.44088935787284,3.27555860008993,-28.4455787356402));
#29113=CARTESIAN_POINT('Ctrl Pts',(-2.34190230406297,3.3493220327469,-28.451584943727));
#29114=CARTESIAN_POINT('Ctrl Pts',(-2.23949345769402,3.41865043738168,-28.4575911518138));
#29115=CARTESIAN_POINT('Ctrl Pts',(-2.1341021784629,3.4832216254324,-28.4635973599006));
#29116=CARTESIAN_POINT('Ctrl Pts',(-2.03211269591741,3.54570859878243,-28.469409700915));
#29117=CARTESIAN_POINT('Ctrl Pts',(-1.9273307206189,3.60374050069382,-28.4752220419294));
#29118=CARTESIAN_POINT('Ctrl Pts',(-1.82018425426441,3.65706908336825,-28.4810343829438));
#29119=CARTESIAN_POINT('Ctrl Pts',(-1.71305411494676,3.71038953980424,-28.4868458382705));
#29120=CARTESIAN_POINT('Ctrl Pts',(-1.60356056538362,3.75900792119536,-28.4926572935972));
#29121=CARTESIAN_POINT('Ctrl Pts',(-1.49215549176468,3.80272231281703,-28.4984687489239));
#29122=CARTESIAN_POINT('Ctrl Pts',(-1.38074132962146,3.84644027069737,-28.5042806783542));
#29123=CARTESIAN_POINT('Ctrl Pts',(-1.26741571220278,3.88525329475721,-28.5100926077846));
#29124=CARTESIAN_POINT('Ctrl Pts',(-1.15264916036561,3.91900815425389,-28.515904537215));
#29125=CARTESIAN_POINT('Ctrl Pts',(-1.03784639515901,3.95277366473883,-28.5217183005381));
#29126=CARTESIAN_POINT('Ctrl Pts',(-0.92160218145053,3.98147772156695,-28.5275320638612));
#29127=CARTESIAN_POINT('Ctrl Pts',(-0.804400192932084,4.00501751926391,
-28.5333458271843));
#29128=CARTESIAN_POINT('Ctrl Pts',(-0.687071603170412,4.0285827445811,-28.5391658705174));
#29129=CARTESIAN_POINT('Ctrl Pts',(-0.568783572669926,4.04697249560267,
-28.5449859138506));
#29130=CARTESIAN_POINT('Ctrl Pts',(-0.450028068493812,4.06013543340216,
-28.5508059571837));
#29131=CARTESIAN_POINT('Ctrl Pts',(-0.331195822144487,4.07330687735435,
-28.5566297615448));
#29132=CARTESIAN_POINT('Ctrl Pts',(-0.211895905580145,4.08124475368808,
-28.562453565906));
#29133=CARTESIAN_POINT('Ctrl Pts',(-0.0926218644566019,4.08394982709442,
-28.5682773702671));
#29134=CARTESIAN_POINT('Ctrl Pts',(0.0268181448968271,4.08665866457417,
-28.5741092783739));
#29135=CARTESIAN_POINT('Ctrl Pts',(0.146231801521961,4.08412017465436,-28.5799411864808));
#29136=CARTESIAN_POINT('Ctrl Pts',(0.265128984138461,4.07638707948224,-28.5857730945876));
#29137=CARTESIAN_POINT('Ctrl Pts',(0.292003834662801,4.07463913413763,-28.5870913062996));
#29138=CARTESIAN_POINT('Ctrl Pts',(0.318852333909899,4.07262599601133,-28.5884095180115));
#29139=CARTESIAN_POINT('Ctrl Pts',(0.345668893292544,4.07034863570799,-28.5897277297235));
#29140=CARTESIAN_POINT('Ctrl Pts',(0.464353441204676,4.06026950981499,-28.5955618622404));
#29141=CARTESIAN_POINT('Ctrl Pts',(0.582779642271394,4.04497959911709,-28.6013959947573));
#29142=CARTESIAN_POINT('Ctrl Pts',(0.700455418714115,4.02449837947464,-28.6072301272742));
#29143=CARTESIAN_POINT('Ctrl Pts',(0.817994270885021,4.00404099121169,-28.6130574713562));
#29144=CARTESIAN_POINT('Ctrl Pts',(0.934784037864472,3.97840437561073,-28.6188848154382));
#29145=CARTESIAN_POINT('Ctrl Pts',(1.05033640115567,3.94765986939191,-28.6247121595202));
#29146=CARTESIAN_POINT('Ctrl Pts',(1.16578128015835,3.91694396104234,-28.6305340831338));
#29147=CARTESIAN_POINT('Ctrl Pts',(1.27999065436538,3.88112971718499,-28.6363560067474));
#29148=CARTESIAN_POINT('Ctrl Pts',(1.39248566642517,3.84033965539514,-28.642177930361));
#29149=CARTESIAN_POINT('Ctrl Pts',(1.50489892442149,3.79957923717116,-28.647995622979));
#29150=CARTESIAN_POINT('Ctrl Pts',(1.61559991907097,3.75385033633467,-28.6538133155969));
#29151=CARTESIAN_POINT('Ctrl Pts',(1.72412488494293,3.70332531397399,-28.6596310082148));
#29152=CARTESIAN_POINT('Ctrl Pts',(1.83260372794383,3.65282176463633,-28.6654462283262));
#29153=CARTESIAN_POINT('Ctrl Pts',(1.93890801482212,3.59752632167616,-28.6712614484376));
#29154=CARTESIAN_POINT('Ctrl Pts',(2.04259438139677,3.53765928165593,-28.6770766685489));
#29155=CARTESIAN_POINT('Ctrl Pts',(2.14627427464938,3.4777959792402,-28.6828915256059));
#29156=CARTESIAN_POINT('Ctrl Pts',(2.24733621845074,3.41336184642097,-28.6887063826629));
#29157=CARTESIAN_POINT('Ctrl Pts',(2.34536224459767,3.34462269047135,-28.6945212397199));
#29158=CARTESIAN_POINT('Ctrl Pts',(2.393336107989,3.31098179930414,-28.6973670263855));
#29159=CARTESIAN_POINT('Ctrl Pts',(2.44058325170965,3.27631047839352,-28.7002128130511));
#29160=CARTESIAN_POINT('Ctrl Pts',(2.48705727606861,3.24064362520074,-28.7030585997167));
#29161=CARTESIAN_POINT('',(-1.05790442297295,-3.94563850749841,-28.));
#29162=CARTESIAN_POINT('Ctrl Pts',(-1.05790442297292,-3.94563850749842,
-28.));
#29163=CARTESIAN_POINT('Ctrl Pts',(-2.35746398375646,-3.59720065525805,
-28.0655253033026));
#29164=CARTESIAN_POINT('Ctrl Pts',(-3.81889380336946,-2.22310313068615,
-28.1523197509));
#29165=CARTESIAN_POINT('Ctrl Pts',(-4.08374969685893,-0.442080030969895,
-28.2391141984974));
#29166=CARTESIAN_POINT('Ctrl Pts',(-4.08069689719269,-0.00446774860307798,
-28.2603833427922));
#29167=CARTESIAN_POINT('',(1.05868926563988,-3.94542799184308,-28.0000001371954));
#29168=CARTESIAN_POINT('Origin',(0.,0.,-28.));
#29169=CARTESIAN_POINT('',(-4.08499944003493,0.00213890492626102,-28.3646150285541));
#29170=CARTESIAN_POINT('Ctrl Pts',(1.05868926563988,-3.94542799184308,-28.0000001371954));
#29171=CARTESIAN_POINT('Ctrl Pts',(0.944487741664465,-3.97607205068852,
-28.0057918022596));
#29172=CARTESIAN_POINT('Ctrl Pts',(0.828763515936965,-4.00180483333926,
-28.0115834673238));
#29173=CARTESIAN_POINT('Ctrl Pts',(0.71197907953204,-4.02247570412908,-28.0173751323881));
#29174=CARTESIAN_POINT('Ctrl Pts',(0.595339831784719,-4.04312087649474,
-28.0231595971429));
#29175=CARTESIAN_POINT('Ctrl Pts',(0.477643397790502,-4.05871657973845,
-28.0289440618977));
#29176=CARTESIAN_POINT('Ctrl Pts',(0.359366687456463,-4.06916214765971,
-28.0347285266525));
#29177=CARTESIAN_POINT('Ctrl Pts',(0.241205292609614,-4.07959753153247,
-28.0405073517648));
#29178=CARTESIAN_POINT('Ctrl Pts',(0.122465156075204,-4.08489273104913,
-28.046286176877));
#29179=CARTESIAN_POINT('Ctrl Pts',(0.00363196429894841,-4.08499838541404,
-28.0520650019893));
#29180=CARTESIAN_POINT('Ctrl Pts',(-0.115120392989385,-4.08510396790916,
-28.0578398961428));
#29181=CARTESIAN_POINT('Ctrl Pts',(-0.233965267613007,-4.08002702667372,
-28.0636147902964));
#29182=CARTESIAN_POINT('Ctrl Pts',(-0.352413915646341,-4.06977019401081,
-28.06938968445));
#29183=CARTESIAN_POINT('Ctrl Pts',(-0.470820428073106,-4.05951700999965,
-28.0751625243068));
#29184=CARTESIAN_POINT('Ctrl Pts',(-0.588830582873998,-4.04408763321666,
-28.0809353641637));
#29185=CARTESIAN_POINT('Ctrl Pts',(-0.705958295995525,-4.02353673828326,
-28.0867082040205));
#29186=CARTESIAN_POINT('Ctrl Pts',(-0.823072782862149,-4.00298816399088,
-28.0924803919987));
#29187=CARTESIAN_POINT('Ctrl Pts',(-0.939304619208435,-3.97731929313919,
-28.098252579977));
#29188=CARTESIAN_POINT('Ctrl Pts',(-1.05417618725878,-3.94663623434141,
-28.1040247679552));
#29189=CARTESIAN_POINT('Ctrl Pts',(-1.16906267583302,-3.91594919015961,
-28.1097977056757));
#29190=CARTESIAN_POINT('Ctrl Pts',(-1.28258814568584,-3.88024677034843,
-28.1155706433962));
#29191=CARTESIAN_POINT('Ctrl Pts',(-1.39428914366026,-3.83968524541676,
-28.1213435811166));
#29192=CARTESIAN_POINT('Ctrl Pts',(-1.50609908259559,-3.79908416120108,
-28.1271221491305));
#29193=CARTESIAN_POINT('Ctrl Pts',(-1.61608060651625,-3.75361464786899,
-28.1329007171443));
#29194=CARTESIAN_POINT('Ctrl Pts',(-1.7237891450077,-3.70348160297221,-28.1386792851581));
#29195=CARTESIAN_POINT('Ctrl Pts',(-1.83155109714163,-3.65332369664314,
-28.1444607188162));
#29196=CARTESIAN_POINT('Ctrl Pts',(-1.9370374518408,-3.59849784256731,-28.1502421524744));
#29197=CARTESIAN_POINT('Ctrl Pts',(-2.03982878353896,-3.53925465795356,
-28.1560235861326));
#29198=CARTESIAN_POINT('Ctrl Pts',(-2.14278062254969,-3.47991896588618,
-28.1618140474234));
#29199=CARTESIAN_POINT('Ctrl Pts',(-2.24302868230147,-3.41615238495911,
-28.1676045087141));
#29200=CARTESIAN_POINT('Ctrl Pts',(-2.34018264791322,-3.34824882205697,
-28.1733949700049));
#29201=CARTESIAN_POINT('Ctrl Pts',(-2.42368245807194,-3.28988852172617,
-28.1783716316931));
#29202=CARTESIAN_POINT('Ctrl Pts',(-2.50489715596483,-3.22847315025996,
-28.1833482933813));
#29203=CARTESIAN_POINT('Ctrl Pts',(-2.58359992194831,-3.16421182023402,
-28.1883249550694));
#29204=CARTESIAN_POINT('Ctrl Pts',(-2.67469731745531,-3.08983019305706,
-28.1940853741912));
#29205=CARTESIAN_POINT('Ctrl Pts',(-2.76273867255094,-3.01138150679804,
-28.199845793313));
#29206=CARTESIAN_POINT('Ctrl Pts',(-2.84733401246239,-2.92914902684633,
-28.2056062124348));
#29207=CARTESIAN_POINT('Ctrl Pts',(-2.9318248531792,-2.84701812728827,-28.2113595158082));
#29208=CARTESIAN_POINT('Ctrl Pts',(-3.01287784470125,-2.76111301561177,
-28.2171128191815));
#29209=CARTESIAN_POINT('Ctrl Pts',(-3.09013500250625,-2.67175797299937,
-28.2228661225549));
#29210=CARTESIAN_POINT('Ctrl Pts',(-3.16944536336043,-2.58002821131674,
-28.2287723269715));
#29211=CARTESIAN_POINT('Ctrl Pts',(-3.2447549366599,-2.48466283089649,-28.2346785313882));
#29212=CARTESIAN_POINT('Ctrl Pts',(-3.31571541134042,-2.38605454904108,
-28.2405847358048));
#29213=CARTESIAN_POINT('Ctrl Pts',(-3.38472557811072,-2.29015645920428,
-28.2463286115836));
#29214=CARTESIAN_POINT('Ctrl Pts',(-3.44962232801767,-2.19119176343797,
-28.2520724873625));
#29215=CARTESIAN_POINT('Ctrl Pts',(-3.5101256581818,-2.0895556618032,-28.2578163631413));
#29216=CARTESIAN_POINT('Ctrl Pts',(-3.5706092748088,-1.98795267581772,-28.263558367418));
#29217=CARTESIAN_POINT('Ctrl Pts',(-3.62670210361944,-1.8836803731514,-28.2693003716948));
#29218=CARTESIAN_POINT('Ctrl Pts',(-3.67816803242041,-1.77716204249375,
-28.2750423759715));
#29219=CARTESIAN_POINT('Ctrl Pts',(-3.72963000019004,-1.67065190992864,
-28.2807839383198));
#29220=CARTESIAN_POINT('Ctrl Pts',(-3.7764655949168,-1.56189646994867,-28.286525500668));
#29221=CARTESIAN_POINT('Ctrl Pts',(-3.81848550066746,-1.45134195873763,
-28.2922670630163));
#29222=CARTESIAN_POINT('Ctrl Pts',(-3.86260901195734,-1.3352528543852,-28.2982960601445));
#29223=CARTESIAN_POINT('Ctrl Pts',(-3.90142197438789,-1.2171803472074,-28.3043250572726));
#29224=CARTESIAN_POINT('Ctrl Pts',(-3.93476355908691,-1.09766148428454,
-28.3103540544008));
#29225=CARTESIAN_POINT('Ctrl Pts',(-3.96655034192614,-0.983716086211329,
-28.316101904246));
#29226=CARTESIAN_POINT('Ctrl Pts',(-3.99336447619579,-0.868456616329263,
-28.3218497540911));
#29227=CARTESIAN_POINT('Ctrl Pts',(-4.0151189006144,-0.75235976362975,-28.3275976039363));
#29228=CARTESIAN_POINT('Ctrl Pts',(-4.03688549258311,-0.636197976356727,
-28.3333486686334));
#29229=CARTESIAN_POINT('Ctrl Pts',(-4.0535866823057,-0.51919828700352,-28.3390997333304));
#29230=CARTESIAN_POINT('Ctrl Pts',(-4.06518723530116,-0.401842931933019,
-28.3448507980274));
#29231=CARTESIAN_POINT('Ctrl Pts',(-4.07680234166089,-0.284340349809415,
-28.3506090776683));
#29232=CARTESIAN_POINT('Ctrl Pts',(-4.0833040231341,-0.166481627636198,
-28.3563673573093));
#29233=CARTESIAN_POINT('Ctrl Pts',(-4.08470910919766,-0.0487492896119779,
-28.3621256369502));
#29234=CARTESIAN_POINT('Ctrl Pts',(-4.08491158920137,-0.0317834646288076,
-28.3629554341515));
#29235=CARTESIAN_POINT('Ctrl Pts',(-4.085008319848,-0.0148202553170852,
-28.3637852313528));
#29236=CARTESIAN_POINT('Ctrl Pts',(-4.08499944003493,0.00213890492626079,
-28.3646150285541));
#29237=CARTESIAN_POINT('Ctrl Pts',(-4.08499944003449,0.00213890577315302,
-28.3646150285955));
#29238=CARTESIAN_POINT('Ctrl Pts',(-4.08492707917895,0.140337632456191,
-28.3713769740561));
#29239=CARTESIAN_POINT('Ctrl Pts',(-4.07784209632971,0.278340655571587,
-28.3781389195167));
#29240=CARTESIAN_POINT('Ctrl Pts',(-4.06380108016489,0.415626973199183,
-28.3849008649773));
#29241=CARTESIAN_POINT('Ctrl Pts',(-4.05171852571603,0.533764392054479,
-28.3907196442771));
#29242=CARTESIAN_POINT('Ctrl Pts',(-4.03446041943139,0.651567788878492,
-28.3965384235768));
#29243=CARTESIAN_POINT('Ctrl Pts',(-4.01205176362136,0.768547751296376,
-28.4023572028766));
#29244=CARTESIAN_POINT('Ctrl Pts',(-3.98967159419813,0.885379006157445,
-28.4081685852134));
#29245=CARTESIAN_POINT('Ctrl Pts',(-3.96215397380015,1.00138851032704,-28.4139799675502));
#29246=CARTESIAN_POINT('Ctrl Pts',(-3.92957571838599,1.11609124782484,-28.419791349887));
#29247=CARTESIAN_POINT('Ctrl Pts',(-3.89703034532761,1.23067821189725,-28.4255968665953));
#29248=CARTESIAN_POINT('Ctrl Pts',(-3.85943460944823,1.34396064186545,-28.4314023833036));
#29249=CARTESIAN_POINT('Ctrl Pts',(-3.8169163835786,1.45546361025252,-28.437207900012));
#29250=CARTESIAN_POINT('Ctrl Pts',(-3.77289175927167,1.57091707031454,-28.4432191031317));
#29251=CARTESIAN_POINT('Ctrl Pts',(-3.72358945971961,1.68446220186831,-28.4492303062514));
#29252=CARTESIAN_POINT('Ctrl Pts',(-3.6692079963623,1.79558839365567,-28.4552415093711));
#29253=CARTESIAN_POINT('Ctrl Pts',(-3.61674721143371,1.90278976131629,-28.4610404050712));
#29254=CARTESIAN_POINT('Ctrl Pts',(-3.55956016589634,2.00773976713687,-28.4668393007712));
#29255=CARTESIAN_POINT('Ctrl Pts',(-3.49787380820038,2.11000090566468,-28.4726381964713));
#29256=CARTESIAN_POINT('Ctrl Pts',(-3.43619685151291,2.21224645958241,-28.4784362084189));
#29257=CARTESIAN_POINT('Ctrl Pts',(-3.37002215752528,2.31180361090308,-28.4842342203666));
#29258=CARTESIAN_POINT('Ctrl Pts',(-3.29962169624125,2.40826112821969,-28.4900322323142));
#29259=CARTESIAN_POINT('Ctrl Pts',(-3.22921527113157,2.50472681673015,-28.4958307354281));
#29260=CARTESIAN_POINT('Ctrl Pts',(-3.15458260825463,2.59809201874398,-28.501629238542));
#29261=CARTESIAN_POINT('Ctrl Pts',(-3.0760375138906,2.68797660204433,-28.5074277416559));
#29262=CARTESIAN_POINT('Ctrl Pts',(-2.99746714174169,2.777890112462,-28.5132281108738));
#29263=CARTESIAN_POINT('Ctrl Pts',(-2.91498210321149,2.86432046866093,-28.5190284800917));
#29264=CARTESIAN_POINT('Ctrl Pts',(-2.82893432733294,2.94692306849658,-28.5248288493096));
#29265=CARTESIAN_POINT('Ctrl Pts',(-2.74279167424872,3.02961674684965,-28.5306356140772));
#29266=CARTESIAN_POINT('Ctrl Pts',(-2.65307873813565,3.10847396111878,-28.5364423788448));
#29267=CARTESIAN_POINT('Ctrl Pts',(-2.56018201574489,3.18318913139896,-28.5422491436123));
#29268=CARTESIAN_POINT('Ctrl Pts',(-2.46722428548866,3.25795336921283,-28.5480597218441));
#29269=CARTESIAN_POINT('Ctrl Pts',(-2.37107893407291,3.32856990437002,-28.5538703000758));
#29270=CARTESIAN_POINT('Ctrl Pts',(-2.27216165718837,3.39477634073336,-28.5596808783076));
#29271=CARTESIAN_POINT('Ctrl Pts',(-2.17310342341672,3.46107712111294,-28.5654997365996));
#29272=CARTESIAN_POINT('Ctrl Pts',(-2.07126572900084,3.52295504848583,-28.5713185948917));
#29273=CARTESIAN_POINT('Ctrl Pts',(-1.96708915965088,3.58019346376477,-28.5771374531838));
#29274=CARTESIAN_POINT('Ctrl Pts',(-1.94119314904434,3.5944216785967,-28.5785838937509));
#29275=CARTESIAN_POINT('Ctrl Pts',(-1.91515271299772,3.60836344604473,-28.580030334318));
#29276=CARTESIAN_POINT('Ctrl Pts',(-1.88897479802175,3.6220159044983,-28.5814767748851));
#29277=CARTESIAN_POINT('Ctrl Pts',(-1.78352022539363,3.67701318647691,-28.587303586225));
#29278=CARTESIAN_POINT('Ctrl Pts',(-1.67549364854706,3.72748889979843,-28.5931303975648));
#29279=CARTESIAN_POINT('Ctrl Pts',(-1.56531918384874,3.77319504567086,-28.5989572089047));
#29280=CARTESIAN_POINT('Ctrl Pts',(-1.45528287044541,3.81884387914101,-28.6047767138189));
#29281=CARTESIAN_POINT('Ctrl Pts',(-1.34310439969314,3.859734886133,-28.6105962187331));
#29282=CARTESIAN_POINT('Ctrl Pts',(-1.2292325975245,3.8956658251425,-28.6164157236474));
#29283=CARTESIAN_POINT('Ctrl Pts',(-1.11547400212432,3.93156104305672,-28.6222294430437));
#29284=CARTESIAN_POINT('Ctrl Pts',(-1.00002581111627,3.96250588109683,-28.6280431624401));
#29285=CARTESIAN_POINT('Ctrl Pts',(-0.883356399224285,3.98834633299937,
-28.6338568818365));
#29286=CARTESIAN_POINT('Ctrl Pts',(-0.762784994606225,4.01505101532637,
-28.639865040293));
#29287=CARTESIAN_POINT('Ctrl Pts',(-0.640909659491408,4.03630372418732,
-28.6458731987495));
#29288=CARTESIAN_POINT('Ctrl Pts',(-0.518264356245074,4.05199050554735,
-28.651881357206));
#29289=CARTESIAN_POINT('Ctrl Pts',(-0.399720308404025,4.06715272139088,
-28.657688603017));
#29290=CARTESIAN_POINT('Ctrl Pts',(-0.280457401269083,4.0771152535832,-28.6634958488279));
#29291=CARTESIAN_POINT('Ctrl Pts',(-0.160967062866826,4.08182736095882,
-28.6693030946388));
#29292=CARTESIAN_POINT('Ctrl Pts',(-0.041494082617508,4.08653878381482,
-28.6751094968412));
#29293=CARTESIAN_POINT('Ctrl Pts',(0.078205855823146,4.08600128267971,-28.6809158990437));
#29294=CARTESIAN_POINT('Ctrl Pts',(0.197638558319185,4.08021617077643,-28.6867223012462));
#29295=CARTESIAN_POINT('Ctrl Pts',(0.317082004084967,4.07443053848791,-28.692529225749));
#29296=CARTESIAN_POINT('Ctrl Pts',(0.43625775877849,4.0633963766382,-28.6983361502518));
#29297=CARTESIAN_POINT('Ctrl Pts',(0.554674625996545,4.04716704118765,-28.7041430747546));
#29298=CARTESIAN_POINT('Ctrl Pts',(0.673129998971635,4.03093242842431,-28.7099518875022));
#29299=CARTESIAN_POINT('Ctrl Pts',(0.790825589889218,4.00949933765131,-28.7157607002497));
#29300=CARTESIAN_POINT('Ctrl Pts',(0.907278924941074,3.98297250208406,-28.7215695129973));
#29301=CARTESIAN_POINT('Ctrl Pts',(1.02386029044877,3.95641650253582,-28.7273847120363));
#29302=CARTESIAN_POINT('Ctrl Pts',(1.13919627614658,3.92475567064944,-28.7331999110754));
#29303=CARTESIAN_POINT('Ctrl Pts',(1.2528179897162,3.88814506990717,-28.7390151101144));
#29304=CARTESIAN_POINT('Ctrl Pts',(1.36651429963588,3.8515104331149,-28.7448341270207));
#29305=CARTESIAN_POINT('Ctrl Pts',(1.47849371455021,3.80991969708604,-28.7506531439271));
#29306=CARTESIAN_POINT('Ctrl Pts',(1.58830733071757,3.76357606847382,-28.7564721608334));
#29307=CARTESIAN_POINT('Ctrl Pts',(1.69827612786726,3.71716695026145,-28.7622994007706));
#29308=CARTESIAN_POINT('Ctrl Pts',(1.80607265072477,3.6659917084866,-28.7681266407079));
#29309=CARTESIAN_POINT('Ctrl Pts',(1.911272482402,3.61029950253617,-28.7739538806451));
#29310=CARTESIAN_POINT('Ctrl Pts',(1.93593787637183,3.5972417801148,-28.7753201486944));
#29311=CARTESIAN_POINT('Ctrl Pts',(1.96046065045553,3.58393593536615,-28.7766864167436));
#29312=CARTESIAN_POINT('Ctrl Pts',(1.98483557515258,3.57038551694474,-28.7780526847929));
#29313=CARTESIAN_POINT('Ctrl Pts',(2.08876992332173,3.51260671665906,-28.7838784332163));
#29314=CARTESIAN_POINT('Ctrl Pts',(2.19034481944784,3.45019380377238,-28.7897041816397));
#29315=CARTESIAN_POINT('Ctrl Pts',(2.2891200188456,3.38336438169469,-28.7955299300632));
#29316=CARTESIAN_POINT('Ctrl Pts',(2.35644383584311,3.33781436702057,-28.7995006800401));
#29317=CARTESIAN_POINT('Ctrl Pts',(2.42246738896646,3.2902136388328,-28.8034714300171));
#29318=CARTESIAN_POINT('Ctrl Pts',(2.48705727606859,3.24064362520075,-28.807442179994));
#29319=CARTESIAN_POINT('Origin',(0.,0.,0.));
#29320=CARTESIAN_POINT('',(-1.30343164629623,3.1291326283706,-38.999956889224));
#29321=CARTESIAN_POINT('',(-2.89372837779137,-1.76542944862289,-39.));
#29322=CARTESIAN_POINT('Origin',(0.,0.,-39.));
#29323=CARTESIAN_POINT('',(-3.38974897938027,0.00263045440945954,-38.7660178032496));
#29324=CARTESIAN_POINT('Ctrl Pts',(-1.30343164629623,3.1291326283706,-38.999956889224));
#29325=CARTESIAN_POINT('Ctrl Pts',(-1.39833027824498,3.08960286253366,-38.99388871478));
#29326=CARTESIAN_POINT('Ctrl Pts',(-1.49159532416278,3.04568278774804,-38.987820540336));
#29327=CARTESIAN_POINT('Ctrl Pts',(-1.58278977870312,2.9975292457177,-38.9817523658921));
#29328=CARTESIAN_POINT('Ctrl Pts',(-1.67386612085234,2.94943807074705,-38.9756920507702));
#29329=CARTESIAN_POINT('Ctrl Pts',(-1.76287682226379,2.89712452704605,-38.9696317356483));
#29330=CARTESIAN_POINT('Ctrl Pts',(-1.84940424216492,2.84079372914726,-38.9635714205265));
#29331=CARTESIAN_POINT('Ctrl Pts',(-1.93976809019622,2.78196535235498,-38.9572424048767));
#29332=CARTESIAN_POINT('Ctrl Pts',(-2.02742291519195,2.71875542496574,-38.9509133892268));
#29333=CARTESIAN_POINT('Ctrl Pts',(-2.11192072102072,2.65145166477221,-38.944584373577));
#29334=CARTESIAN_POINT('Ctrl Pts',(-2.19269466403182,2.5871140167471,-38.9385342809811));
#29335=CARTESIAN_POINT('Ctrl Pts',(-2.2705835622744,2.51903600965155,-38.9324841883852));
#29336=CARTESIAN_POINT('Ctrl Pts',(-2.34522613869442,2.44751290515177,-38.9264340957893));
#29337=CARTESIAN_POINT('Ctrl Pts',(-2.41984501993697,2.37601250555763,-38.9203859237864));
#29338=CARTESIAN_POINT('Ctrl Pts',(-2.49121931485692,2.30106948112322,-38.9143377517836));
#29339=CARTESIAN_POINT('Ctrl Pts',(-2.55902268804625,2.2230177562414,-38.9082895797808));
#29340=CARTESIAN_POINT('Ctrl Pts',(-2.62682261012922,2.14497000409414,-38.9022417156224));
#29341=CARTESIAN_POINT('Ctrl Pts',(-2.69105168836955,2.06381419339159,-38.8961938514639));
#29342=CARTESIAN_POINT('Ctrl Pts',(-2.75142282563774,1.9799185581886,-38.8901459873054));
#29343=CARTESIAN_POINT('Ctrl Pts',(-2.81180698217444,1.89600483056843,-38.8840968189018));
#29344=CARTESIAN_POINT('Ctrl Pts',(-2.86833129250096,1.80935045635071,-38.8780476504981));
#29345=CARTESIAN_POINT('Ctrl Pts',(-2.92075163866745,1.72035314041083,-38.8719984820944));
#29346=CARTESIAN_POINT('Ctrl Pts',(-2.97322659162087,1.63126311509713,-38.8659430122128));
#29347=CARTESIAN_POINT('Ctrl Pts',(-3.02158882850242,1.53982565066671,-38.8598875423313));
#29348=CARTESIAN_POINT('Ctrl Pts',(-3.0656400215595,1.44646338381332,-38.8538320724498));
#29349=CARTESIAN_POINT('Ctrl Pts',(-3.10971820406863,1.35304391541214,-38.84777289248));
#29350=CARTESIAN_POINT('Ctrl Pts',(-3.14947991874989,1.25769769613465,-38.8417137125102));
#29351=CARTESIAN_POINT('Ctrl Pts',(-3.18477558775203,1.16086584847635,-38.8356545325404));
#29352=CARTESIAN_POINT('Ctrl Pts',(-3.22012294762422,1.06389218958184,-38.8295864788393));
#29353=CARTESIAN_POINT('Ctrl Pts',(-3.25099108070739,0.965428972501001,
-38.8235184251381));
#29354=CARTESIAN_POINT('Ctrl Pts',(-3.27728073635541,0.865930734882268,
-38.817450371437));
#29355=CARTESIAN_POINT('Ctrl Pts',(-3.28562121105491,0.834364610752882,
-38.8155252626015));
#29356=CARTESIAN_POINT('Ctrl Pts',(-3.29350125325975,0.802694372619393,
-38.813600153766));
#29357=CARTESIAN_POINT('Ctrl Pts',(-3.30091878121429,0.770934668001608,
-38.8116750449306));
#29358=CARTESIAN_POINT('Ctrl Pts',(-3.33201007028159,0.637810780499659,
-38.8036057642138));
#29359=CARTESIAN_POINT('Ctrl Pts',(-3.35505703564748,0.5027501102116,-38.7955364834971));
#29360=CARTESIAN_POINT('Ctrl Pts',(-3.36986949869865,0.366585084585444,
-38.7874672027803));
#29361=CARTESIAN_POINT('Ctrl Pts',(-3.3829941066685,0.245935833048101,-38.7803174029367));
#29362=CARTESIAN_POINT('Ctrl Pts',(-3.38965447070927,0.12441955287756,-38.7731676030932));
#29363=CARTESIAN_POINT('Ctrl Pts',(-3.38974897938027,0.00263045440945954,
-38.7660178032496));
#29364=CARTESIAN_POINT('',(-3.38517229864742,-0.00153545903651936,-37.5160178032496));
#29365=CARTESIAN_POINT('Ctrl Pts',(-3.38956806600938,0.0026303140201922,
-38.7660178032496));
#29366=CARTESIAN_POINT('Ctrl Pts',(-3.38196169697795,-0.854242402898206,
-38.7157115805073));
#29367=CARTESIAN_POINT('Ctrl Pts',(-2.62050801171528,-2.83865004984225,
-38.5998800544626));
#29368=CARTESIAN_POINT('Ctrl Pts',(0.699092616145842,-3.93244007385531,
-38.4185232251148));
#29369=CARTESIAN_POINT('Ctrl Pts',(3.66779171704377,-1.58009583571682,-38.2219473152072));
#29370=CARTESIAN_POINT('Ctrl Pts',(3.33787025741108,2.1929856073312,-38.0253714052993));
#29371=CARTESIAN_POINT('Ctrl Pts',(0.00554946209745111,3.99384108558651,
-37.8287954953915));
#29372=CARTESIAN_POINT('Ctrl Pts',(-2.87684185453993,2.44650803385519,-37.659010961375));
#29373=CARTESIAN_POINT('Ctrl Pts',(-3.38241331840635,0.660535797814238,
-37.5547517306609));
#29374=CARTESIAN_POINT('Ctrl Pts',(-3.38517229864742,-0.00153545903651936,
-37.5160178032496));
#29375=CARTESIAN_POINT('',(-3.38974885847844,0.0027818957803985,-35.0146790786306));
#29376=CARTESIAN_POINT('Ctrl Pts',(-3.38974971482863,-0.00139043850725259,
-37.5133796950408));
#29377=CARTESIAN_POINT('Ctrl Pts',(-3.38963540845987,-0.280057908424469,
-37.4978425875729));
#29378=CARTESIAN_POINT('Ctrl Pts',(-3.35516103288601,-0.557648974801886,
-37.4833830197543));
#29379=CARTESIAN_POINT('Ctrl Pts',(-3.25561678295251,-0.952875792877547,
-37.4615574925989));
#29380=CARTESIAN_POINT('Ctrl Pts',(-3.21704324491428,-1.07593653096365,
-37.4545556953373));
#29381=CARTESIAN_POINT('Ctrl Pts',(-3.16085149518451,-1.22488526578853,
-37.4455004378842));
#29382=CARTESIAN_POINT('Ctrl Pts',(-3.14975886689697,-1.25313408462521,
-37.4437563425721));
#29383=CARTESIAN_POINT('Ctrl Pts',(-3.13118482705633,-1.29863000893447,
-37.4408981292982));
#29384=CARTESIAN_POINT('Ctrl Pts',(-3.12393634803657,-1.31597111737372,
-37.4397969630444));
#29385=CARTESIAN_POINT('Ctrl Pts',(-3.10909088499153,-1.35067317583879,
-37.4375680137118));
#29386=CARTESIAN_POINT('Ctrl Pts',(-3.10149179434903,-1.36803244507079,
-37.436440149866));
#29387=CARTESIAN_POINT('Ctrl Pts',(-3.08104545250067,-1.41369375209662,
-37.4334411339879));
#29388=CARTESIAN_POINT('Ctrl Pts',(-3.06795406907797,-1.44188376329372,
-37.4315565766478));
#29389=CARTESIAN_POINT('Ctrl Pts',(-2.99128261356095,-1.60120959250344,
-37.4207324475503));
#29390=CARTESIAN_POINT('Ctrl Pts',(-2.91968998855778,-1.72830749538175,
-37.4114314136678));
#29391=CARTESIAN_POINT('Ctrl Pts',(-2.73788159051288,-2.00736348670642,
-37.3900152668832));
#29392=CARTESIAN_POINT('Ctrl Pts',(-2.62276765961903,-2.15559806704704,
-37.3779037505251));
#29393=CARTESIAN_POINT('Ctrl Pts',(-2.42333512627505,-2.37263183313778,
-37.3594093966504));
#29394=CARTESIAN_POINT('Ctrl Pts',(-2.34696086604114,-2.44820613917663,
-37.3527929769091));
#29395=CARTESIAN_POINT('Ctrl Pts',(-2.23539596463779,-2.54857430955382,
-37.3437582625166));
#29396=CARTESIAN_POINT('Ctrl Pts',(-2.20313382079788,-2.5765146507674,-37.3412133491296));
#29397=CARTESIAN_POINT('Ctrl Pts',(-2.14603341260647,-2.62410896963293,
-37.3368232030854));
#29398=CARTESIAN_POINT('Ctrl Pts',(-2.12143193505007,-2.64403743127729,
-37.3349671727457));
#29399=CARTESIAN_POINT('Ctrl Pts',(-2.0696393654739,-2.68480374906934,-37.3311310704333));
#29400=CARTESIAN_POINT('Ctrl Pts',(-2.04240425341824,-2.70558002341925,
-37.3291535184971));
#29401=CARTESIAN_POINT('Ctrl Pts',(-1.96930754881953,-2.75960889653867,
-37.3239463890803));
#29402=CARTESIAN_POINT('Ctrl Pts',(-1.92291852092737,-2.79213150784517,
-37.3207442956922));
#29403=CARTESIAN_POINT('Ctrl Pts',(-1.69126127141587,-2.94602946603464,
-37.3052071942986));
#29404=CARTESIAN_POINT('Ctrl Pts',(-1.49522021485583,-3.05020996918097,
-37.2934905946234));
#29405=CARTESIAN_POINT('Ctrl Pts',(-1.17115894301394,-3.18361758405139,
-37.2748888614377));
#29406=CARTESIAN_POINT('Ctrl Pts',(-1.04921620738403,-3.2258605134561,-37.2680344628154));
#29407=CARTESIAN_POINT('Ctrl Pts',(-0.856542246070162,-3.28052274294266,
-37.2570449311983));
#29408=CARTESIAN_POINT('Ctrl Pts',(-0.787320272462905,-3.29782041749641,
-37.2530650195709));
#29409=CARTESIAN_POINT('Ctrl Pts',(-0.692464501908122,-3.31836705228204,
-37.24750650796));
#29410=CARTESIAN_POINT('Ctrl Pts',(-0.667259489825077,-3.32352699212036,
-37.2460195384264));
#29411=CARTESIAN_POINT('Ctrl Pts',(-0.624385947828445,-3.33179666432789,
-37.2434696442412));
#29412=CARTESIAN_POINT('Ctrl Pts',(-0.606747255388106,-3.33505390999365,
-37.2424146452682));
#29413=CARTESIAN_POINT('Ctrl Pts',(-0.568902731844816,-3.34173228415333,
-37.240137255103));
#29414=CARTESIAN_POINT('Ctrl Pts',(-0.548691396713423,-3.34511026448881,
-37.2389128053741));
#29415=CARTESIAN_POINT('Ctrl Pts',(-0.491488497042306,-3.35413839860511,
-37.2354266033609));
#29416=CARTESIAN_POINT('Ctrl Pts',(-0.45443327077754,-3.35935938769356,
-37.233143893227));
#29417=CARTESIAN_POINT('Ctrl Pts',(-0.278234446005362,-3.3812169021349,
-37.2221975052339));
#29418=CARTESIAN_POINT('Ctrl Pts',(-0.13824217771398,-3.38982673429237,
-37.2132344463832));
#29419=CARTESIAN_POINT('Ctrl Pts',(0.180879260881719,-3.38965078839984,
-37.1927027217061));
#29420=CARTESIAN_POINT('Ctrl Pts',(0.359613646406424,-3.37537199890944,
-37.181142917244));
#29421=CARTESIAN_POINT('Ctrl Pts',(0.643743779185407,-3.32983775579119,
-37.1630773731505));
#29422=CARTESIAN_POINT('Ctrl Pts',(0.750213658200293,-3.30747770784222,
-37.156375013297));
#29423=CARTESIAN_POINT('Ctrl Pts',(0.896894210673183,-3.2692234156588,-37.1472471643914));
#29424=CARTESIAN_POINT('Ctrl Pts',(0.938147434880559,-3.25762499498695,
-37.1446915064063));
#29425=CARTESIAN_POINT('Ctrl Pts',(1.00950729334849,-3.23609396502341,-37.1402888758628));
#29426=CARTESIAN_POINT('Ctrl Pts',(1.039714347059,-3.22651565982465,-37.1384309341173));
#29427=CARTESIAN_POINT('Ctrl Pts',(1.10222659122524,-3.20572465957939,-37.1345963158099));
#29428=CARTESIAN_POINT('Ctrl Pts',(1.13450544613777,-3.19444385877272,-37.132622076957));
#29429=CARTESIAN_POINT('Ctrl Pts',(1.21948563729376,-3.1632943971537,-37.1274364308162));
#29430=CARTESIAN_POINT('Ctrl Pts',(1.27187298856821,-3.14259705765547,-37.1242520709946));
#29431=CARTESIAN_POINT('Ctrl Pts',(1.53312660093978,-3.0317764030757,-37.1083940019937));
#29432=CARTESIAN_POINT('Ctrl Pts',(1.73306040307067,-2.92209806939385,-37.096379427684));
#29433=CARTESIAN_POINT('Ctrl Pts',(2.02362355231975,-2.72231711417247,-37.0776567639117));
#29434=CARTESIAN_POINT('Ctrl Pts',(2.12272344425099,-2.64577108350339,-37.0709964134981));
#29435=CARTESIAN_POINT('Ctrl Pts',(2.27038593574331,-2.51806823261727,-37.0602758875193));
#29436=CARTESIAN_POINT('Ctrl Pts',(2.3219736320467,-2.47057828583941,-37.0563619986539));
#29437=CARTESIAN_POINT('Ctrl Pts',(2.39032007572925,-2.40362834051028,-37.050881193941));
#29438=CARTESIAN_POINT('Ctrl Pts',(2.40838795298934,-2.38552439665988,-37.0494025962997));
#29439=CARTESIAN_POINT('Ctrl Pts',(2.4387613683404,-2.35439357229379,-37.0468622450008));
#29440=CARTESIAN_POINT('Ctrl Pts',(2.45117145587889,-2.3414706038599,-37.0458082567081));
#29441=CARTESIAN_POINT('Ctrl Pts',(2.4776081814976,-2.31350077822359,-37.0435271392372));
#29442=CARTESIAN_POINT('Ctrl Pts',(2.49160055708871,-2.29842440999425,-37.0422978618386));
#29443=CARTESIAN_POINT('Ctrl Pts',(2.53090583014691,-2.25529344460598,-37.0387843399938));
#29444=CARTESIAN_POINT('Ctrl Pts',(2.55588732691935,-2.22694242434155,-37.0364786491366));
#29445=CARTESIAN_POINT('Ctrl Pts',(2.67702066273505,-2.08474709737769,-37.024958165882));
#29446=CARTESIAN_POINT('Ctrl Pts',(2.7660607728452,-1.96507283719963,-37.0154051702325));
#29447=CARTESIAN_POINT('Ctrl Pts',(2.92058453359913,-1.72597881861116,-36.9970778900346));
#29448=CARTESIAN_POINT('Ctrl Pts',(2.98733039815867,-1.60769301421061,-36.9883260596764));
#29449=CARTESIAN_POINT('Ctrl Pts',(3.08689678282724,-1.40350959963229,-36.9739255933961));
#29450=CARTESIAN_POINT('Ctrl Pts',(3.12364412436115,-1.31970463846546,-36.9681994225809));
#29451=CARTESIAN_POINT('Ctrl Pts',(3.18206775740662,-1.17030049618221,-36.958332226596));
#29452=CARTESIAN_POINT('Ctrl Pts',(3.20521317281995,-1.10533614854875,-36.9541500786922));
#29453=CARTESIAN_POINT('Ctrl Pts',(3.23760283507773,-1.00482634346251,-36.9478416790135));
#29454=CARTESIAN_POINT('Ctrl Pts',(3.24827728849505,-0.969764359213442,
-36.9456705258882));
#29455=CARTESIAN_POINT('Ctrl Pts',(3.26612683571896,-0.907529530516667,
-36.9418669513655));
#29456=CARTESIAN_POINT('Ctrl Pts',(3.27353642503602,-0.880428134212425,
-36.9402272215186));
#29457=CARTESIAN_POINT('Ctrl Pts',(3.28994593809484,-0.817335256605636,
-36.9364468937442));
#29458=CARTESIAN_POINT('Ctrl Pts',(3.2986937525358,-0.781281561849035,-36.9343144044559));
#29459=CARTESIAN_POINT('Ctrl Pts',(3.32205393578808,-0.67760478434035,-36.928256036336));
#29460=CARTESIAN_POINT('Ctrl Pts',(3.33519086007305,-0.609666638926558,
-36.9243757263973));
#29461=CARTESIAN_POINT('Ctrl Pts',(3.38593130831218,-0.296037321377273,
-36.9067957535624));
#29462=CARTESIAN_POINT('Ctrl Pts',(3.39852253502943,-0.0470894588677387,
-36.8938370785724));
#29463=CARTESIAN_POINT('Ctrl Pts',(3.37613239024138,0.329834739874389,-36.8736691421433));
#29464=CARTESIAN_POINT('Ctrl Pts',(3.36112902024774,0.458112252655445,-36.8666926566614));
#29465=CARTESIAN_POINT('Ctrl Pts',(3.33255306525874,0.621149297998841,-36.8573479236848));
#29466=CARTESIAN_POINT('Ctrl Pts',(3.32567426244639,0.656983149682284,-36.8552638049035));
#29467=CARTESIAN_POINT('Ctrl Pts',(3.31411472531476,0.712356635612162,-36.851986628945));
#29468=CARTESIAN_POINT('Ctrl Pts',(3.30983623744387,0.731978432981562,-36.8508142461076));
#29469=CARTESIAN_POINT('Ctrl Pts',(3.30142031677509,0.76899188285912,-36.8485797427721));
#29470=CARTESIAN_POINT('Ctrl Pts',(3.2973192564117,0.786390672315879,-36.8475195568989));
#29471=CARTESIAN_POINT('Ctrl Pts',(3.28781378529916,0.825335699727807,-36.845125362408));
#29472=CARTESIAN_POINT('Ctrl Pts',(3.28233480387825,0.846862847541506,-36.8437874592787));
#29473=CARTESIAN_POINT('Ctrl Pts',(3.26195011065856,0.923784172914644,-36.8389585648473));
#29474=CARTESIAN_POINT('Ctrl Pts',(3.24585105380082,0.978849263470516,-36.835411755264));
#29475=CARTESIAN_POINT('Ctrl Pts',(3.14671399007535,1.28853281277306,-36.8150489715525));
#29476=CARTESIAN_POINT('Ctrl Pts',(3.03512728580681,1.53301667217336,-36.7974540857716));
#29477=CARTESIAN_POINT('Ctrl Pts',(2.83127818513881,1.86808407053455,-36.7726834517822));
#29478=CARTESIAN_POINT('Ctrl Pts',(2.76082995469431,1.97070996222896,-36.7649766481907));
#29479=CARTESIAN_POINT('Ctrl Pts',(2.65764289395974,2.10459782470753,-36.7547785215423));
#29480=CARTESIAN_POINT('Ctrl Pts',(2.62969640471604,2.13941460640223,-36.7521117654725));
#29481=CARTESIAN_POINT('Ctrl Pts',(2.58057133996229,2.19819890626915,-36.7475814060649));
#29482=CARTESIAN_POINT('Ctrl Pts',(2.55972693292132,2.22243672680613,-36.7457049822149));
#29483=CARTESIAN_POINT('Ctrl Pts',(2.51630172941993,2.27150984692276,-36.7418866949192));
#29484=CARTESIAN_POINT('Ctrl Pts',(2.49368863783129,2.29631192832581,-36.7399464504953));
#29485=CARTESIAN_POINT('Ctrl Pts',(2.43431512589236,2.35952131539616,-36.7349710953629));
#29486=CARTESIAN_POINT('Ctrl Pts',(2.3970122292564,2.39740771893907,-36.7319590102458));
#29487=CARTESIAN_POINT('Ctrl Pts',(2.15088632243893,2.63589321649151,-36.712758227023));
#29488=CARTESIAN_POINT('Ctrl Pts',(1.91799292279426,2.80990251898898,-36.6977432595635));
#29489=CARTESIAN_POINT('Ctrl Pts',(1.55314974567294,3.01576933811904,-36.6753127763765));
#29490=CARTESIAN_POINT('Ctrl Pts',(1.43695196584987,3.07283282443071,-36.6682858473396));
#29491=CARTESIAN_POINT('Ctrl Pts',(1.28980836909209,3.13491975252192,-36.6592018255467));
#29492=CARTESIAN_POINT('Ctrl Pts',(1.26166959434878,3.14634981889251,-36.6574564540419));
#29493=CARTESIAN_POINT('Ctrl Pts',(1.21587004403559,3.16424059868812,-36.6545966320535));
#29494=CARTESIAN_POINT('Ctrl Pts',(1.19830180062916,3.17093539698664,-36.6534951583886));
#29495=CARTESIAN_POINT('Ctrl Pts',(1.16291816173434,3.18408313651429,-36.6512660514002));
#29496=CARTESIAN_POINT('Ctrl Pts',(1.14510257695021,3.19053351675171,-36.6501383437206));
#29497=CARTESIAN_POINT('Ctrl Pts',(1.09793790533473,3.20716423215931,-36.6471405291085));
#29498=CARTESIAN_POINT('Ctrl Pts',(1.06850196797633,3.21709083682903,-36.6452570381004));
#29499=CARTESIAN_POINT('Ctrl Pts',(0.903354215304466,3.27026668065216,-36.6346362138455));
#29500=CARTESIAN_POINT('Ctrl Pts',(0.76516796330292,3.30532962305828,-36.6255538485042));
#29501=CARTESIAN_POINT('Ctrl Pts',(0.438688555273904,3.36659606322334,-36.604201646272));
#29502=CARTESIAN_POINT('Ctrl Pts',(0.24955235674908,3.38587506471536,-36.5919267647744));
#29503=CARTESIAN_POINT('Ctrl Pts',(-0.0482586469328648,3.39112874000251,
-36.573232101153));
#29504=CARTESIAN_POINT('Ctrl Pts',(-0.156343374508001,3.38786710198308,
-36.5665717655171));
#29505=CARTESIAN_POINT('Ctrl Pts',(-0.306730355255403,3.3761146722249,-36.5574893862273));
#29506=CARTESIAN_POINT('Ctrl Pts',(-0.349298503499069,3.37197636346342,
-36.5549389206137));
#29507=CARTESIAN_POINT('Ctrl Pts',(-0.423239823571647,3.36337276156537,
-36.5505422834501));
#29508=CARTESIAN_POINT('Ctrl Pts',(-0.454649092917693,3.35927113887308,
-36.5486852265698));
#29509=CARTESIAN_POINT('Ctrl Pts',(-0.519865078520934,3.34982335021355,
-36.54484977863));
#29510=CARTESIAN_POINT('Ctrl Pts',(-0.553657688208975,3.34440420177297,
-36.5428738656095));
#29511=CARTESIAN_POINT('Ctrl Pts',(-0.642986736253272,3.32868785719603,
-36.5376775800884));
#29512=CARTESIAN_POINT('Ctrl Pts',(-0.698358870837683,3.31751265083307,
-36.5344844687493));
#29513=CARTESIAN_POINT('Ctrl Pts',(-0.972632597582847,3.25498673347624,
-36.5187668276294));
#29514=CARTESIAN_POINT('Ctrl Pts',(-1.18632412308613,3.18333127265262,-36.5068832572459));
#29515=CARTESIAN_POINT('Ctrl Pts',(-1.50697620799302,3.0389970525262,-36.4882152280711));
#29516=CARTESIAN_POINT('Ctrl Pts',(-1.61957504954803,2.98051231352566,-36.4814707004853));
#29517=CARTESIAN_POINT('Ctrl Pts',(-1.78939514211345,2.87983692166256,-36.4706332817705));
#29518=CARTESIAN_POINT('Ctrl Pts',(-1.84901829541532,2.84192288414976,-36.4666905246977));
#29519=CARTESIAN_POINT('Ctrl Pts',(-1.92860798984674,2.7877470975686,-36.4611757219193));
#29520=CARTESIAN_POINT('Ctrl Pts',(-1.94964149379764,2.77307782418434,-36.4596934336464));
#29521=CARTESIAN_POINT('Ctrl Pts',(-1.98509225644066,2.74775092645692,-36.4571488777277));
#29522=CARTESIAN_POINT('Ctrl Pts',(-1.99959488379094,2.73721513790705,-36.4560944459888));
#29523=CARTESIAN_POINT('Ctrl Pts',(-2.0305309959958,2.71436375693765,-36.4538150025067));
#29524=CARTESIAN_POINT('Ctrl Pts',(-2.04693642275421,2.70201368700692,-36.4525878825084));
#29525=CARTESIAN_POINT('Ctrl Pts',(-2.09307938011474,2.66661569695726,-36.449086528822));
#29526=CARTESIAN_POINT('Ctrl Pts',(-2.12254597947455,2.64322130772275,-36.4467910663034));
#29527=CARTESIAN_POINT('Ctrl Pts',(-2.26415715591376,2.52689713479139,-36.4354902678453));
#29528=CARTESIAN_POINT('Ctrl Pts',(-2.37061544419424,2.42730154426324,-36.4261615471792));
#29529=CARTESIAN_POINT('Ctrl Pts',(-2.56435969262928,2.2211078204855,-36.4079504145397));
#29530=CARTESIAN_POINT('Ctrl Pts',(-2.6522246367592,2.11541198741061,-36.3990894847843));
#29531=CARTESIAN_POINT('Ctrl Pts',(-2.81460296825852,1.89400395431492,-36.3816750048194));
#29532=CARTESIAN_POINT('Ctrl Pts',(-2.88897867676167,1.77849665377634,-36.3731374462106));
#29533=CARTESIAN_POINT('Ctrl Pts',(-2.97860289939383,1.61877566047522,-36.3620740851882));
#29534=CARTESIAN_POINT('Ctrl Pts',(-3.00023974070472,1.57831292113921,-36.3593305186187));
#29535=CARTESIAN_POINT('Ctrl Pts',(-3.03564331088719,1.50874455258696,-36.354710883625));
#29536=CARTESIAN_POINT('Ctrl Pts',(-3.0498285821636,1.4798601829526,-36.3528206853845));
#29537=CARTESIAN_POINT('Ctrl Pts',(-3.07781449699598,1.42076244132663,-36.3490079180979));
#29538=CARTESIAN_POINT('Ctrl Pts',(-3.09158667677173,1.39053943694513,-36.347086467368));
#29539=CARTESIAN_POINT('Ctrl Pts',(-3.12552945611725,1.31305398188221,-36.3422291699285));
#29540=CARTESIAN_POINT('Ctrl Pts',(-3.1450740137539,1.26552557359411,-36.3393141875322));
#29541=CARTESIAN_POINT('Ctrl Pts',(-3.26042524067152,0.965815988506703,
-36.3212943391837));
#29542=CARTESIAN_POINT('Ctrl Pts',(-3.32692152549007,0.703403048467539,
-36.3071956188689));
#29543=CARTESIAN_POINT('Ctrl Pts',(-3.37484868173537,0.333768330703661,
-36.2873331531732));
#29544=CARTESIAN_POINT('Ctrl Pts',(-3.38342800232922,0.231122495838761,
-36.2818043858664));
#29545=CARTESIAN_POINT('Ctrl Pts',(-3.38895531052209,0.085137740948565,
-36.2737404954765));
#29546=CARTESIAN_POINT('Ctrl Pts',(-3.38976435368707,0.0419983438670175,
-36.2713325854174));
#29547=CARTESIAN_POINT('Ctrl Pts',(-3.38973839521835,-0.0349886614083398,
-36.2669728674685));
#29548=CARTESIAN_POINT('Ctrl Pts',(-3.38922007416214,-0.0688309581393426,
-36.2650348265363));
#29549=CARTESIAN_POINT('Ctrl Pts',(-3.38760352429533,-0.12218444861052,
-36.2619376108225));
#29550=CARTESIAN_POINT('Ctrl Pts',(-3.38684314440264,-0.141704452383818,
-36.2607956163946));
#29551=CARTESIAN_POINT('Ctrl Pts',(-3.38504113885493,-0.179550731973185,
-36.2585624594746));
#29552=CARTESIAN_POINT('Ctrl Pts',(-3.38401930001063,-0.197876979546816,
-36.2574723222941));
#29553=CARTESIAN_POINT('Ctrl Pts',(-3.38105278745011,-0.2442949827133,-36.2546903034723));
#29554=CARTESIAN_POINT('Ctrl Pts',(-3.37890681710992,-0.27237216931501,
-36.2529881945179));
#29555=CARTESIAN_POINT('Ctrl Pts',(-3.36799641371311,-0.394994544287951,
-36.245479299598));
#29556=CARTESIAN_POINT('Ctrl Pts',(-3.35561202683189,-0.489168258874862,
-36.2395175926695));
#29557=CARTESIAN_POINT('Ctrl Pts',(-3.29921295692525,-0.812381407571793,
-36.2186386217596));
#29558=CARTESIAN_POINT('Ctrl Pts',(-3.23553595440599,-1.03734737911403,
-36.2034229629017));
#29559=CARTESIAN_POINT('Ctrl Pts',(-3.10719430582373,-1.35966359966522,
-36.1815814961799));
#29560=CARTESIAN_POINT('Ctrl Pts',(-3.05982341694822,-1.46315634725182,
-36.1745508426855));
#29561=CARTESIAN_POINT('Ctrl Pts',(-2.98679581922174,-1.60357009832929,
-36.1650036378923));
#29562=CARTESIAN_POINT('Ctrl Pts',(-2.96548110509562,-1.64265286118646,
-36.1623448312114));
#29563=CARTESIAN_POINT('Ctrl Pts',(-2.92771424475063,-1.70876995032401,
-36.1578423493469));
#29564=CARTESIAN_POINT('Ctrl Pts',(-2.91164247062311,-1.73601372854303,
-36.1559857128867));
#29565=CARTESIAN_POINT('Ctrl Pts',(-2.87775686237685,-1.79165961057409,
-36.1521890920382));
#29566=CARTESIAN_POINT('Ctrl Pts',(-2.85989824314657,-1.82003045964922,
-36.150250977227));
#29567=CARTESIAN_POINT('Ctrl Pts',(-2.81274790603219,-1.89252710178116,
-36.1452889876274));
#29568=CARTESIAN_POINT('Ctrl Pts',(-2.78283716256883,-1.93624052328844,
-36.1422878896269));
#29569=CARTESIAN_POINT('Ctrl Pts',(-2.61171169171275,-2.17417184715629,
-36.125865148514));
#29570=CARTESIAN_POINT('Ctrl Pts',(-2.4511953361399,-2.35365964699743,-36.1132062187244));
#29571=CARTESIAN_POINT('Ctrl Pts',(-2.1516137921046,-2.62445375285005,-36.0917555682986));
#29572=CARTESIAN_POINT('Ctrl Pts',(-2.02240006915864,-2.72526829712647,
-36.0830245805293));
#29573=CARTESIAN_POINT('Ctrl Pts',(-1.85443367684918,-2.83777438219757,
-36.0716417696793));
#29574=CARTESIAN_POINT('Ctrl Pts',(-1.82208061079064,-2.8586552249444,-36.0694474577999));
#29575=CARTESIAN_POINT('Ctrl Pts',(-1.77178215599723,-2.88991736675737,
-36.0660221020505));
#29576=CARTESIAN_POINT('Ctrl Pts',(-1.75408454353289,-2.90069332427577,
-36.0648142893501));
#29577=CARTESIAN_POINT('Ctrl Pts',(-1.72093607994034,-2.92046291783851,
-36.0625450703752));
#29578=CARTESIAN_POINT('Ctrl Pts',(-1.70551117556095,-2.92949760569601,
-36.0614861976795));
#29579=CARTESIAN_POINT('Ctrl Pts',(-1.66809839286833,-2.95101543464584,
-36.0589116005543));
#29580=CARTESIAN_POINT('Ctrl Pts',(-1.64604126486683,-2.96337517275562,
-36.0573886523304));
#29581=CARTESIAN_POINT('Ctrl Pts',(-1.56432258236601,-3.00797250833878,
-36.0517335326194));
#29582=CARTESIAN_POINT('Ctrl Pts',(-1.50383885698185,-3.03866273527339,
-36.0475232784955));
#29583=CARTESIAN_POINT('Ctrl Pts',(-1.33544950623357,-3.1178467429777,-36.0358126086579));
#29584=CARTESIAN_POINT('Ctrl Pts',(-1.22586271860974,-3.16253885004161,
-36.0282057087537));
#29585=CARTESIAN_POINT('Ctrl Pts',(-0.888254867450782,-3.2800347041917,
-36.0051825609125));
#29586=CARTESIAN_POINT('Ctrl Pts',(-0.654618483524561,-3.33453609092645,
-35.9898530327583));
#29587=CARTESIAN_POINT('Ctrl Pts',(-0.362261221123828,-3.37079110216086,
-35.971908066701));
#29588=CARTESIAN_POINT('Ctrl Pts',(-0.307196747023287,-3.37625480977194,
-35.9685774097085));
#29589=CARTESIAN_POINT('Ctrl Pts',(-0.218123255140295,-3.38289561332583,
-35.9632665174595));
#29590=CARTESIAN_POINT('Ctrl Pts',(-0.184188855582638,-3.38491286087705,
-35.9612611032613));
#29591=CARTESIAN_POINT('Ctrl Pts',(-0.11849771889123,-3.38782706213647,
-35.9574119329923));
#29592=CARTESIAN_POINT('Ctrl Pts',(-0.0867475641552904,-3.38878870282408,
-35.9555663972429));
#29593=CARTESIAN_POINT('Ctrl Pts',(-0.0116322428499328,-3.39000736728844,
-35.9512330582839));
#29594=CARTESIAN_POINT('Ctrl Pts',(0.0317340902763956,-3.38987882492134,
-35.9487572233508));
#29595=CARTESIAN_POINT('Ctrl Pts',(0.187992105544546,-3.38641665289971,
-35.9399180038886));
#29596=CARTESIAN_POINT('Ctrl Pts',(0.300707005503613,-3.37827431458885,
-35.9336987043895));
#29597=CARTESIAN_POINT('Ctrl Pts',(0.619594829507402,-3.33914804678742,
-35.9163039542508));
#29598=CARTESIAN_POINT('Ctrl Pts',(0.823591161485063,-3.2947690859119,-35.9054385378855));
#29599=CARTESIAN_POINT('Ctrl Pts',(1.13570417907403,-3.1960519131598,-35.8878626376712));
#29600=CARTESIAN_POINT('Ctrl Pts',(1.24720835052323,-3.15420957655838,-35.8813723102588));
#29601=CARTESIAN_POINT('Ctrl Pts',(1.38404174785385,-3.09447115720145,-35.8728790888058));
#29602=CARTESIAN_POINT('Ctrl Pts',(1.41164814078924,-3.08197545324783,-35.8711375438792));
#29603=CARTESIAN_POINT('Ctrl Pts',(1.45609166648871,-3.06113623517513,-35.8682824142993));
#29604=CARTESIAN_POINT('Ctrl Pts',(1.47303406830883,-3.05301958604326,-35.8671817266046));
#29605=CARTESIAN_POINT('Ctrl Pts',(1.50694078355954,-3.03642785717476,-35.8649524553408));
#29606=CARTESIAN_POINT('Ctrl Pts',(1.52390314248648,-3.02795043409674,-35.8638237741904));
#29607=CARTESIAN_POINT('Ctrl Pts',(1.56852791514194,-3.00517799536937,-35.8608204983834));
#29608=CARTESIAN_POINT('Ctrl Pts',(1.59606542350502,-2.99064367976562,-35.8589324370416));
#29609=CARTESIAN_POINT('Ctrl Pts',(1.75515405330412,-2.90385358523485,-35.8478377590605));
#29610=CARTESIAN_POINT('Ctrl Pts',(1.88198005820198,-2.82330916098814,-35.8382477837061));
#29611=CARTESIAN_POINT('Ctrl Pts',(2.22190461392328,-2.5743244473306,-35.811142967574));
#29612=CARTESIAN_POINT('Ctrl Pts',(2.4207719259826,-2.38828735094287,-35.793666225208));
#29613=CARTESIAN_POINT('Ctrl Pts',(2.62824357639812,-2.14134463149509,-35.7740878728666));
#29614=CARTESIAN_POINT('Ctrl Pts',(2.66025562186351,-2.10144273738525,-35.7710171302957));
#29615=CARTESIAN_POINT('Ctrl Pts',(2.71151645436461,-2.03449833384725,-35.7660131284493));
#29616=CARTESIAN_POINT('Ctrl Pts',(2.73129216285076,-2.00787155713928,-35.7640598230247));
#29617=CARTESIAN_POINT('Ctrl Pts',(2.7694970082527,-1.9548219286716,-35.7602387472698));
#29618=CARTESIAN_POINT('Ctrl Pts',(2.7879465419603,-1.92841816900404,-35.7583703340007));
#29619=CARTESIAN_POINT('Ctrl Pts',(2.83185644359355,-1.86362961156201,-35.753863551595));
#29620=CARTESIAN_POINT('Ctrl Pts',(2.85691658203132,-1.8249805958334,-35.7512399971177));
#29621=CARTESIAN_POINT('Ctrl Pts',(2.95456302344382,-1.66744211377166,-35.7407876002999));
#29622=CARTESIAN_POINT('Ctrl Pts',(3.02058102121791,-1.5446363899599,-35.7331885529657));
#29623=CARTESIAN_POINT('Ctrl Pts',(3.13779660490655,-1.29014891682289,-35.7181530819279));
#29624=CARTESIAN_POINT('Ctrl Pts',(3.18869885792408,-1.15864214182427,-35.7107336777653));
#29625=CARTESIAN_POINT('Ctrl Pts',(3.27357568452938,-0.890901410643851,
-35.6957682698137));
#29626=CARTESIAN_POINT('Ctrl Pts',(3.30756907122169,-0.754972180261875,
-35.6882360499423));
#29627=CARTESIAN_POINT('Ctrl Pts',(3.33987432595466,-0.580555294451817,
-35.6782367155578));
#29628=CARTESIAN_POINT('Ctrl Pts',(3.34607856261757,-0.543657039550838,
-35.6761024735501));
#29629=CARTESIAN_POINT('Ctrl Pts',(3.35473323994378,-0.486404986074056,
-35.6727515128988));
#29630=CARTESIAN_POINT('Ctrl Pts',(3.35761209360037,-0.466117908197508,
-35.6715564866613));
#29631=CARTESIAN_POINT('Ctrl Pts',(3.36266612317762,-0.428022707125048,
-35.6692961122991));
#29632=CARTESIAN_POINT('Ctrl Pts',(3.36488412333369,-0.410221494465349,
-35.6682330218748));
#29633=CARTESIAN_POINT('Ctrl Pts',(3.36993951203867,-0.366844527507218,
-35.6656267425808));
#29634=CARTESIAN_POINT('Ctrl Pts',(3.37262711463376,-0.341252809454412,
-35.6640758649838));
#29635=CARTESIAN_POINT('Ctrl Pts',(3.38166803055292,-0.244579717956199,
-35.6581737932529));
#29636=CARTESIAN_POINT('Ctrl Pts',(3.38606709792027,-0.173338154094305,
-35.6537358352297));
#29637=CARTESIAN_POINT('Ctrl Pts',(3.39209787000417,0.0269591193623061,
-35.6411024242808));
#29638=CARTESIAN_POINT('Ctrl Pts',(3.3886135728306,0.156046133010528,-35.6327827053161));
#29639=CARTESIAN_POINT('Ctrl Pts',(3.35919806089852,0.505146437764565,-35.6102193697391));
#29640=CARTESIAN_POINT('Ctrl Pts',(3.31906075600859,0.723357316537435,-35.5960839801021));
#29641=CARTESIAN_POINT('Ctrl Pts',(3.24228276425979,0.990563709351955,-35.579131222648));
#29642=CARTESIAN_POINT('Ctrl Pts',(3.22527598938504,1.04460966478665,-35.5757181242752));
#29643=CARTESIAN_POINT('Ctrl Pts',(3.19582385311498,1.13061416202461,-35.570309960583));
#29644=CARTESIAN_POINT('Ctrl Pts',(3.18423499574958,1.16285257169047,-35.5682880035938));
#29645=CARTESIAN_POINT('Ctrl Pts',(3.16099830853646,1.2245395834795,-35.5644276608068));
#29646=CARTESIAN_POINT('Ctrl Pts',(3.14942266251315,1.25401135960587,-35.5625871655881));
#29647=CARTESIAN_POINT('Ctrl Pts',(3.12127764948337,1.32281987468349,-35.5582969606599));
#29648=CARTESIAN_POINT('Ctrl Pts',(3.10437471087395,1.36201485701024,-35.5558585177571));
#29649=CARTESIAN_POINT('Ctrl Pts',(3.04234956386105,1.49868254100265,-35.547364184295));
#29650=CARTESIAN_POINT('Ctrl Pts',(2.99333835916829,1.59432386103436,-35.541437015488));
#29651=CARTESIAN_POINT('Ctrl Pts',(2.84655605256545,1.85004207590527,-35.5254372455207));
#29652=CARTESIAN_POINT('Ctrl Pts',(2.73992619745353,2.00458042800868,-35.5156083257711));
#29653=CARTESIAN_POINT('Ctrl Pts',(2.52872369518004,2.26211583136712,-35.4978420196618));
#29654=CARTESIAN_POINT('Ctrl Pts',(2.4292286334931,2.36863913446108,-35.4899830205033));
#29655=CARTESIAN_POINT('Ctrl Pts',(2.30057154086953,2.48972724355342,-35.4799431363505));
#29656=CARTESIAN_POINT('Ctrl Pts',(2.27764635977323,2.510716646156,-35.4781583002393));
#29657=CARTESIAN_POINT('Ctrl Pts',(2.24028431650326,2.54399103644436,-35.4752499083225));
#29658=CARTESIAN_POINT('Ctrl Pts',(2.22602688251641,2.55647579551089,-35.4741401558282));
#29659=CARTESIAN_POINT('Ctrl Pts',(2.19742069022496,2.58110455369589,-35.4719119940472));
#29660=CARTESIAN_POINT('Ctrl Pts',(2.18307413061031,2.59325002772499,-35.470793748612));
#29661=CARTESIAN_POINT('Ctrl Pts',(2.14529786002383,2.62469494669861,-35.467848942649));
#29662=CARTESIAN_POINT('Ctrl Pts',(2.12170906474633,2.64379972334544,-35.4660097871439));
#29663=CARTESIAN_POINT('Ctrl Pts',(1.99654586488111,2.74241663346574,-35.4562634997736));
#29664=CARTESIAN_POINT('Ctrl Pts',(1.89075797493347,2.81639359174969,-35.4480716716442));
#29665=CARTESIAN_POINT('Ctrl Pts',(1.53412583652597,3.03662093769474,-35.4211804309473));
#29666=CARTESIAN_POINT('Ctrl Pts',(1.26862023717671,3.15678103822604,-35.402377130979));
#29667=CARTESIAN_POINT('Ctrl Pts',(0.940328517767844,3.25714570684734,-35.3815053250412));
#29668=CARTESIAN_POINT('Ctrl Pts',(0.88926918375433,3.27145482434731,-35.3783183075523));
#29669=CARTESIAN_POINT('Ctrl Pts',(0.805400792195501,3.29284968847446,-35.3731770256372));
#29670=CARTESIAN_POINT('Ctrl Pts',(0.772786597138734,3.300656071499,-35.3712004682832));
#29671=CARTESIAN_POINT('Ctrl Pts',(0.708851055281177,3.31495973724186,-35.367368413038));
#29672=CARTESIAN_POINT('Ctrl Pts',(0.677543080154877,3.32150016626207,-35.3655117429411));
#29673=CARTESIAN_POINT('Ctrl Pts',(0.602233899826317,3.33612356035288,-35.3610906496112));
#29674=CARTESIAN_POINT('Ctrl Pts',(0.558155540942289,3.34378060511813,-35.3585396273404));
#29675=CARTESIAN_POINT('Ctrl Pts',(0.390112332263439,3.36955645889512,-35.3489390989292));
#29676=CARTESIAN_POINT('Ctrl Pts',(0.265323540830097,3.38167207190852,-35.3420711985415));
#29677=CARTESIAN_POINT('Ctrl Pts',(-0.133825280243136,3.39818802304987,
-35.3205395814368));
#29678=CARTESIAN_POINT('Ctrl Pts',(-0.408123693636666,3.37624031980092,
-35.3064587443863));
#29679=CARTESIAN_POINT('Ctrl Pts',(-0.72917124688984,3.31082706671568,-35.2882542383586));
#29680=CARTESIAN_POINT('Ctrl Pts',(-0.781324390242077,3.29890862792953,
-35.2852380316754));
#29681=CARTESIAN_POINT('Ctrl Pts',(-0.855426656402831,3.28011851518359,
-35.2808400857608));
#29682=CARTESIAN_POINT('Ctrl Pts',(-0.877624030616094,3.27424926300633,
-35.2795081033863));
#29683=CARTESIAN_POINT('Ctrl Pts',(-0.916816127973238,3.26345924341068,
-35.2771277156001));
#29684=CARTESIAN_POINT('Ctrl Pts',(-0.933834647300374,3.25863021426924,
-35.276084315212));
#29685=CARTESIAN_POINT('Ctrl Pts',(-0.971939212435668,3.24749496755305,
-35.273725733932));
#29686=CARTESIAN_POINT('Ctrl Pts',(-0.993002081545012,3.24111650608469,
-35.2724067790341));
#29687=CARTESIAN_POINT('Ctrl Pts',(-1.05834747716395,3.22063124100564,-35.2682705981386));
#29688=CARTESIAN_POINT('Ctrl Pts',(-1.1024013976433,3.20581903481167,-35.2654185209672));
#29689=CARTESIAN_POINT('Ctrl Pts',(-1.20876620773108,3.16760451992292,-35.2583994904839));
#29690=CARTESIAN_POINT('Ctrl Pts',(-1.27071869601075,3.14326379231797,-35.2541985019763));
#29691=CARTESIAN_POINT('Ctrl Pts',(-1.5646566151258,3.01766719613628,-35.2338390689934));
#29692=CARTESIAN_POINT('Ctrl Pts',(-1.78556139979106,2.89244838674332,-35.2173119344543));
#29693=CARTESIAN_POINT('Ctrl Pts',(-2.06815256537044,2.68744509732641,-35.1954943415727));
#29694=CARTESIAN_POINT('Ctrl Pts',(-2.14341477093615,2.62781124612691,-35.1895974241435));
#29695=CARTESIAN_POINT('Ctrl Pts',(-2.244879163353,2.5401523672277,-35.1815282750651));
#29696=CARTESIAN_POINT('Ctrl Pts',(-2.27328707125211,2.51476093791386,-35.1792548913127));
#29697=CARTESIAN_POINT('Ctrl Pts',(-2.32456864559389,2.46734539104511,-35.1751231716981));
#29698=CARTESIAN_POINT('Ctrl Pts',(-2.34757222579197,2.4454687511797,-35.173259075372));
#29699=CARTESIAN_POINT('Ctrl Pts',(-2.39408409152166,2.39997427236873,-35.1694661800941));
#29700=CARTESIAN_POINT('Ctrl Pts',(-2.41755826841108,2.37632642502359,-35.1675389688969));
#29701=CARTESIAN_POINT('Ctrl Pts',(-2.4767171268181,2.31494578202879,-35.1626453363539));
#29702=CARTESIAN_POINT('Ctrl Pts',(-2.51189093953784,2.27673143094917,-35.1597004368941));
#29703=CARTESIAN_POINT('Ctrl Pts',(-2.68311125714268,2.08190979673944,-35.1451537794022));
#29704=CARTESIAN_POINT('Ctrl Pts',(-2.8054612434935,1.91385276459354,-35.1341008080905));
#29705=CARTESIAN_POINT('Ctrl Pts',(-3.01581907170894,1.56096125538752,-35.112297331369));
#29706=CARTESIAN_POINT('Ctrl Pts',(-3.10400753889546,1.37727412792108,-35.1015783717022));
#29707=CARTESIAN_POINT('Ctrl Pts',(-3.18781449811626,1.15305796832824,-35.0880578608937));
#29708=CARTESIAN_POINT('Ctrl Pts',(-3.19989312193933,1.11910131089135,-35.0859984435236));
#29709=CARTESIAN_POINT('Ctrl Pts',(-3.21782618493657,1.06602033691627,-35.0827516677928));
#29710=CARTESIAN_POINT('Ctrl Pts',(-3.22405697578774,1.04702497047019,-35.0815843734478));
#29711=CARTESIAN_POINT('Ctrl Pts',(-3.23561446776625,1.01070887697591,-35.0793404501551));
#29712=CARTESIAN_POINT('Ctrl Pts',(-3.24097087998713,0.993398769585393,
-35.078265455474));
#29713=CARTESIAN_POINT('Ctrl Pts',(-3.25392415086441,0.950318111576882,
-35.07557777389));
#29714=CARTESIAN_POINT('Ctrl Pts',(-3.26135380112186,0.924498879218724,
-35.073956218275));
#29715=CARTESIAN_POINT('Ctrl Pts',(-3.29003392315046,0.820180159838878,
-35.0673688655477));
#29716=CARTESIAN_POINT('Ctrl Pts',(-3.30876191773472,0.741020462581538,
-35.0622897317037));
#29717=CARTESIAN_POINT('Ctrl Pts',(-3.3677558328077,0.444420749121013,-35.0431403213278));
#29718=CARTESIAN_POINT('Ctrl Pts',(-3.3895674096443,0.223877877417544,-35.0287082001579));
#29719=CARTESIAN_POINT('Ctrl Pts',(-3.38974885847844,0.0027818957803985,
-35.0146790786306));
#29720=CARTESIAN_POINT('',(-3.38974998254981,0.000343952908442827,-32.5190351755825));
#29721=CARTESIAN_POINT('Ctrl Pts',(-3.38974886104885,0.00277876196049448,
-35.0146788797815));
#29722=CARTESIAN_POINT('Ctrl Pts',(-3.38982690422481,-0.0924243430868422,
-35.0086379939658));
#29723=CARTESIAN_POINT('Ctrl Pts',(-3.38589419625354,-0.187595440304559,
-35.0026733461612));
#29724=CARTESIAN_POINT('Ctrl Pts',(-3.37293905739721,-0.342514592893689,
-34.9931112098591));
#29725=CARTESIAN_POINT('Ctrl Pts',(-3.36631922380223,-0.402404885928521,
-34.9894503069998));
#29726=CARTESIAN_POINT('Ctrl Pts',(-3.35379977026001,-0.493386448102765,
-34.9839425626804));
#29727=CARTESIAN_POINT('Ctrl Pts',(-3.34905581760021,-0.524622071065607,
-34.982061307855));
#29728=CARTESIAN_POINT('Ctrl Pts',(-3.33864491805334,-0.587258865172567,
-34.9783072956048));
#29729=CARTESIAN_POINT('Ctrl Pts',(-3.33296990619702,-0.618655454138839,
-34.9764349946944));
#29730=CARTESIAN_POINT('Ctrl Pts',(-3.32039385159822,-0.683025811840888,
-34.9726140902599));
#29731=CARTESIAN_POINT('Ctrl Pts',(-3.3134428264174,-0.715986272984172,
-34.9706672713481));
#29732=CARTESIAN_POINT('Ctrl Pts',(-3.2941222857227,-0.801283347624241,
-34.9656510515532));
#29733=CARTESIAN_POINT('Ctrl Pts',(-3.28099640480404,-0.853439904297473,
-34.9626054396638));
#29734=CARTESIAN_POINT('Ctrl Pts',(-3.19872454510333,-1.15031689560506,
-34.9453548010599));
#29735=CARTESIAN_POINT('Ctrl Pts',(-3.10345829663412,-1.3869478189448,-34.9320159235403));
#29736=CARTESIAN_POINT('Ctrl Pts',(-2.91209376832095,-1.74130504901877,
-34.9105885352962));
#29737=CARTESIAN_POINT('Ctrl Pts',(-2.83307429722507,-1.8671142113853,-34.9026298518415));
#29738=CARTESIAN_POINT('Ctrl Pts',(-2.72340772966983,-2.01865060633102,
-34.8920944175098));
#29739=CARTESIAN_POINT('Ctrl Pts',(-2.70020698384903,-2.04958091179739,
-34.8898902172084));
#29740=CARTESIAN_POINT('Ctrl Pts',(-2.66388893673579,-2.09631152873596,
-34.8864653816285));
#29741=CARTESIAN_POINT('Ctrl Pts',(-2.651147961684,-2.11240165016111,-34.8852684963686));
#29742=CARTESIAN_POINT('Ctrl Pts',(-2.62700414677674,-2.14232951565063,
-34.8830068796901));
#29743=CARTESIAN_POINT('Ctrl Pts',(-2.61563641773531,-2.15619401155531,
-34.8819444464711));
#29744=CARTESIAN_POINT('Ctrl Pts',(-2.58773013465438,-2.18968410729951,
-34.8793429744375));
#29745=CARTESIAN_POINT('Ctrl Pts',(-2.57107787604637,-2.2092130290383,-34.8777963171741));
#29746=CARTESIAN_POINT('Ctrl Pts',(-2.51093542071305,-2.27814403811377,
-34.8722361233496));
#29747=CARTESIAN_POINT('Ctrl Pts',(-2.46623226764138,-2.32646388856345,
-34.8681505158557));
#29748=CARTESIAN_POINT('Ctrl Pts',(-2.24375158879616,-2.55332261558018,
-34.8481621869646));
#29749=CARTESIAN_POINT('Ctrl Pts',(-2.04784572541907,-2.71297165087198,
-34.8316493323975));
#29750=CARTESIAN_POINT('Ctrl Pts',(-1.72815727676698,-2.91896408340487,
-34.8075972434133));
#29751=CARTESIAN_POINT('Ctrl Pts',(-1.61639515349901,-2.98230643125532,
-34.7996342873614));
#29752=CARTESIAN_POINT('Ctrl Pts',(-1.46091289751696,-3.05911221545851,
-34.78916749588));
#29753=CARTESIAN_POINT('Ctrl Pts',(-1.4201324522529,-3.07825569928002,-34.7864756530796));
#29754=CARTESIAN_POINT('Ctrl Pts',(-1.34971782903468,-3.10961299889367,
-34.7819161898915));
#29755=CARTESIAN_POINT('Ctrl Pts',(-1.32027064987619,-3.12222944965444,
-34.7800353246241));
#29756=CARTESIAN_POINT('Ctrl Pts',(-1.2634153235531,-3.14564050097317,-34.7764517186054));
#29757=CARTESIAN_POINT('Ctrl Pts',(-1.23603678667977,-3.15649894378423,
-34.7747470011713));
#29758=CARTESIAN_POINT('Ctrl Pts',(-1.16290015217932,-3.18440771224144,
-34.7702464072632));
#29759=CARTESIAN_POINT('Ctrl Pts',(-1.1169084277803,-3.20082882119852,-34.767471080449));
#29760=CARTESIAN_POINT('Ctrl Pts',(-0.900493809802508,-3.27286559500886,
-34.7546428422546));
#29761=CARTESIAN_POINT('Ctrl Pts',(-0.72618148303251,-3.31590226899461,
-34.7449914641347));
#29762=CARTESIAN_POINT('Ctrl Pts',(-0.379578793328886,-3.37281719444198,
-34.726300713963));
#29763=CARTESIAN_POINT('Ctrl Pts',(-0.208023834352916,-3.38772733832745,
-34.7172749306414));
#29764=CARTESIAN_POINT('Ctrl Pts',(0.047085910097641,-3.39044342520962,
-34.7033694546863));
#29765=CARTESIAN_POINT('Ctrl Pts',(0.130257999734886,-3.38826718370647,
-34.6987573660932));
#29766=CARTESIAN_POINT('Ctrl Pts',(0.240265078516032,-3.38133257232834,
-34.6924579124442));
#29767=CARTESIAN_POINT('Ctrl Pts',(0.267248596295292,-3.37930693511218,
-34.6908967460967));
#29768=CARTESIAN_POINT('Ctrl Pts',(0.312288774480554,-3.375382989154,-34.6882599348768));
#29769=CARTESIAN_POINT('Ctrl Pts',(0.330360255566219,-3.37366220801277,
-34.6871935860849));
#29770=CARTESIAN_POINT('Ctrl Pts',(0.368228177019154,-3.36974921072111,
-34.6849401296154));
#29771=CARTESIAN_POINT('Ctrl Pts',(0.388020327948082,-3.36752756711329,
-34.683751625354));
#29772=CARTESIAN_POINT('Ctrl Pts',(0.443209978488878,-3.3608396107482,-34.6804097647904));
#29773=CARTESIAN_POINT('Ctrl Pts',(0.47855730307099,-3.35598877603464,-34.6782374617739));
#29774=CARTESIAN_POINT('Ctrl Pts',(0.758580321919093,-3.31304655222868,
-34.6608083933622));
#29775=CARTESIAN_POINT('Ctrl Pts',(0.998479534114965,-3.24880794519959,
-34.6446007813284));
#29776=CARTESIAN_POINT('Ctrl Pts',(1.33625315593318,-3.11737391340009,-34.6214151778978));
#29777=CARTESIAN_POINT('Ctrl Pts',(1.44109473445916,-3.0703162874983,-34.614151712773));
#29778=CARTESIAN_POINT('Ctrl Pts',(1.61507637750078,-2.9813458370174,-34.6020485668035));
#29779=CARTESIAN_POINT('Ctrl Pts',(1.68547421987451,-2.9421204875355,-34.5971356323225));
#29780=CARTESIAN_POINT('Ctrl Pts',(1.78754027826934,-2.88038258668276,-34.5899885204448));
#29781=CARTESIAN_POINT('Ctrl Pts',(1.82032374714407,-2.85977721737487,-34.5876888672072));
#29782=CARTESIAN_POINT('Ctrl Pts',(1.87891134715219,-2.82153740751192,-34.5835700369392));
#29783=CARTESIAN_POINT('Ctrl Pts',(1.90483791915879,-2.80409946156646,-34.5817440172448));
#29784=CARTESIAN_POINT('Ctrl Pts',(1.96052894272978,-2.7655133591886,-34.5778126423914));
#29785=CARTESIAN_POINT('Ctrl Pts',(1.99020046699295,-2.74423762164994,-34.5757123216832));
#29786=CARTESIAN_POINT('Ctrl Pts',(2.07269969422843,-2.68304020503453,-34.5698513756995));
#29787=CARTESIAN_POINT('Ctrl Pts',(2.12471106887763,-2.64204322917209,-34.566131601432));
#29788=CARTESIAN_POINT('Ctrl Pts',(2.36883912125081,-2.43773906428165,-34.5484816449661));
#29789=CARTESIAN_POINT('Ctrl Pts',(2.54352796260521,-2.25487041198006,-34.5353339358947));
#29790=CARTESIAN_POINT('Ctrl Pts',(2.78161233832029,-1.94238020353759,-34.5143564651655));
#29791=CARTESIAN_POINT('Ctrl Pts',(2.85983464248742,-1.82525233641982,-34.5067468903608));
#29792=CARTESIAN_POINT('Ctrl Pts',(2.94604314139119,-1.67695729859936,-34.496996244675));
#29793=CARTESIAN_POINT('Ctrl Pts',(2.96117599889122,-1.65008864443326,-34.4952250266343));
#29794=CARTESIAN_POINT('Ctrl Pts',(2.98498861800167,-1.60642621811201,-34.4923334026055));
#29795=CARTESIAN_POINT('Ctrl Pts',(2.9938984525569,-1.58975918375157,-34.4912265136524));
#29796=CARTESIAN_POINT('Ctrl Pts',(3.01141434457904,-1.55632385093623,-34.4889981508541));
#29797=CARTESIAN_POINT('Ctrl Pts',(3.02002084306773,-1.53955654410371,-34.4878767579429));
#29798=CARTESIAN_POINT('Ctrl Pts',(3.04222895874108,-1.49538753152628,-34.4849142697675));
#29799=CARTESIAN_POINT('Ctrl Pts',(3.05559995408492,-1.46787250316995,-34.4830603185984));
#29800=CARTESIAN_POINT('Ctrl Pts',(3.12203706839389,-1.32631486062107,-34.4734931609101));
#29801=CARTESIAN_POINT('Ctrl Pts',(3.16909422511869,-1.2095713718572,-34.4655108527891));
#29802=CARTESIAN_POINT('Ctrl Pts',(3.27478666286398,-0.898496657571354,
-34.4444418374273));
#29803=CARTESIAN_POINT('Ctrl Pts',(3.32266627058404,-0.701015921487936,
-34.4312867947251));
#29804=CARTESIAN_POINT('Ctrl Pts',(3.36907463558273,-0.390108002041411,
-34.4115286979423));
#29805=CARTESIAN_POINT('Ctrl Pts',(3.38008809278936,-0.279028156420628,
-34.4046454587518));
#29806=CARTESIAN_POINT('Ctrl Pts',(3.387739896363,-0.124455798019335,-34.395322880176));
#29807=CARTESIAN_POINT('Ctrl Pts',(3.38905080939095,-0.0812755772965244,
-34.3927456916865));
#29808=CARTESIAN_POINT('Ctrl Pts',(3.38989263039676,-0.00634539808840575,
-34.3883185136122));
#29809=CARTESIAN_POINT('Ctrl Pts',(3.38980346890386,0.0253939600347397,
-34.3864571985843));
#29810=CARTESIAN_POINT('Ctrl Pts',(3.38869465853402,0.0911768085449157,
-34.3826267956063));
#29811=CARTESIAN_POINT('Ctrl Pts',(3.38760768910887,0.12521567487828,-34.3806599755761));
#29812=CARTESIAN_POINT('Ctrl Pts',(3.38339448490624,0.214807128708987,-34.3755198093596));
#29813=CARTESIAN_POINT('Ctrl Pts',(3.37941314899832,0.270310188160491,-34.3723726237765));
#29814=CARTESIAN_POINT('Ctrl Pts',(3.35138791555575,0.560642492992985,-34.356064483073));
#29815=CARTESIAN_POINT('Ctrl Pts',(3.30423138807837,0.792581950040394,-34.3436247233995));
#29816=CARTESIAN_POINT('Ctrl Pts',(3.18203957869957,1.18077919016614,-34.3220050374073));
#29817=CARTESIAN_POINT('Ctrl Pts',(3.11847370633536,1.33967349091239,-34.3128847286386));
#29818=CARTESIAN_POINT('Ctrl Pts',(3.028184406851,1.52370197866563,-34.3012802745253));
#29819=CARTESIAN_POINT('Ctrl Pts',(3.01269946871612,1.55409467099378,-34.2993276287108));
#29820=CARTESIAN_POINT('Ctrl Pts',(2.98760338732323,1.60156637139249,-34.2962124072376));
#29821=CARTESIAN_POINT('Ctrl Pts',(2.97829786937535,1.61880530089336,-34.2950673489921));
#29822=CARTESIAN_POINT('Ctrl Pts',(2.96010590324536,1.65181896467861,-34.2928459738907));
#29823=CARTESIAN_POINT('Ctrl Pts',(2.95124160465024,1.66760480554725,-34.2917709541762));
#29824=CARTESIAN_POINT('Ctrl Pts',(2.92845116777581,1.70743993326548,-34.2890268015878));
#29825=CARTESIAN_POINT('Ctrl Pts',(2.91435508712683,1.73139010196063,-34.2873476786546));
#29826=CARTESIAN_POINT('Ctrl Pts',(2.85671301609949,1.82662914591736,-34.2805608077938));
#29827=CARTESIAN_POINT('Ctrl Pts',(2.81083545310889,1.89646652462634,-34.2753352262041));
#29828=CARTESIAN_POINT('Ctrl Pts',(2.6380484380674,2.13943112941956,-34.25643062724));
#29829=CARTESIAN_POINT('Ctrl Pts',(2.49733850557292,2.3021230731035,-34.2424324035838));
#29830=CARTESIAN_POINT('Ctrl Pts',(2.2405586149924,2.54756079739279,-34.2198805859861));
#29831=CARTESIAN_POINT('Ctrl Pts',(2.13297840919079,2.63829108123176,-34.2111266444174));
#29832=CARTESIAN_POINT('Ctrl Pts',(1.9829884592345,2.74959874265178,-34.1998407347253));
#29833=CARTESIAN_POINT('Ctrl Pts',(1.94535511608205,2.77635196988582,-34.1970792399544));
#29834=CARTESIAN_POINT('Ctrl Pts',(1.88054234961348,2.82046169728733,-34.1924386905388));
#29835=CARTESIAN_POINT('Ctrl Pts',(1.85364125362016,2.8382138615208,-34.1905451964203));
#29836=CARTESIAN_POINT('Ctrl Pts',(1.79857558217943,2.87343504720916,-34.1867331930546));
#29837=CARTESIAN_POINT('Ctrl Pts',(1.77039980389121,2.89088009818977,-34.1848156913425));
#29838=CARTESIAN_POINT('Ctrl Pts',(1.69821794267487,2.93412036244863,-34.1799834300892));
#29839=CARTESIAN_POINT('Ctrl Pts',(1.65387640054368,2.95934109472077,-34.1770890852916));
#29840=CARTESIAN_POINT('Ctrl Pts',(1.36931157522843,3.11280223228045,-34.1589416404228));
#29841=CARTESIAN_POINT('Ctrl Pts',(1.1149486422462,3.21270146399418,-34.1447188437405));
#29842=CARTESIAN_POINT('Ctrl Pts',(0.706691321019504,3.31863389521196,-34.1222359671799));
#29843=CARTESIAN_POINT('Ctrl Pts',(0.559711031811383,3.34655914131875,-34.1141814014913));
#29844=CARTESIAN_POINT('Ctrl Pts',(0.380495662063168,3.36847094907184,-34.103921970846));
#29845=CARTESIAN_POINT('Ctrl Pts',(0.349556827479023,3.37182196490236,-34.1021350630129));
#29846=CARTESIAN_POINT('Ctrl Pts',(0.29970217596337,3.37652826406392,-34.099224119708));
#29847=CARTESIAN_POINT('Ctrl Pts',(0.280812807596176,3.37815166056643,-34.0981139312925));
#29848=CARTESIAN_POINT('Ctrl Pts',(0.245425847365641,3.38089405612176,-34.0960189027458));
#29849=CARTESIAN_POINT('Ctrl Pts',(0.228931684723151,3.38205096360446,-34.0950361934042));
#29850=CARTESIAN_POINT('Ctrl Pts',(0.184365920817121,3.38484932843634,-34.0923654626453));
#29851=CARTESIAN_POINT('Ctrl Pts',(0.156281830147808,3.38626219395434,-34.0906658153288));
#29852=CARTESIAN_POINT('Ctrl Pts',(0.0410736120218453,3.39062194637338,
-34.0836340332441));
#29853=CARTESIAN_POINT('Ctrl Pts',(-0.0461256647190106,3.39055664230569,
-34.0781733023392));
#29854=CARTESIAN_POINT('Ctrl Pts',(-0.344170923460956,3.37883430929543,
-34.0592348346581));
#29855=CARTESIAN_POINT('Ctrl Pts',(-0.5538886370471,3.35084877875865,-34.0454722381292));
#29856=CARTESIAN_POINT('Ctrl Pts',(-0.895972408694878,3.27218670582534,
-34.0231917227614));
#29857=CARTESIAN_POINT('Ctrl Pts',(-1.03023846418474,3.23242769352349,-34.0144831957068));
#29858=CARTESIAN_POINT('Ctrl Pts',(-1.2049923575738,3.16867865182188,-34.0032439002521));
#29859=CARTESIAN_POINT('Ctrl Pts',(-1.247982515665,3.15199475459977,-34.0004860993103));
#29860=CARTESIAN_POINT('Ctrl Pts',(-1.32041155998456,3.12217173589579,-33.9958498607988));
#29861=CARTESIAN_POINT('Ctrl Pts',(-1.35002690204469,3.10948074541583,-33.9939570476905));
#29862=CARTESIAN_POINT('Ctrl Pts',(-1.40617296441659,3.08446721872072,-33.9903726190409));
#29863=CARTESIAN_POINT('Ctrl Pts',(-1.4327337628727,3.07221979542705,-33.9886787036729));
#29864=CARTESIAN_POINT('Ctrl Pts',(-1.50211284904934,3.03913300309358,-33.9842566093757));
#29865=CARTESIAN_POINT('Ctrl Pts',(-1.54465707347693,3.01773213870837,-33.9815475853754));
#29866=CARTESIAN_POINT('Ctrl Pts',(-1.71123422964111,2.92949329442905,-33.9709334303889));
#29867=CARTESIAN_POINT('Ctrl Pts',(-1.83150452424359,2.85584491763664,-33.9632608626042));
#29868=CARTESIAN_POINT('Ctrl Pts',(-2.11437066166908,2.65738925318995,-33.9447401392526));
#29869=CARTESIAN_POINT('Ctrl Pts',(-2.27089458589667,2.52493804283488,-33.9340762232955));
#29870=CARTESIAN_POINT('Ctrl Pts',(-2.47774434496852,2.31501709533584,-33.918068483271));
#29871=CARTESIAN_POINT('Ctrl Pts',(-2.53838805005272,2.24835601688879,-33.913089983142));
#29872=CARTESIAN_POINT('Ctrl Pts',(-2.61412830695887,2.15812585139271,-33.9063641739515));
#29873=CARTESIAN_POINT('Ctrl Pts',(-2.63169457216682,2.13666973791777,-33.9047656902064));
#29874=CARTESIAN_POINT('Ctrl Pts',(-2.66039688509124,2.10072068920883,-33.9020843802752));
#29875=CARTESIAN_POINT('Ctrl Pts',(-2.67168291330316,2.08634834074651,-33.9010115727456));
#29876=CARTESIAN_POINT('Ctrl Pts',(-2.69487819497183,2.05631313302973,-33.8987664425462));
#29877=CARTESIAN_POINT('Ctrl Pts',(-2.70676812006585,2.0406367851908,-33.8975930315553));
#29878=CARTESIAN_POINT('Ctrl Pts',(-2.73913920649202,1.99717622962009,-33.8943375632345));
#29879=CARTESIAN_POINT('Ctrl Pts',(-2.75933297341615,1.96918202013568,-33.8922380276508));
#29880=CARTESIAN_POINT('Ctrl Pts',(-2.90427141219207,1.76164908418293,-33.8766830481539));
#29881=CARTESIAN_POINT('Ctrl Pts',(-3.01180706092764,1.5707347405806,-33.862462698946));
#29882=CARTESIAN_POINT('Ctrl Pts',(-3.17838338482558,1.19400785940032,-33.8359956404397));
#29883=CARTESIAN_POINT('Ctrl Pts',(-3.24130113660487,1.01082189572249,-33.8237566009576));
#29884=CARTESIAN_POINT('Ctrl Pts',(-3.30105900602259,0.772134059237047,
-33.8088007363692));
#29885=CARTESIAN_POINT('Ctrl Pts',(-3.3126630524489,0.720725697539464,-33.8056339120265));
#29886=CARTESIAN_POINT('Ctrl Pts',(-3.32967030175316,0.636255361438118,
-33.8005164773026));
#29887=CARTESIAN_POINT('Ctrl Pts',(-3.33579016482181,0.603348405979583,
-33.7985439698615));
#29888=CARTESIAN_POINT('Ctrl Pts',(-3.34674838592617,0.539149758655512,
-33.7947351132573));
#29889=CARTESIAN_POINT('Ctrl Pts',(-3.35163765731479,0.507870390737447,
-33.7928973667653));
#29890=CARTESIAN_POINT('Ctrl Pts',(-3.36236980150594,0.432285853419744,
-33.7884976425721));
#29891=CARTESIAN_POINT('Ctrl Pts',(-3.36777624898775,0.387924142197492,
-33.7859492800458));
#29892=CARTESIAN_POINT('Ctrl Pts',(-3.38400763646391,0.228557513167015,
-33.776902692303));
#29893=CARTESIAN_POINT('Ctrl Pts',(-3.38983092727204,0.113119094727432,
-33.7705541994048));
#29894=CARTESIAN_POINT('Ctrl Pts',(-3.38958757092891,-0.230649292059321,
-33.7519739261274));
#29895=CARTESIAN_POINT('Ctrl Pts',(-3.36637334460148,-0.458287124936508,
-33.7401275512925));
#29896=CARTESIAN_POINT('Ctrl Pts',(-3.30112254656824,-0.776040945303472,
-33.7225654538627));
#29897=CARTESIAN_POINT('Ctrl Pts',(-3.27778502338376,-0.869351485472063,
-33.7172710373615));
#29898=CARTESIAN_POINT('Ctrl Pts',(-3.24231509939374,-0.989259157956663,
-33.7101442169138));
#29899=CARTESIAN_POINT('Ctrl Pts',(-3.23376027829352,-1.01687522807927,
-33.7084800290812));
#29900=CARTESIAN_POINT('Ctrl Pts',(-3.21971606485589,-1.06024128279909,
-33.7058257648327));
#29901=CARTESIAN_POINT('Ctrl Pts',(-3.21446167112142,-1.0760665663484,-33.7048484835209));
#29902=CARTESIAN_POINT('Ctrl Pts',(-3.20304920165912,-1.10960925254065,
-33.702757327867));
#29903=CARTESIAN_POINT('Ctrl Pts',(-3.19686044851894,-1.12731544459897,
-33.7016416492259));
#29904=CARTESIAN_POINT('Ctrl Pts',(-3.18033780316556,-1.17335680068938,
-33.6987113216133));
#29905=CARTESIAN_POINT('Ctrl Pts',(-3.1697722962889,-1.20160649849822,-33.6968842906415));
#29906=CARTESIAN_POINT('Ctrl Pts',(-3.11349267381627,-1.34617538055025,
-33.6873976541616));
#29907=CARTESIAN_POINT('Ctrl Pts',(-3.06175103806851,-1.46003422783873,
-33.6794705559301));
#29908=CARTESIAN_POINT('Ctrl Pts',(-2.87251916865601,-1.82191101057061,
-33.6532892840511));
#29909=CARTESIAN_POINT('Ctrl Pts',(-2.71018547359303,-2.05564329151342,
-33.6348981444548));
#29910=CARTESIAN_POINT('Ctrl Pts',(-2.48126986182878,-2.31023186044375,
-33.6139858574241));
#29911=CARTESIAN_POINT('Ctrl Pts',(-2.44076904396329,-2.35298076765167,
-33.6104337927574));
#29912=CARTESIAN_POINT('Ctrl Pts',(-2.37466077365739,-2.41921376989797,
-33.6048618921935));
#29913=CARTESIAN_POINT('Ctrl Pts',(-2.34977201870952,-2.44339531139193,
-33.6028121834748));
#29914=CARTESIAN_POINT('Ctrl Pts',(-2.30157152496064,-2.48880841323714,
-33.5989313170498));
#29915=CARTESIAN_POINT('Ctrl Pts',(-2.27832642819208,-2.51010509478455,
-33.5970975199136));
#29916=CARTESIAN_POINT('Ctrl Pts',(-2.22367282168149,-2.55879280491719,
-33.5928703978457));
#29917=CARTESIAN_POINT('Ctrl Pts',(-2.19204924390185,-2.58593537502077,
-33.5904873124589));
#29918=CARTESIAN_POINT('Ctrl Pts',(-2.08301725361847,-2.67607995535169,
-33.5824711351141));
#29919=CARTESIAN_POINT('Ctrl Pts',(-2.00332771654797,-2.73624656227071,
-33.5769470788099));
#29920=CARTESIAN_POINT('Ctrl Pts',(-1.78674439549559,-2.88522787384046,
-33.562634828032));
#29921=CARTESIAN_POINT('Ctrl Pts',(-1.6458973334152,-2.96783087167764,-33.554023574467));
#29922=CARTESIAN_POINT('Ctrl Pts',(-1.34952063081701,-3.11403645803161,
-33.5364725832783));
#29923=CARTESIAN_POINT('Ctrl Pts',(-1.19412464909152,-3.17686709673405,
-33.5275510093057));
#29924=CARTESIAN_POINT('Ctrl Pts',(-0.998751741711168,-3.23949508585984,
-33.515990352926));
#29925=CARTESIAN_POINT('Ctrl Pts',(-0.962572696906014,-3.25042874250805,
-33.513835225288));
#29926=CARTESIAN_POINT('Ctrl Pts',(-0.906432122661093,-3.2663755177457,
-33.5104583875593));
#29927=CARTESIAN_POINT('Ctrl Pts',(-0.886594028074614,-3.27181588702464,
-33.5092588996264));
#29928=CARTESIAN_POINT('Ctrl Pts',(-0.849387287517357,-3.28165618210674,
-33.5069955184983));
#29929=CARTESIAN_POINT('Ctrl Pts',(-0.832031386866415,-3.28609947777207,
-33.5059339799804));
#29930=CARTESIAN_POINT('Ctrl Pts',(-0.789819624934591,-3.29655030526925,
-33.5033391217881));
#29931=CARTESIAN_POINT('Ctrl Pts',(-0.76492979701057,-3.3024144613338,-33.5017982804914));
#29932=CARTESIAN_POINT('Ctrl Pts',(-0.67160076930187,-3.32329154645115,
-33.4959863355616));
#29933=CARTESIAN_POINT('Ctrl Pts',(-0.602771362054284,-3.33646214517497,
-33.4916316908523));
#29934=CARTESIAN_POINT('Ctrl Pts',(-0.410140706734968,-3.36716738381519,
-33.4793417682405));
#29935=CARTESIAN_POINT('Ctrl Pts',(-0.285703800938918,-3.38000037518403,
-33.4712889483607));
#29936=CARTESIAN_POINT('Ctrl Pts',(0.0665665797099702,-3.396734914986,-33.4485737223653));
#29937=CARTESIAN_POINT('Ctrl Pts',(0.294522395735952,-3.38460092837313,
-33.4340140258785));
#29938=CARTESIAN_POINT('Ctrl Pts',(0.575199971240628,-3.34106569254644,
-33.4166991185306));
#29939=CARTESIAN_POINT('Ctrl Pts',(0.630615251683416,-3.33105087573173,
-33.4133075510693));
#29940=CARTESIAN_POINT('Ctrl Pts',(0.719237411589568,-3.31274377463789,
-33.4079247835941));
#29941=CARTESIAN_POINT('Ctrl Pts',(0.752611236702497,-3.30532150090951,
-33.4059071432027));
#29942=CARTESIAN_POINT('Ctrl Pts',(0.816690848854646,-3.29004941168908,
-33.4020497998382));
#29943=CARTESIAN_POINT('Ctrl Pts',(0.847409901580814,-3.28227141351291,
-33.4002080723699));
#29944=CARTESIAN_POINT('Ctrl Pts',(0.91940460470855,-3.26296436272826,-33.3959070518673));
#29945=CARTESIAN_POINT('Ctrl Pts',(0.960580090632091,-3.25108095591568,
-33.3934592015028));
#29946=CARTESIAN_POINT('Ctrl Pts',(1.10542587100572,-3.20628564171881,-33.3848799033921));
#29947=CARTESIAN_POINT('Ctrl Pts',(1.20772978215323,-3.16916798519504,-33.3788808702972));
#29948=CARTESIAN_POINT('Ctrl Pts',(1.47335019931879,-3.05806115134583,-33.3632659170203));
#29949=CARTESIAN_POINT('Ctrl Pts',(1.63288022594376,-2.97593723923242,-33.3538572650203));
#29950=CARTESIAN_POINT('Ctrl Pts',(1.90415739098513,-2.8078781740471,-33.3368540579961));
#29951=CARTESIAN_POINT('Ctrl Pts',(2.01845030156449,-2.72687488923117,-33.3293232744458));
#29952=CARTESIAN_POINT('Ctrl Pts',(2.15652736667546,-2.61556774086048,-33.3193255694748));
#29953=CARTESIAN_POINT('Ctrl Pts',(2.18526380609547,-2.59160698193444,-33.3171913811095));
#29954=CARTESIAN_POINT('Ctrl Pts',(2.22911452090418,-2.55379587401048,-33.3138404866312));
#29955=CARTESIAN_POINT('Ctrl Pts',(2.24451044594963,-2.54027512785831,-33.3126454715545));
#29956=CARTESIAN_POINT('Ctrl Pts',(2.27315414420973,-2.51465646419266,-33.3103851040725));
#29957=CARTESIAN_POINT('Ctrl Pts',(2.28642991286373,-2.50259167544523,-33.3093220091149));
#29958=CARTESIAN_POINT('Ctrl Pts',(2.31851470370448,-2.47296518647542,-33.306715698344));
#29959=CARTESIAN_POINT('Ctrl Pts',(2.33722044479533,-2.45529382139935,-33.3051647933528));
#29960=CARTESIAN_POINT('Ctrl Pts',(2.4070397709563,-2.38781447267138,-33.2992624748821));
#29961=CARTESIAN_POINT('Ctrl Pts',(2.45677446713755,-2.33661212705251,-33.2948242886297));
#29962=CARTESIAN_POINT('Ctrl Pts',(2.59179809789646,-2.18852467634677,-33.2821899273249));
#29963=CARTESIAN_POINT('Ctrl Pts',(2.67322413028724,-2.08828349997284,-33.2738694674998));
#29964=CARTESIAN_POINT('Ctrl Pts',(2.8782347061422,-1.80420118401244,-33.2513065257479));
#29965=CARTESIAN_POINT('Ctrl Pts',(2.98986834418226,-1.61247939164622,-33.237172282167));
#29966=CARTESIAN_POINT('Ctrl Pts',(3.10560602388813,-1.35971515142524,-33.2202205180091));
#29967=CARTESIAN_POINT('Ctrl Pts',(3.12789592060347,-1.30762446913768,-33.2168073740174));
#29968=CARTESIAN_POINT('Ctrl Pts',(3.16155325642045,-1.22317598918447,-33.2113991563452));
#29969=CARTESIAN_POINT('Ctrl Pts',(3.17375297204456,-1.19116358837664,-33.2093771900424));
#29970=CARTESIAN_POINT('Ctrl Pts',(3.1962907946282,-1.12921771651209,-33.2055168403932));
#29971=CARTESIAN_POINT('Ctrl Pts',(3.2066987779171,-1.09931366857137,-33.2036763474485));
#29972=CARTESIAN_POINT('Ctrl Pts',(3.23014923994992,-1.02876743916606,-33.1993861642674));
#29973=CARTESIAN_POINT('Ctrl Pts',(3.24284627148427,-0.988015610180735,
-33.1969477404765));
#29974=CARTESIAN_POINT('Ctrl Pts',(3.28477606706078,-0.843911027164396,
-33.1884535800894));
#29975=CARTESIAN_POINT('Ctrl Pts',(3.30986512477057,-0.739415557750358,
-33.1825265577575));
#29976=CARTESIAN_POINT('Ctrl Pts',(3.36500111904763,-0.449778692293402,
-33.1665274462738));
#29977=CARTESIAN_POINT('Ctrl Pts',(3.38471977495014,-0.263071598775227,
-33.1566990097192));
#29978=CARTESIAN_POINT('Ctrl Pts',(3.39215679905814,0.0699119802708021,
-33.1389325557749));
#29979=CARTESIAN_POINT('Ctrl Pts',(3.38602152600385,0.215557880546048,-33.131072877132));
#29980=CARTESIAN_POINT('Ctrl Pts',(3.36723869527788,0.391247663705663,-33.121032235086));
#29981=CARTESIAN_POINT('Ctrl Pts',(3.3635097464359,0.422105681653361,-33.1192473959467));
#29982=CARTESIAN_POINT('Ctrl Pts',(3.35682505184185,0.471688227620651,-33.1163390002505));
#29983=CARTESIAN_POINT('Ctrl Pts',(3.35413556856925,0.490447512835545,-33.1152292470669));
#29984=CARTESIAN_POINT('Ctrl Pts',(3.34846539057391,0.527766932086595,-33.1130010853458));
#29985=CARTESIAN_POINT('Ctrl Pts',(3.34548732531331,0.546326753637205,-33.1118828406793));
#29986=CARTESIAN_POINT('Ctrl Pts',(3.33729690947443,0.594790556610575,-33.1089380387386));
#29987=CARTESIAN_POINT('Ctrl Pts',(3.33183706087192,0.624650405556525,-33.1070988865434));
#29988=CARTESIAN_POINT('Ctrl Pts',(3.30107365063774,0.78099734309863,-33.0973526706085));
#29989=CARTESIAN_POINT('Ctrl Pts',(3.26896802608414,0.906027782546418,-33.0891609153821));
#29990=CARTESIAN_POINT('Ctrl Pts',(3.1417404640823,1.30540294946159,-33.0622696173468));
#29991=CARTESIAN_POINT('Ctrl Pts',(3.0185010387914,1.56949562350026,-33.043466177757));
#29992=CARTESIAN_POINT('Ctrl Pts',(2.83472248995926,1.85945267099938,-33.0225942797385));
#29993=CARTESIAN_POINT('Ctrl Pts',(2.80529273004858,1.90356218744007,-33.0194072893487));
#29994=CARTESIAN_POINT('Ctrl Pts',(2.75557897934114,1.97441484738668,-33.0142660396197));
#29995=CARTESIAN_POINT('Ctrl Pts',(2.73591214558279,2.00157796568216,-33.0122894878802));
#29996=CARTESIAN_POINT('Ctrl Pts',(2.69670702001363,2.05406892021864,-33.0084574360071));
#29997=CARTESIAN_POINT('Ctrl Pts',(2.6772069704642,2.07942078953108,-33.0066007637849));
#29998=CARTESIAN_POINT('Ctrl Pts',(2.62957850237576,2.1395614046487,-33.0021796531248));
#29999=CARTESIAN_POINT('Ctrl Pts',(2.60111415750851,2.1740771621632,-32.9996286159414));
#30000=CARTESIAN_POINT('Ctrl Pts',(2.49037179336167,2.30307345995335,-32.9900279240602));
#30001=CARTESIAN_POINT('Ctrl Pts',(2.40355888159715,2.39353461554367,-32.9831598837663));
#30002=CARTESIAN_POINT('Ctrl Pts',(2.11138770723128,2.66601645534111,-32.9616270865751));
#30003=CARTESIAN_POINT('Ctrl Pts',(1.8889150198122,2.82799830735902,-32.9475453066251));
#30004=CARTESIAN_POINT('Ctrl Pts',(1.60267083293559,2.98742549060242,-32.9293403696739));
#30005=CARTESIAN_POINT('Ctrl Pts',(1.55534470717127,3.01233581598341,-32.9263250338815));
#30006=CARTESIAN_POINT('Ctrl Pts',(1.48688924114406,3.04632442547569,-32.9219281338846));
#30007=CARTESIAN_POINT('Ctrl Pts',(1.46622397861806,3.05632447598448,-32.9205962941572));
#30008=CARTESIAN_POINT('Ctrl Pts',(1.42945722054536,3.07365744608497,-32.9182160557564));
#30009=CARTESIAN_POINT('Ctrl Pts',(1.41339738655488,3.08107543640678,-32.9171726594546));
#30010=CARTESIAN_POINT('Ctrl Pts',(1.37722681499142,3.09744020020741,-32.9148139476308));
#30011=CARTESIAN_POINT('Ctrl Pts',(1.35708660065256,3.1063170145883,-32.9134948557009));
#30012=CARTESIAN_POINT('Ctrl Pts',(1.29414286192117,3.13333055459123,-32.90935778409));
#30013=CARTESIAN_POINT('Ctrl Pts',(1.25105327837817,3.15078265804886,-32.9065049328919));
#30014=CARTESIAN_POINT('Ctrl Pts',(1.14541285191986,3.19106045729588,-32.8994835351815));
#30015=CARTESIAN_POINT('Ctrl Pts',(1.08252257160822,3.21293969093737,-32.8952809260689));
#30016=CARTESIAN_POINT('Ctrl Pts',(0.777370039512734,3.30912431481032,-32.8749017878759));
#30017=CARTESIAN_POINT('Ctrl Pts',(0.527896504186848,3.35796886294455,-32.8583562129981));
#30018=CARTESIAN_POINT('Ctrl Pts',(0.17990431218647,3.38632571147815,-32.8365393294357));
#30019=CARTESIAN_POINT('Ctrl Pts',(0.0842079902564654,3.39005590231105,
-32.830658542228));
#30020=CARTESIAN_POINT('Ctrl Pts',(-0.0495985192761317,3.38960095676014,
-32.8226064202216));
#30021=CARTESIAN_POINT('Ctrl Pts',(-0.087668078497511,3.38883005523327,
-32.8203345422437));
#30022=CARTESIAN_POINT('Ctrl Pts',(-0.157433144747235,3.38624085355091,
-32.8162046717881));
#30023=CARTESIAN_POINT('Ctrl Pts',(-0.1891311919983,3.38461841379444,-32.8143409386869));
#30024=CARTESIAN_POINT('Ctrl Pts',(-0.25405906147528,3.38038012074537,-32.8105478928362));
#30025=CARTESIAN_POINT('Ctrl Pts',(-0.287282511437232,3.37771885157417,
-32.8086201810603));
#30026=CARTESIAN_POINT('Ctrl Pts',(-0.372205990094181,3.36965418544892,
-32.8037233990268));
#30027=CARTESIAN_POINT('Ctrl Pts',(-0.42383169661312,3.36355076122683,-32.8007759079591));
#30028=CARTESIAN_POINT('Ctrl Pts',(-0.673641776112479,3.32817379114229,
-32.7866261091439));
#30029=CARTESIAN_POINT('Ctrl Pts',(-0.869110742142148,3.28255858320625,
-32.7759302171727));
#30030=CARTESIAN_POINT('Ctrl Pts',(-1.26049061512538,3.15378716126089,-32.7540579221479));
#30031=CARTESIAN_POINT('Ctrl Pts',(-1.45489817716245,3.06895119036221,-32.7429292510127));
#30032=CARTESIAN_POINT('Ctrl Pts',(-1.67100262171976,2.94947485907622,-32.7289697065074));
#30033=CARTESIAN_POINT('Ctrl Pts',(-1.70163241128534,2.93191040756535,-32.7269507652376));
#30034=CARTESIAN_POINT('Ctrl Pts',(-1.74903570035984,2.90373428665369,-32.7237538429069));
#30035=CARTESIAN_POINT('Ctrl Pts',(-1.76600063746828,2.89344783859725,-32.7225949434459));
#30036=CARTESIAN_POINT('Ctrl Pts',(-1.79834455594705,2.8734461530914,-32.7203551105036));
#30037=CARTESIAN_POINT('Ctrl Pts',(-1.81373722503326,2.86375507991179,-32.7192756141966));
#30038=CARTESIAN_POINT('Ctrl Pts',(-1.85200492281088,2.83922985079057,-32.7165591055902));
#30039=CARTESIAN_POINT('Ctrl Pts',(-1.87478013897929,2.82424285554802,-32.7149128092817));
#30040=CARTESIAN_POINT('Ctrl Pts',(-1.96798067435477,2.76128910996908,-32.7080610152107));
#30041=CARTESIAN_POINT('Ctrl Pts',(-2.03676150607504,2.71095294159866,-32.7027309399712));
#30042=CARTESIAN_POINT('Ctrl Pts',(-2.24534396095765,2.54588390676022,-32.6858615489026));
#30043=CARTESIAN_POINT('Ctrl Pts',(-2.3779150878297,2.42252233708731,-32.6741084802996));
#30044=CARTESIAN_POINT('Ctrl Pts',(-2.61379999917827,2.16491184293108,-32.6517737266632));
#30045=CARTESIAN_POINT('Ctrl Pts',(-2.71817304432898,2.03232424853033,-32.6411967970714));
#30046=CARTESIAN_POINT('Ctrl Pts',(-2.8393777943812,1.85221424424317,-32.6280489941279));
#30047=CARTESIAN_POINT('Ctrl Pts',(-2.86562505852472,1.81134128587344,-32.6251385359313));
#30048=CARTESIAN_POINT('Ctrl Pts',(-2.90634038473951,1.74483678140426,-32.6205166987396));
#30049=CARTESIAN_POINT('Ctrl Pts',(-2.92136814978037,1.7195575128752,-32.6187854777751));
#30050=CARTESIAN_POINT('Ctrl Pts',(-2.95209327289725,1.66630696386272,-32.6151906042328));
#30051=CARTESIAN_POINT('Ctrl Pts',(-2.96772648642255,1.63830192397688,-32.6133293418135));
#30052=CARTESIAN_POINT('Ctrl Pts',(-3.00445897765211,1.57024837133797,-32.608874096377));
#30053=CARTESIAN_POINT('Ctrl Pts',(-3.02515840316091,1.52999039336254,-32.6062940755834));
#30054=CARTESIAN_POINT('Ctrl Pts',(-3.10241675143629,1.37202979350173,-32.5963696053623));
#30055=CARTESIAN_POINT('Ctrl Pts',(-3.15296491172492,1.25150804308817,-32.5892242917128));
#30056=CARTESIAN_POINT('Ctrl Pts',(-3.25034058446021,0.975660823085285,
-32.5734851217536));
#30057=CARTESIAN_POINT('Ctrl Pts',(-3.29323273681335,0.819296151041877,
-32.564979006293));
#30058=CARTESIAN_POINT('Ctrl Pts',(-3.32508144317155,0.658969485091512,
-32.5562530931637));
#30059=CARTESIAN_POINT('Ctrl Pts',(-3.32537743267149,0.657474194383888,
-32.5561717093476));
#30060=CARTESIAN_POINT('Ctrl Pts',(-3.33982528833165,0.584226641344357,
-32.5521849965956));
#30061=CARTESIAN_POINT('Ctrl Pts',(-3.35165186773748,0.512037809713025,
-32.5482521781375));
#30062=CARTESIAN_POINT('Ctrl Pts',(-3.37093460479456,0.364579209396957,
-32.5401177403836));
#30063=CARTESIAN_POINT('Ctrl Pts',(-3.37822501044656,0.289330795697706,
-32.5359138068072));
#30064=CARTESIAN_POINT('Ctrl Pts',(-3.38465642193842,0.187616451665435,
-32.5300873279099));
#30065=CARTESIAN_POINT('Ctrl Pts',(-3.38601220147362,0.161308114618323,
-32.5285673520936));
#30066=CARTESIAN_POINT('Ctrl Pts',(-3.38777324823923,0.117120526173392,
-32.5259887268538));
#30067=CARTESIAN_POINT('Ctrl Pts',(-3.38834392234425,0.0992484370684867,
-32.5249387123237));
#30068=CARTESIAN_POINT('Ctrl Pts',(-3.38911919979665,0.0669619443574267,
-32.5230278783059));
#30069=CARTESIAN_POINT('Ctrl Pts',(-3.38937330428478,0.0525494048286926,
-32.5221699614643));
#30070=CARTESIAN_POINT('Ctrl Pts',(-3.38967720194844,0.025538900972615,
-32.5205534547019));
#30071=CARTESIAN_POINT('Ctrl Pts',(-3.38974870430922,0.0129413635074798,
-32.5197959849455));
#30072=CARTESIAN_POINT('Ctrl Pts',(-3.38974998254981,0.000343952908442827,
-32.5190351755825));
#30073=CARTESIAN_POINT('',(-3.38974872454211,-0.00294057224222385,-30.0160178032104));
#30074=CARTESIAN_POINT('Ctrl Pts',(-3.38974998234963,0.000345920085544606,
-32.5190352943883));
#30075=CARTESIAN_POINT('Ctrl Pts',(-3.38975151971354,-0.0147190602479393,
-32.5181254587716));
#30076=CARTESIAN_POINT('Ctrl Pts',(-3.38965262764753,-0.0297836515172151,
-32.5172108597942));
#30077=CARTESIAN_POINT('Ctrl Pts',(-3.38910134638758,-0.0714486137903887,
-32.5146689626663));
#30078=CARTESIAN_POINT('Ctrl Pts',(-3.38843622082854,-0.0980445619635314,
-32.5130324841435));
#30079=CARTESIAN_POINT('Ctrl Pts',(-3.38310214657387,-0.24302633539895,
-32.5040452157681));
#30080=CARTESIAN_POINT('Ctrl Pts',(-3.37254214438138,-0.361106114222097,
-32.4964868766424));
#30081=CARTESIAN_POINT('Ctrl Pts',(-3.31992162810586,-0.730236373057563,
-32.4725274243699));
#30082=CARTESIAN_POINT('Ctrl Pts',(-3.25577428233754,-0.977288287365443,
-32.4560766797842));
#30083=CARTESIAN_POINT('Ctrl Pts',(-3.14088421989889,-1.27656623872225,
-32.4363955308566));
#30084=CARTESIAN_POINT('Ctrl Pts',(-3.11539122277617,-1.33757746549877,
-32.4323913716381));
#30085=CARTESIAN_POINT('Ctrl Pts',(-3.07323823294502,-1.43070464592318,
-32.426289868579));
#30086=CARTESIAN_POINT('Ctrl Pts',(-3.05782253215433,-1.46336274807284,
-32.4241521218584));
#30087=CARTESIAN_POINT('Ctrl Pts',(-3.02808668173032,-1.52383538469427,
-32.420195677516));
#30088=CARTESIAN_POINT('Ctrl Pts',(-3.01389780054778,-1.55170982325741,
-32.4183727837166));
#30089=CARTESIAN_POINT('Ctrl Pts',(-2.98103854325281,-1.6141110811488,-32.4142918379305));
#30090=CARTESIAN_POINT('Ctrl Pts',(-2.96215004564179,-1.64851832480108,
-32.4120415954188));
#30091=CARTESIAN_POINT('Ctrl Pts',(-2.90109981451286,-1.75528851497847,
-32.4050514933619));
#30092=CARTESIAN_POINT('Ctrl Pts',(-2.85685035878308,-1.82642421983521,
-32.4003844402938));
#30093=CARTESIAN_POINT('Ctrl Pts',(-2.66269852626281,-2.11419371528011,
-32.3813320629483));
#30094=CARTESIAN_POINT('Ctrl Pts',(-2.49045186970781,-2.31461078277455,
-32.3677164724198));
#30095=CARTESIAN_POINT('Ctrl Pts',(-2.24337340630939,-2.54223262717457,
-32.3495979173992));
#30096=CARTESIAN_POINT('Ctrl Pts',(-2.18844024476452,-2.58967164110989,
-32.3456386241792));
#30097=CARTESIAN_POINT('Ctrl Pts',(-2.0936412999557,-2.66636633690654,-32.3388403996283));
#30098=CARTESIAN_POINT('Ctrl Pts',(-2.05458039961716,-2.69657972356982,
-32.336048410294));
#30099=CARTESIAN_POINT('Ctrl Pts',(-1.99676715231779,-2.73931251908909,
-32.3319068937879));
#30100=CARTESIAN_POINT('Ctrl Pts',(-1.97852624161241,-2.75251630138135,
-32.3305988955317));
#30101=CARTESIAN_POINT('Ctrl Pts',(-1.94573637166981,-2.77575708617915,
-32.3282427403961));
#30102=CARTESIAN_POINT('Ctrl Pts',(-1.93123837070507,-2.78586355586294,
-32.3271991307333));
#30103=CARTESIAN_POINT('Ctrl Pts',(-1.89786797103962,-2.80874018489604,
-32.3247927102158));
#30104=CARTESIAN_POINT('Ctrl Pts',(-1.87894531895663,-2.82143379993151,
-32.323425287011));
#30105=CARTESIAN_POINT('Ctrl Pts',(-1.81729893291112,-2.86189199647878,
-32.318964980714));
#30106=CARTESIAN_POINT('Ctrl Pts',(-1.77407850648132,-2.88888319078675,
-32.315829462847));
#30107=CARTESIAN_POINT('Ctrl Pts',(-1.4918076705427,-3.05643827710386,-32.2953771169475));
#30108=CARTESIAN_POINT('Ctrl Pts',(-1.23687917387077,-3.16819295326867,
-32.2771270209124));
#30109=CARTESIAN_POINT('Ctrl Pts',(-0.850753381473515,-3.28365985675345,
-32.2516615987019));
#30110=CARTESIAN_POINT('Ctrl Pts',(-0.728411976184832,-3.31294809311484,
-32.2438700378893));
#30111=CARTESIAN_POINT('Ctrl Pts',(-0.560656866619073,-3.34336265233418,
-32.2335828126538));
#30112=CARTESIAN_POINT('Ctrl Pts',(-0.516443766568526,-3.35047699128768,
-32.2309076030414));
#30113=CARTESIAN_POINT('Ctrl Pts',(-0.440424128754461,-3.36116868443577,
-32.2263674332771));
#30114=CARTESIAN_POINT('Ctrl Pts',(-0.408684962785469,-3.36517533621465,
-32.2244895101848));
#30115=CARTESIAN_POINT('Ctrl Pts',(-0.343581202104071,-3.37245913042291,
-32.2206719825815));
#30116=CARTESIAN_POINT('Ctrl Pts',(-0.310215131144468,-3.37569182795055,
-32.2187339399547));
#30117=CARTESIAN_POINT('Ctrl Pts',(-0.224031479536461,-3.38275313537361,
-32.213772409949));
#30118=CARTESIAN_POINT('Ctrl Pts',(-0.171161347240629,-3.38584008708192,
-32.2107716907595));
#30119=CARTESIAN_POINT('Ctrl Pts',(0.152403171726233,-3.39713327359408,
-32.192629532053));
#30120=CARTESIAN_POINT('Ctrl Pts',(0.423194586134779,-3.37411556981751,
-32.1784944292937));
#30121=CARTESIAN_POINT('Ctrl Pts',(0.832448089137162,-3.28923784710404,
-32.156205297257));
#30122=CARTESIAN_POINT('Ctrl Pts',(0.974410596902226,-3.25001088267025,
-32.1482686350341));
#30123=CARTESIAN_POINT('Ctrl Pts',(1.14268809315137,-3.19149386898141,-32.1381440005817));
#30124=CARTESIAN_POINT('Ctrl Pts',(1.17187332846928,-3.18089326320842,-32.1363609225856));
#30125=CARTESIAN_POINT('Ctrl Pts',(1.2186235246861,-3.16318204707204,-32.1334546956653));
#30126=CARTESIAN_POINT('Ctrl Pts',(1.23628229264225,-3.15632222898905,-32.1323453129663));
#30127=CARTESIAN_POINT('Ctrl Pts',(1.27135219907536,-3.1423593414256,-32.1301171321725));
#30128=CARTESIAN_POINT('Ctrl Pts',(1.28876355065354,-3.13525869979164,-32.1289984872903));
#30129=CARTESIAN_POINT('Ctrl Pts',(1.33415312945107,-3.11630610314004,-32.1260514332473));
#30130=CARTESIAN_POINT('Ctrl Pts',(1.36203211367256,-3.10422239592704,-32.1242103959884));
#30131=CARTESIAN_POINT('Ctrl Pts',(1.50044861992926,-3.04200440081785,-32.1149279386334));
#30132=CARTESIAN_POINT('Ctrl Pts',(1.60839185426979,-2.98633679156353,-32.1072358396914));
#30133=CARTESIAN_POINT('Ctrl Pts',(1.89121686555835,-2.82069285590838,-32.086233579308));
#30134=CARTESIAN_POINT('Ctrl Pts',(2.05944080312321,-2.70031919651049,-32.0728324592527));
#30135=CARTESIAN_POINT('Ctrl Pts',(2.30078306400376,-2.49187677696339,-32.0527815041129));
#30136=CARTESIAN_POINT('Ctrl Pts',(2.38218971825948,-2.41417250712736,-32.0458398222432));
#30137=CARTESIAN_POINT('Ctrl Pts',(2.48938838697,-2.30113577159368,-32.0364544963012));
#30138=CARTESIAN_POINT('Ctrl Pts',(2.51858351714032,-2.2691447081807,-32.0338704792926));
#30139=CARTESIAN_POINT('Ctrl Pts',(2.56811024884799,-2.21274108673938,-32.0294354746061));
#30140=CARTESIAN_POINT('Ctrl Pts',(2.58872602650768,-2.18858653663426,-32.0275730486659));
#30141=CARTESIAN_POINT('Ctrl Pts',(2.63071460277566,-2.1379669255012,-32.0237438125809));
#30142=CARTESIAN_POINT('Ctrl Pts',(2.65203462269421,-2.11146261552585,-32.021779218035));
#30143=CARTESIAN_POINT('Ctrl Pts',(2.70704039947975,-2.0409335290338,-32.0166528116558));
#30144=CARTESIAN_POINT('Ctrl Pts',(2.74005214706653,-1.9963947773594,-32.0135168930657));
#30145=CARTESIAN_POINT('Ctrl Pts',(2.90905725893796,-1.75628223338974,-31.9970972469591));
#30146=CARTESIAN_POINT('Ctrl Pts',(3.02524537975443,-1.54759234531545,-31.9845509433189));
#30147=CARTESIAN_POINT('Ctrl Pts',(3.16517969934154,-1.21908522433469,-31.965579495503));
#30148=CARTESIAN_POINT('Ctrl Pts',(3.205972530853,-1.10737005535036,-31.9592385609194));
#30149=CARTESIAN_POINT('Ctrl Pts',(3.25455517536627,-0.948932646057613,
-31.9501262309488));
#30150=CARTESIAN_POINT('Ctrl Pts',(3.26736618886803,-0.903836477129002,
-31.9475191588104));
#30151=CARTESIAN_POINT('Ctrl Pts',(3.28835846768625,-0.823650830252975,
-31.942837139873));
#30152=CARTESIAN_POINT('Ctrl Pts',(3.29692331742208,-0.788668830872896,
-31.940779141611));
#30153=CARTESIAN_POINT('Ctrl Pts',(3.30937183520242,-0.734072585114871,
-31.9375341131935));
#30154=CARTESIAN_POINT('Ctrl Pts',(3.31364228905111,-0.714548277460725,
-31.9363671122508));
#30155=CARTESIAN_POINT('Ctrl Pts',(3.32141282648714,-0.677453212267713,
-31.9341355646797));
#30156=CARTESIAN_POINT('Ctrl Pts',(3.32494666421573,-0.659890629650698,
-31.9330728304017));
#30157=CARTESIAN_POINT('Ctrl Pts',(3.33258300824863,-0.620319869497174,
-31.9306654097903));
#30158=CARTESIAN_POINT('Ctrl Pts',(3.33660701655666,-0.598297423062006,
-31.9293166849474));
#30159=CARTESIAN_POINT('Ctrl Pts',(3.35062524030221,-0.517034646906688,
-31.9243110963898));
#30160=CARTESIAN_POINT('Ctrl Pts',(3.35926169643006,-0.457574364224408,
-31.9205924114407));
#30161=CARTESIAN_POINT('Ctrl Pts',(3.39743511407486,-0.134635786069528,
-31.9002004799878));
#30162=CARTESIAN_POINT('Ctrl Pts',(3.39756389851286,0.1313917637633,-31.8827908067997));
#30163=CARTESIAN_POINT('Ctrl Pts',(3.35225191822044,0.517863932089777,-31.8582184823072));
#30164=CARTESIAN_POINT('Ctrl Pts',(3.33106915431097,0.640124794758583,-31.850537157987));
#30165=CARTESIAN_POINT('Ctrl Pts',(3.29322028354437,0.804421689542251,-31.8403658271591));
#30166=CARTESIAN_POINT('Ctrl Pts',(3.28235135109967,0.847681532885321,-31.8377016180511));
#30167=CARTESIAN_POINT('Ctrl Pts',(3.26223363223903,0.921552051855528,-31.8331741912953));
#30168=CARTESIAN_POINT('Ctrl Pts',(3.25339990815082,0.952268657884555,-31.8312981964903));
#30169=CARTESIAN_POINT('Ctrl Pts',(3.23439814928035,1.01498811684034,-31.8274796076031));
#30170=CARTESIAN_POINT('Ctrl Pts',(3.22418635551133,1.04697408130729,-31.8255386502022));
#30171=CARTESIAN_POINT('Ctrl Pts',(3.19656176751911,1.12926117191592,-31.8205589283141));
#30172=CARTESIAN_POINT('Ctrl Pts',(3.17843613728034,1.17931424088149,-31.8175432698798));
#30173=CARTESIAN_POINT('Ctrl Pts',(3.06606107300469,1.46819220847407,-31.8001782209697));
#30174=CARTESIAN_POINT('Ctrl Pts',(2.94610490198888,1.69611166540161,-31.7867171792342));
#30175=CARTESIAN_POINT('Ctrl Pts',(2.71865546621671,2.03002560661381,-31.7652171753579));
#30176=CARTESIAN_POINT('Ctrl Pts',(2.627915131404,2.14619332135222,-31.757316805065));
#30177=CARTESIAN_POINT('Ctrl Pts',(2.50426879268441,2.28484754334589,-31.7468520104919));
#30178=CARTESIAN_POINT('Ctrl Pts',(2.47812974048097,2.31317167783212,-31.744654557653));
#30179=CARTESIAN_POINT('Ctrl Pts',(2.43735725880367,2.35586817983901,-31.7412380095916));
#30180=CARTESIAN_POINT('Ctrl Pts',(2.42306607845527,2.37056449416151,-31.7400424866073));
#30181=CARTESIAN_POINT('Ctrl Pts',(2.3960218696451,2.39787530923101,-31.7377817819865));
#30182=CARTESIAN_POINT('Ctrl Pts',(2.38330065572409,2.41051959691851,-31.7367188688881));
#30183=CARTESIAN_POINT('Ctrl Pts',(2.35499716151906,2.43820888754345,-31.7343558485799));
#30184=CARTESIAN_POINT('Ctrl Pts',(2.33936989640805,2.45320660461194,-31.7330524615085));
#30185=CARTESIAN_POINT('Ctrl Pts',(2.28458935125208,2.50478089936443,-31.7284914248393));
#30186=CARTESIAN_POINT('Ctrl Pts',(2.24471508978919,2.54057658310158,-31.725185388131));
#30187=CARTESIAN_POINT('Ctrl Pts',(1.99711839932039,2.75246749035028,-31.704825440136));
#30188=CARTESIAN_POINT('Ctrl Pts',(1.76964422816903,2.90395081557588,-31.6869201017299));
#30189=CARTESIAN_POINT('Ctrl Pts',(1.41486497211439,3.08288678069223,-31.6618189514095));
#30190=CARTESIAN_POINT('Ctrl Pts',(1.30020588933392,3.1329704842609,-31.654070958215));
#30191=CARTESIAN_POINT('Ctrl Pts',(1.14113539300481,3.19221141665818,-31.6438294989835));
#30192=CARTESIAN_POINT('Ctrl Pts',(1.09893419962264,3.20698419445037,-31.6411586085529));
#30193=CARTESIAN_POINT('Ctrl Pts',(1.02606713926823,3.23088437154998,-31.6366234440141));
#30194=CARTESIAN_POINT('Ctrl Pts',(0.995542485260382,3.24042016726061,-31.6347462799687));
#30195=CARTESIAN_POINT('Ctrl Pts',(0.932733427338256,3.25907017390353,-31.6309283468252));
#30196=CARTESIAN_POINT('Ctrl Pts',(0.900439463139534,3.26813998084528,-31.6289891688546));
#30197=CARTESIAN_POINT('Ctrl Pts',(0.816726664639992,3.2903157508031,-31.624020548206));
#30198=CARTESIAN_POINT('Ctrl Pts',(0.765124283453533,3.30269669230534,-31.6210140052148));
#30199=CARTESIAN_POINT('Ctrl Pts',(0.4297043246537,3.37488994330375,-31.6017898870362));
#30200=CARTESIAN_POINT('Ctrl Pts',(0.139512299108629,3.39927465568513,-31.5867512803949));
#30201=CARTESIAN_POINT('Ctrl Pts',(-0.279219414748744,3.38069633815382,
-31.5643070827361));
#30202=CARTESIAN_POINT('Ctrl Pts',(-0.40774617734941,3.36761161432466,-31.5572936131331));
#30203=CARTESIAN_POINT('Ctrl Pts',(-0.565179005201581,3.34243914711843,
-31.5482249953726));
#30204=CARTESIAN_POINT('Ctrl Pts',(-0.595090835820295,3.33724340164118,
-31.546480284736));
#30205=CARTESIAN_POINT('Ctrl Pts',(-0.643403867305303,3.32818117059328,
-31.5436212676159));
#30206=CARTESIAN_POINT('Ctrl Pts',(-0.661850424346191,3.32456198972908,
-31.542519923956));
#30207=CARTESIAN_POINT('Ctrl Pts',(-0.698830184186938,3.31698666663779,
-31.5402907814393));
#30208=CARTESIAN_POINT('Ctrl Pts',(-0.717362173257835,3.31302816883222,
-31.5391629042066));
#30209=CARTESIAN_POINT('Ctrl Pts',(-0.766195590686987,3.30216825295493,
-31.5361641317044));
#30210=CARTESIAN_POINT('Ctrl Pts',(-0.796436324362887,3.29500529393247,
-31.5342798378231));
#30211=CARTESIAN_POINT('Ctrl Pts',(-0.966538458874326,3.25223573177051,
-31.5235426059));
#30212=CARTESIAN_POINT('Ctrl Pts',(-1.10410178664264,3.20814367359347,-31.5143353183145));
#30213=CARTESIAN_POINT('Ctrl Pts',(-1.4137763253231,3.08660436933167,-31.4929471636992));
#30214=CARTESIAN_POINT('Ctrl Pts',(-1.58310081161304,3.00328010318528,-31.4807663393065));
#30215=CARTESIAN_POINT('Ctrl Pts',(-1.83694710054287,2.85089871606752,-31.4621868410934));
#30216=CARTESIAN_POINT('Ctrl Pts',(-1.92657626219327,2.79111191646911,-31.4555516579836));
#30217=CARTESIAN_POINT('Ctrl Pts',(-2.04757908680858,2.70178633571687,-31.4464964842643));
#30218=CARTESIAN_POINT('Ctrl Pts',(-2.08146204766934,2.67577007855744,-31.4439491146149));
#30219=CARTESIAN_POINT('Ctrl Pts',(-2.13959288511099,2.62936305968285,-31.4395560183774));
#30220=CARTESIAN_POINT('Ctrl Pts',(-2.1640628729233,2.60926039257545,-31.437699457054));
#30221=CARTESIAN_POINT('Ctrl Pts',(-2.2143989852583,2.56671281344454,-31.4338634098585));
#30222=CARTESIAN_POINT('Ctrl Pts',(-2.24021398478587,2.54421283666147,-31.43188642674));
#30223=CARTESIAN_POINT('Ctrl Pts',(-2.30776730045797,2.48350884524459,-31.4266834914391));
#30224=CARTESIAN_POINT('Ctrl Pts',(-2.34889843289533,2.44464368757765,-31.423484932569));
#30225=CARTESIAN_POINT('Ctrl Pts',(-2.54717917518094,2.24765963631828,-31.4078699265141));
#30226=CARTESIAN_POINT('Ctrl Pts',(-2.68943915218223,2.07533677068973,-31.3960814686697));
#30227=CARTESIAN_POINT('Ctrl Pts',(-2.88514301046738,1.78402392867721,-31.3774518676823));
#30228=CARTESIAN_POINT('Ctrl Pts',(-2.95044718856002,1.67381286684701,-31.3706453191104));
#30229=CARTESIAN_POINT('Ctrl Pts',(-3.04205500627029,1.49711477012226,-31.3597219688441));
#30230=CARTESIAN_POINT('Ctrl Pts',(-3.07275806088825,1.4330414655169,-31.3557581511853));
#30231=CARTESIAN_POINT('Ctrl Pts',(-3.11179268219523,1.34454879119662,-31.3502185318787));
#30232=CARTESIAN_POINT('Ctrl Pts',(-3.12189375193288,1.32092560914252,-31.3487335402309));
#30233=CARTESIAN_POINT('Ctrl Pts',(-3.13858774022151,1.28062237411466,-31.3461858765785));
#30234=CARTESIAN_POINT('Ctrl Pts',(-3.1453184926567,1.26400088530767,-31.3451310915843));
#30235=CARTESIAN_POINT('Ctrl Pts',(-3.15946450275532,1.22825477427803,-31.3428527810384));
#30236=CARTESIAN_POINT('Ctrl Pts',(-3.16683821919544,1.20911595026986,-31.3416271758218));
#30237=CARTESIAN_POINT('Ctrl Pts',(-3.18720438822845,1.15479009275808,-31.3381343733759));
#30238=CARTESIAN_POINT('Ctrl Pts',(-3.19978675257161,1.11945364383098,-31.3358460998761));
#30239=CARTESIAN_POINT('Ctrl Pts',(-3.25740035908007,0.948737477520367,
-31.3247368281054));
#30240=CARTESIAN_POINT('Ctrl Pts',(-3.29443792279989,0.810822123735642,
-31.3156054528134));
#30241=CARTESIAN_POINT('Ctrl Pts',(-3.34674789599764,0.551790708433814,
-31.2985999385216));
#30242=CARTESIAN_POINT('Ctrl Pts',(-3.36438901312496,0.431372879284578,
-31.2907501180964));
#30243=CARTESIAN_POINT('Ctrl Pts',(-3.38493988534087,0.20779045872944,-31.2764460155949));
#30244=CARTESIAN_POINT('Ctrl Pts',(-3.38968826149535,0.104933788933924,
-31.2699692516742));
#30245=CARTESIAN_POINT('Ctrl Pts',(-3.38979385698205,-0.0728188464554172,
-31.2589960814788));
#30246=CARTESIAN_POINT('Ctrl Pts',(-3.38736030023665,-0.147636275167262,
-31.2544439856543));
#30247=CARTESIAN_POINT('Ctrl Pts',(-3.3799777540892,-0.259958664242163,
-31.2477087911456));
#30248=CARTESIAN_POINT('Ctrl Pts',(-3.3768754011307,-0.297558098380861,
-31.2454707990118));
#30249=CARTESIAN_POINT('Ctrl Pts',(-3.3700604981018,-0.366157697312476,
-31.2414162325367));
#30250=CARTESIAN_POINT('Ctrl Pts',(-3.3665461481857,-0.397172944746368,
-31.2395938076593));
#30251=CARTESIAN_POINT('Ctrl Pts',(-3.35788342164304,-0.465210476368273,
-31.2356177905748));
#30252=CARTESIAN_POINT('Ctrl Pts',(-3.35255004886927,-0.502205324968264,
-31.233470124624));
#30253=CARTESIAN_POINT('Ctrl Pts',(-3.33501390700637,-0.611064454422087,
-31.227187101642));
#30254=CARTESIAN_POINT('Ctrl Pts',(-3.32110365733512,-0.682633908516753,
-31.2231040606011));
#30255=CARTESIAN_POINT('Ctrl Pts',(-3.28287462343786,-0.850263589851162,
-31.2136076618927));
#30256=CARTESIAN_POINT('Ctrl Pts',(-3.25663117512684,-0.945816613963547,
-31.2082480238829));
#30257=CARTESIAN_POINT('Ctrl Pts',(-3.18734777525435,-1.16072630669105,
-31.1961568670839));
#30258=CARTESIAN_POINT('Ctrl Pts',(-3.14171992980308,-1.27908853430591,
-31.1894721588661));
#30259=CARTESIAN_POINT('Ctrl Pts',(-3.03017314661259,-1.52620404824792,
-31.1750364905036));
#30260=CARTESIAN_POINT('Ctrl Pts',(-2.96243489678285,-1.65385008477966,
-31.1672810596357));
#30261=CARTESIAN_POINT('Ctrl Pts',(-2.86708023764613,-1.80877519681317,
-31.1570278564257));
#30262=CARTESIAN_POINT('Ctrl Pts',(-2.84685603117243,-1.84044214728108,
-31.1548849091984));
#30263=CARTESIAN_POINT('Ctrl Pts',(-2.81477756377269,-1.88887626923582,
-31.1515231625217));
#30264=CARTESIAN_POINT('Ctrl Pts',(-2.80328972537393,-1.90588377483582,
-31.1503262756566));
#30265=CARTESIAN_POINT('Ctrl Pts',(-2.78147809194234,-1.93755158959592,
-31.1480646615379));
#30266=CARTESIAN_POINT('Ctrl Pts',(-2.77119133144748,-1.952235919978,-31.1470022325769));
#30267=CARTESIAN_POINT('Ctrl Pts',(-2.74589752158615,-1.9877400555362,-31.1444007790509));
#30268=CARTESIAN_POINT('Ctrl Pts',(-2.73076978621036,-2.00847205979082,
-31.1428541362297));
#30269=CARTESIAN_POINT('Ctrl Pts',(-2.67302123364847,-2.08575576116977,
-31.1369902723998));
#30270=CARTESIAN_POINT('Ctrl Pts',(-2.62886948022658,-2.14113602896012,
-31.1325876610165));
#30271=CARTESIAN_POINT('Ctrl Pts',(-2.50057659895951,-2.29210164758648,
-31.1201008439151));
#30272=CARTESIAN_POINT('Ctrl Pts',(-2.41273708626509,-2.3843889440527,-31.11189525565));
#30273=CARTESIAN_POINT('Ctrl Pts',(-2.15660742127133,-2.62480849445823,
-31.0892696180546));
#30274=CARTESIAN_POINT('Ctrl Pts',(-1.97848156117016,-2.76155976973937,
-31.0749557831196));
#30275=CARTESIAN_POINT('Ctrl Pts',(-1.74012771650372,-2.90956270561394,
-31.0578493421647));
#30276=CARTESIAN_POINT('Ctrl Pts',(-1.69137096811816,-2.93817365481448,
-31.0544441629388));
#30277=CARTESIAN_POINT('Ctrl Pts',(-1.61197293424524,-2.98213346563277,
-31.0490453406497));
#30278=CARTESIAN_POINT('Ctrl Pts',(-1.58177641138783,-2.99825953843388,
-31.0470249721748));
#30279=CARTESIAN_POINT('Ctrl Pts',(-1.52318100968024,-3.02841999715123,
-31.0431657423445));
#30280=CARTESIAN_POINT('Ctrl Pts',(-1.49481965507596,-3.04251908216918,
-31.0413248026946));
#30281=CARTESIAN_POINT('Ctrl Pts',(-1.42772787918613,-3.07470730768495,
-31.0370306620228));
#30282=CARTESIAN_POINT('Ctrl Pts',(-1.3888442303788,-3.09246566025329,-31.0345887918594));
#30283=CARTESIAN_POINT('Ctrl Pts',(-1.25065984687188,-3.15244290847438,
-31.0260636256352));
#30284=CARTESIAN_POINT('Ctrl Pts',(-1.14968624739726,-3.19065366171112,
-31.0201103846451));
#30285=CARTESIAN_POINT('Ctrl Pts',(-0.867134331467032,-3.28241815109112,
-31.0039929771783));
#30286=CARTESIAN_POINT('Ctrl Pts',(-0.682640247903144,-3.32568702675918,
-30.9940776699118));
#30287=CARTESIAN_POINT('Ctrl Pts',(-0.353777072665913,-3.3742806976672,
-30.9763369476531));
#30288=CARTESIAN_POINT('Ctrl Pts',(-0.210884370300202,-3.38621442189802,
-30.9685988550972));
#30289=CARTESIAN_POINT('Ctrl Pts',(-0.0366170520661458,-3.38969462241773,
-30.9586938126423));
#30290=CARTESIAN_POINT('Ctrl Pts',(-0.00554678726381804,-3.38988783451179,
-30.9569096196713));
#30291=CARTESIAN_POINT('Ctrl Pts',(0.0444688304589123,-3.38951126902333,
-30.9540020189534));
#30292=CARTESIAN_POINT('Ctrl Pts',(0.0634150740758199,-3.38920973245243,
-30.952892400916));
#30293=CARTESIAN_POINT('Ctrl Pts',(0.101151720335835,-3.38829261295725,
-30.950664219388));
#30294=CARTESIAN_POINT('Ctrl Pts',(0.119941480844943,-3.38767951582361,
-30.9495458157444));
#30295=CARTESIAN_POINT('Ctrl Pts',(0.169065348107693,-3.3856674489129,-30.9466001496575));
#30296=CARTESIAN_POINT('Ctrl Pts',(0.199386880875708,-3.38401712455632,
-30.9447602798778));
#30297=CARTESIAN_POINT('Ctrl Pts',(0.358621538985245,-3.37320292966175,
-30.9349982333533));
#30298=CARTESIAN_POINT('Ctrl Pts',(0.486945130178296,-3.35707998583838,
-30.9267903019519));
#30299=CARTESIAN_POINT('Ctrl Pts',(0.898948223787798,-3.28119397567878,
-30.8999118934604));
#30300=CARTESIAN_POINT('Ctrl Pts',(1.17602920784825,-3.1923896776265,-30.8811395999651));
#30301=CARTESIAN_POINT('Ctrl Pts',(1.48654697431218,-3.04686791706524,-30.8602883492586));
#30302=CARTESIAN_POINT('Ctrl Pts',(1.53410575535585,-3.02320128617517,-30.8570953911699));
#30303=CARTESIAN_POINT('Ctrl Pts',(1.61076928485538,-2.98277607231283,-30.8519470839224));
#30304=CARTESIAN_POINT('Ctrl Pts',(1.64021452933924,-2.96668623292598,-30.8499693252217));
#30305=CARTESIAN_POINT('Ctrl Pts',(1.69724219777491,-2.93441581226866,-30.8461366071284));
#30306=CARTESIAN_POINT('Ctrl Pts',(1.72484405320441,-2.91827694557501,-30.8442804495745));
#30307=CARTESIAN_POINT('Ctrl Pts',(1.79045444548963,-2.87865827583648,-30.8398632985484));
#30308=CARTESIAN_POINT('Ctrl Pts',(1.82823571109384,-2.85481260980144,-30.8373156410031));
#30309=CARTESIAN_POINT('Ctrl Pts',(1.96963375714398,-2.7616104762695,-30.8277515771831));
#30310=CARTESIAN_POINT('Ctrl Pts',(2.06987222650949,-2.68730026220169,-30.8209148612623));
#30311=CARTESIAN_POINT('Ctrl Pts',(2.37343823670961,-2.43517017810186,-30.7996416203131));
#30312=CARTESIAN_POINT('Ctrl Pts',(2.55971696357321,-2.23854577817081,-30.7857669976423));
#30313=CARTESIAN_POINT('Ctrl Pts',(2.75383891590257,-1.97733759359598,-30.7677347445065));
#30314=CARTESIAN_POINT('Ctrl Pts',(2.78588022888441,-1.93193255319577,-30.7646099781548));
#30315=CARTESIAN_POINT('Ctrl Pts',(2.82901226379223,-1.86750566617952,-30.760159203402));
#30316=CARTESIAN_POINT('Ctrl Pts',(2.84105706949321,-1.84913019440083,-30.7588879068001));
#30317=CARTESIAN_POINT('Ctrl Pts',(2.86264322671582,-1.81548969573245,-30.7565546544792));
#30318=CARTESIAN_POINT('Ctrl Pts',(2.87224336388092,-1.80026307194904,-30.7554963608487));
#30319=CARTESIAN_POINT('Ctrl Pts',(2.89241085282885,-1.76770375759864,-30.7532275169567));
#30320=CARTESIAN_POINT('Ctrl Pts',(2.9029443526255,-1.75035172354173,-30.7520151004813));
#30321=CARTESIAN_POINT('Ctrl Pts',(2.9325160771017,-1.70063644909779,-30.748534468944));
#30322=CARTESIAN_POINT('Ctrl Pts',(2.95117274399542,-1.66805097637427,-30.7462448436943));
#30323=CARTESIAN_POINT('Ctrl Pts',(3.03594077366381,-1.51412125799535,-30.7354139611759));
#30324=CARTESIAN_POINT('Ctrl Pts',(3.09512937938103,-1.38912485332063,-30.7265810616998));
#30325=CARTESIAN_POINT('Ctrl Pts',(3.24763652493694,-1.00854290486759,-30.7002075809962));
#30326=CARTESIAN_POINT('Ctrl Pts',(3.31804926228116,-0.744914686325395,
-30.6826943261426));
#30327=CARTESIAN_POINT('Ctrl Pts',(3.36337438075651,-0.425118351672462,
-30.6630892474786));
#30328=CARTESIAN_POINT('Ctrl Pts',(3.36939727275887,-0.374399891633058,
-30.6600235459955));
#30329=CARTESIAN_POINT('Ctrl Pts',(3.37743624900858,-0.29056542973385,-30.6550255082604));
#30330=CARTESIAN_POINT('Ctrl Pts',(3.38011626918766,-0.257522829622696,
-30.6530732210642));
#30331=CARTESIAN_POINT('Ctrl Pts',(3.38444456660954,-0.192296929617676,
-30.6492525912571));
#30332=CARTESIAN_POINT('Ctrl Pts',(3.3861194827012,-0.160118975755224,-30.6473836293678));
#30333=CARTESIAN_POINT('Ctrl Pts',(3.38907579492038,-0.0818362454576772,
-30.6428728641016));
#30334=CARTESIAN_POINT('Ctrl Pts',(3.38987556491014,-0.0357191256188062,
-30.6402459422375));
#30335=CARTESIAN_POINT('Ctrl Pts',(3.38930442140298,0.150408905845254,-30.629750063403));
#30336=CARTESIAN_POINT('Ctrl Pts',(3.3802012615131,0.290262323944762,-30.622113549099));
#30337=CARTESIAN_POINT('Ctrl Pts',(3.33566807784563,0.63917773754255,-30.6032417664708));
#30338=CARTESIAN_POINT('Ctrl Pts',(3.289248366481,0.8462076556394,-30.5922233648316));
#30339=CARTESIAN_POINT('Ctrl Pts',(3.19707720214389,1.12986473755841,-30.5760045100455));
#30340=CARTESIAN_POINT('Ctrl Pts',(3.16718736854465,1.21112298518536,-30.5712169438975));
#30341=CARTESIAN_POINT('Ctrl Pts',(3.12353346545864,1.317092038145,-30.564676904615));
#30342=CARTESIAN_POINT('Ctrl Pts',(3.11252184696708,1.3429074390276,-30.5630597173948));
#30343=CARTESIAN_POINT('Ctrl Pts',(3.09451938455987,1.38370080854579,-30.5604615088903));
#30344=CARTESIAN_POINT('Ctrl Pts',(3.08773709048788,1.3987700981898,-30.5594923380764));
#30345=CARTESIAN_POINT('Ctrl Pts',(3.07293157488553,1.43103340071639,-30.5573958955008));
#30346=CARTESIAN_POINT('Ctrl Pts',(3.06487369573038,1.4482107060445,-30.5562665474254));
#30347=CARTESIAN_POINT('Ctrl Pts',(3.04319024312234,1.49344263707125,-30.5532594900161));
#30348=CARTESIAN_POINT('Ctrl Pts',(3.02932124395607,1.52137780228847,-30.5513682562254));
#30349=CARTESIAN_POINT('Ctrl Pts',(2.94563728794847,1.68425317340055,-30.5401570101325));
#30350=CARTESIAN_POINT('Ctrl Pts',(2.86720422054698,1.81455772225659,-30.5304443542113));
#30351=CARTESIAN_POINT('Ctrl Pts',(2.62669602784828,2.15939238426101,-30.5033952975243));
#30352=CARTESIAN_POINT('Ctrl Pts',(2.44743232508606,2.36064138573899,-30.4861048516039));
#30353=CARTESIAN_POINT('Ctrl Pts',(2.20765789863874,2.57280197556173,-30.4666632546015));
#30354=CARTESIAN_POINT('Ctrl Pts',(2.16826854625577,2.60608429426852,-30.4635669205954));
#30355=CARTESIAN_POINT('Ctrl Pts',(2.10225677930828,2.65932824886272,-30.4585327183357));
#30356=CARTESIAN_POINT('Ctrl Pts',(2.07607369131353,2.67981873389785,-30.4565743160044));
#30357=CARTESIAN_POINT('Ctrl Pts',(2.02398217569842,2.71936299408918,-30.452751098815));
#30358=CARTESIAN_POINT('Ctrl Pts',(1.99809572754697,2.73843979449582,-30.4508855211496));
#30359=CARTESIAN_POINT('Ctrl Pts',(1.9347327171463,2.78375771747031,-30.4463989360582));
#30360=CARTESIAN_POINT('Ctrl Pts',(1.89698829102849,2.80961446114797,-30.4437924085016));
#30361=CARTESIAN_POINT('Ctrl Pts',(1.74519873107027,2.90914383004763,-30.4335530735329));
#30362=CARTESIAN_POINT('Ctrl Pts',(1.62729121329034,2.97670368884181,-30.4261373697569));
#30363=CARTESIAN_POINT('Ctrl Pts',(1.38411138919737,3.09726327145284,-30.4115570565399));
#30364=CARTESIAN_POINT('Ctrl Pts',(1.25907495134038,3.15016426924282,-30.4044048234716));
#30365=CARTESIAN_POINT('Ctrl Pts',(0.990894153168696,3.24510222204355,-30.3892677287199));
#30366=CARTESIAN_POINT('Ctrl Pts',(0.847475427105129,3.28547363548857,-30.3812851836906));
#30367=CARTESIAN_POINT('Ctrl Pts',(0.664923058647628,3.32411035450556,-30.3707706846519));
#30368=CARTESIAN_POINT('Ctrl Pts',(0.627836088364567,3.33131414360195,-30.3686163806658));
#30369=CARTESIAN_POINT('Ctrl Pts',(0.570385047073269,3.34148005983637,-30.3652405548998));
#30370=CARTESIAN_POINT('Ctrl Pts',(0.550100349700086,3.34487931781875,-30.3640412337996));
#30371=CARTESIAN_POINT('Ctrl Pts',(0.512088254238199,3.35089417237066,-30.3617778965681));
#30372=CARTESIAN_POINT('Ctrl Pts',(0.494369121350027,3.35355412229385,-30.3607162304572));
#30373=CARTESIAN_POINT('Ctrl Pts',(0.451304085638983,3.35967022682391,-30.3581207033446));
#30374=CARTESIAN_POINT('Ctrl Pts',(0.425938912102345,3.36298013188903,-30.3565793125276));
#30375=CARTESIAN_POINT('Ctrl Pts',(0.330901913095462,3.37428911865159,-30.3507629405616));
#30376=CARTESIAN_POINT('Ctrl Pts',(0.261028423953723,3.3804120985929,-30.3464042718121));
#30377=CARTESIAN_POINT('Ctrl Pts',(0.0660205524847508,3.39141874390945,
-30.3340979306516));
#30378=CARTESIAN_POINT('Ctrl Pts',(-0.0592694319147097,3.3915430929957,
-30.3260324125525));
#30379=CARTESIAN_POINT('Ctrl Pts',(-0.411268998308128,3.37237935504958,
-30.3033269244206));
#30380=CARTESIAN_POINT('Ctrl Pts',(-0.636476659751925,3.33721586636319,
-30.288789981977));
#30381=CARTESIAN_POINT('Ctrl Pts',(-0.910985651576816,3.26552942853779,
-30.2714942813932));
#30382=CARTESIAN_POINT('Ctrl Pts',(-0.965119870503428,3.24994176958631,
-30.2681014264206));
#30383=CARTESIAN_POINT('Ctrl Pts',(-1.0514536739844,3.22273475516236,-30.262717071615));
#30384=CARTESIAN_POINT('Ctrl Pts',(-1.08390781583331,3.21196483555598,-30.2606991069521));
#30385=CARTESIAN_POINT('Ctrl Pts',(-1.14611375329735,3.19027151872824,-30.2568414095638));
#30386=CARTESIAN_POINT('Ctrl Pts',(-1.17588607666498,3.17941836390154,-30.254999647956));
#30387=CARTESIAN_POINT('Ctrl Pts',(-1.24554624105348,3.15291219026105,-30.2506989419629));
#30388=CARTESIAN_POINT('Ctrl Pts',(-1.28529859029521,3.13691703502367,-30.2482514322087));
#30389=CARTESIAN_POINT('Ctrl Pts',(-1.42479366301469,3.07769130386727,-30.2396758498533));
#30390=CARTESIAN_POINT('Ctrl Pts',(-1.52275286718551,3.03042033681127,-30.2336800194438));
#30391=CARTESIAN_POINT('Ctrl Pts',(-1.77551187615951,2.8930923073103,-30.2180790358137));
#30392=CARTESIAN_POINT('Ctrl Pts',(-1.92573392557676,2.79534896820772,-30.2086805884349));
#30393=CARTESIAN_POINT('Ctrl Pts',(-2.17867119322614,2.60066597443253,-30.1916745069931));
#30394=CARTESIAN_POINT('Ctrl Pts',(-2.28437775215542,2.50832274690606,-30.184129774781));
#30395=CARTESIAN_POINT('Ctrl Pts',(-2.41065658131156,2.38338844450821,-30.174116233239));
#30396=CARTESIAN_POINT('Ctrl Pts',(-2.43682187083831,2.35662991597437,-30.1719814985218));
#30397=CARTESIAN_POINT('Ctrl Pts',(-2.47662025365248,2.3145576532787,-30.168629911429));
#30398=CARTESIAN_POINT('Ctrl Pts',(-2.490567177018,2.29954345505224,-30.1674347630228));
#30399=CARTESIAN_POINT('Ctrl Pts',(-2.51646534743088,2.27115146695888,-30.1651743722106));
#30400=CARTESIAN_POINT('Ctrl Pts',(-2.52844785787659,2.25780384554049,-30.1641113909861));
#30401=CARTESIAN_POINT('Ctrl Pts',(-2.55735685659966,2.22508265047021,-30.1615056083016));
#30402=CARTESIAN_POINT('Ctrl Pts',(-2.57416956818621,2.20561053675838,-30.1599551237235));
#30403=CARTESIAN_POINT('Ctrl Pts',(-2.63675296855501,2.13143752162013,-30.1540559373522));
#30404=CARTESIAN_POINT('Ctrl Pts',(-2.6810125056473,2.07549094726914,-30.1496205625073));
#30405=CARTESIAN_POINT('Ctrl Pts',(-2.8002212030882,1.91462364107994,-30.1369977695026));
#30406=CARTESIAN_POINT('Ctrl Pts',(-2.87099762910775,1.80676303771441,-30.1286862764339));
#30407=CARTESIAN_POINT('Ctrl Pts',(-3.04556133080121,1.50447259189867,-30.1062040789973));
#30408=CARTESIAN_POINT('Ctrl Pts',(-3.13684151164966,1.303507574418,-30.092139217259));
#30409=CARTESIAN_POINT('Ctrl Pts',(-3.2265181311771,1.04080522694941,-30.0752034532165));
#30410=CARTESIAN_POINT('Ctrl Pts',(-3.24366755888014,0.986060917945988,
-30.0717461698013));
#30411=CARTESIAN_POINT('Ctrl Pts',(-3.268865766985,0.897833295513708,-30.0662860419803));
#30412=CARTESIAN_POINT('Ctrl Pts',(-3.2778075980432,0.864618707316396,-30.0642553663751));
#30413=CARTESIAN_POINT('Ctrl Pts',(-3.29399433744646,0.800628221617553,
-30.0603890394647));
#30414=CARTESIAN_POINT('Ctrl Pts',(-3.30131721612446,0.76987595206582,-30.0585511056436));
#30415=CARTESIAN_POINT('Ctrl Pts',(-3.317438459156,0.697709997797373,-30.0542828012291));
#30416=CARTESIAN_POINT('Ctrl Pts',(-3.32589337531506,0.656224544131117,
-30.0518633469465));
#30417=CARTESIAN_POINT('Ctrl Pts',(-3.34624000959653,0.545863348588604,
-30.0455094883723));
#30418=CARTESIAN_POINT('Ctrl Pts',(-3.35678289001173,0.476758323617263,
-30.0416156751619));
#30419=CARTESIAN_POINT('Ctrl Pts',(-3.38166259622505,0.271235008702921,
-30.0302304108983));
#30420=CARTESIAN_POINT('Ctrl Pts',(-3.38986683334396,0.134219282446046,
-30.0228978926989));
#30421=CARTESIAN_POINT('Ctrl Pts',(-3.38974874325427,-0.00291892207943553,
-30.0156103845689));
#30422=CARTESIAN_POINT('',(-3.38974953533873,0.00177487207047444,-28.7660178032));
#30423=CARTESIAN_POINT('Ctrl Pts',(-3.38974872454211,-0.00294057224222385,
-30.0160178032104));
#30424=CARTESIAN_POINT('Ctrl Pts',(-3.38963484568422,-0.134214583385583,
-30.0083170754981));
#30425=CARTESIAN_POINT('Ctrl Pts',(-3.38189161080866,-0.265159729420946,
-30.0006163477858));
#30426=CARTESIAN_POINT('Ctrl Pts',(-3.36665492089121,-0.395018614927236,
-29.9929156200736));
#30427=CARTESIAN_POINT('Ctrl Pts',(-3.35111993381036,-0.527419820149826,
-29.9850641309266));
#30428=CARTESIAN_POINT('Ctrl Pts',(-3.32779521844705,-0.658692042817637,
-29.9772126417796));
#30429=CARTESIAN_POINT('Ctrl Pts',(-3.29687322499598,-0.788055836095793,
-29.9693611526326));
#30430=CARTESIAN_POINT('Ctrl Pts',(-3.29214449671142,-0.807838720703128,
-29.9681604681145));
#30431=CARTESIAN_POINT('Ctrl Pts',(-3.28723819018725,-0.827577014639484,
-29.9669597835964));
#30432=CARTESIAN_POINT('Ctrl Pts',(-3.28215509176372,-0.847267971842154,
-29.9657590990783));
#30433=CARTESIAN_POINT('Ctrl Pts',(-3.25631504677856,-0.947367394973932,
-29.9596553923673));
#30434=CARTESIAN_POINT('Ctrl Pts',(-3.22584825566311,-1.04645142692693,
-29.9535516856563));
#30435=CARTESIAN_POINT('Ctrl Pts',(-3.19085081991225,-1.14406123418518,
-29.9474479789452));
#30436=CARTESIAN_POINT('Ctrl Pts',(-3.15589918499894,-1.24154330034387,
-29.9413522601017));
#30437=CARTESIAN_POINT('Ctrl Pts',(-3.11642883628647,-1.33755457844917,
-29.9352565412582));
#30438=CARTESIAN_POINT('Ctrl Pts',(-3.07258634988741,-1.43164876453185,
-29.9291608224147));
#30439=CARTESIAN_POINT('Ctrl Pts',(-3.0287887209982,-1.52564667799801,-29.9230713404156));
#30440=CARTESIAN_POINT('Ctrl Pts',(-2.980628029503,-1.61773101454663,-29.9169818584165));
#30441=CARTESIAN_POINT('Ctrl Pts',(-2.9282995880987,-1.70747374352901,-29.9108923764175));
#30442=CARTESIAN_POINT('Ctrl Pts',(-2.87600805259324,-1.7971531792814,-29.9048071891728));
#30443=CARTESIAN_POINT('Ctrl Pts',(-2.81955482721702,-1.88449392346243,
-29.8987220019282));
#30444=CARTESIAN_POINT('Ctrl Pts',(-2.75918158501452,-1.96909167978963,
-29.8926368146836));
#30445=CARTESIAN_POINT('Ctrl Pts',(-2.69883044215406,-2.05365846950506,
-29.8865538548932));
#30446=CARTESIAN_POINT('Ctrl Pts',(-2.6345623823551,-2.13548391940741,-29.8804708951028));
#30447=CARTESIAN_POINT('Ctrl Pts',(-2.56666246662722,-2.21419259435738,
-29.8743879353125));
#30448=CARTESIAN_POINT('Ctrl Pts',(-2.49876984974142,-2.29289280858715,
-29.8683056294045));
#30449=CARTESIAN_POINT('Ctrl Pts',(-2.42724643247243,-2.36847659050669,
-29.8622233234966));
#30450=CARTESIAN_POINT('Ctrl Pts',(-2.3524170444764,-2.44060220260429,-29.8561410175886));
#30451=CARTESIAN_POINT('Ctrl Pts',(-2.27757635327864,-2.51273870949023,
-29.8500577929303));
#30452=CARTESIAN_POINT('Ctrl Pts',(-2.19942900695891,-2.58141571209807,
-29.8439745682719));
#30453=CARTESIAN_POINT('Ctrl Pts',(-2.11833543487584,-2.64632954256445,
-29.8378913436136));
#30454=CARTESIAN_POINT('Ctrl Pts',(-2.03715807415193,-2.71131044421154,
-29.8318018335603));
#30455=CARTESIAN_POINT('Ctrl Pts',(-1.95302874273048,-2.77252014120312,
-29.8257123235071));
#30456=CARTESIAN_POINT('Ctrl Pts',(-1.86633955206104,-2.82969640401804,
-29.8196228134538));
#30457=CARTESIAN_POINT('Ctrl Pts',(-1.77960360175262,-2.88690350737242,
-29.8135300187547));
#30458=CARTESIAN_POINT('Ctrl Pts',(-1.69030540905641,-2.9400726241836,-29.8074372240555));
#30459=CARTESIAN_POINT('Ctrl Pts',(-1.59886284357325,-2.98898689691689,
-29.8013444293564));
#30460=CARTESIAN_POINT('Ctrl Pts',(-1.507272722582,-3.03798009974503,-29.7952418030716));
#30461=CARTESIAN_POINT('Ctrl Pts',(-1.41353170251924,-3.08270455912023,
-29.7891391767867));
#30462=CARTESIAN_POINT('Ctrl Pts',(-1.31807902546371,-3.12299099344405,
-29.7830365505019));
#30463=CARTESIAN_POINT('Ctrl Pts',(-1.24585108273921,-3.15347527487726,
-29.7784187633914));
#30464=CARTESIAN_POINT('Ctrl Pts',(-1.17264352409538,-3.18141943340367,
-29.773800976281));
#30465=CARTESIAN_POINT('Ctrl Pts',(-1.09865184334181,-3.20676927601935,
-29.7691831891705));
#30466=CARTESIAN_POINT('Ctrl Pts',(-1.00084858134843,-3.24027706059163,
-29.7630793321152));
#30467=CARTESIAN_POINT('Ctrl Pts',(-0.9013471461894,-3.26936255109773,-29.75697547506));
#30468=CARTESIAN_POINT('Ctrl Pts',(-0.800583569394607,-3.29385351995431,
-29.7508716180047));
#30469=CARTESIAN_POINT('Ctrl Pts',(-0.699951809905278,-3.3183124501157,
-29.744775745918));
#30470=CARTESIAN_POINT('Ctrl Pts',(-0.59806160317771,-3.338188707894,-29.7386798738313));
#30471=CARTESIAN_POINT('Ctrl Pts',(-0.495366290736147,-3.35335910700037,
-29.7325840017446));
#30472=CARTESIAN_POINT('Ctrl Pts',(-0.392776003753793,-3.36851399149273,
-29.7264943638448));
#30473=CARTESIAN_POINT('Ctrl Pts',(-0.289382668966533,-3.37897252537377,
-29.7204047259449));
#30474=CARTESIAN_POINT('Ctrl Pts',(-0.185651185774396,-3.38466227262345,
-29.714315088045));
#30475=CARTESIAN_POINT('Ctrl Pts',(-0.081992803451167,-3.39034801023734,
-29.7082297415889));
#30476=CARTESIAN_POINT('Ctrl Pts',(0.0220028278789831,-3.3912716208874,
-29.7021443951327));
#30477=CARTESIAN_POINT('Ctrl Pts',(0.125865117903764,-3.387412439399,-29.6960590486766));
#30478=CARTESIAN_POINT('Ctrl Pts',(0.229689424208958,-3.38355466926083,
-29.6899759277066));
#30479=CARTESIAN_POINT('Ctrl Pts',(0.333380059500198,-3.37491759923433,
-29.6838928067367));
#30480=CARTESIAN_POINT('Ctrl Pts',(0.436466658870567,-3.36153267397394,
-29.6778096857667));
#30481=CARTESIAN_POINT('Ctrl Pts',(0.539542207175188,-3.3481491836012,-29.6717272169181));
#30482=CARTESIAN_POINT('Ctrl Pts',(0.642013424516179,-3.33001890519619,
-29.6656447480695));
#30483=CARTESIAN_POINT('Ctrl Pts',(0.743416201023518,-3.30722503234294,
-29.6595622792208));
#30484=CARTESIAN_POINT('Ctrl Pts',(0.844834320244893,-3.28442771067019,
-29.6534788900663));
#30485=CARTESIAN_POINT('Ctrl Pts',(0.945183260445176,-3.2569654863683,-29.6473955009117));
#30486=CARTESIAN_POINT('Ctrl Pts',(1.04401111103125,-3.22497222663131,-29.6413121117571));
#30487=CARTESIAN_POINT('Ctrl Pts',(1.14294109343841,-3.19294590404958,-29.6352224358361));
#30488=CARTESIAN_POINT('Ctrl Pts',(1.24034643965251,-3.15637932680083,-29.629132759915));
#30489=CARTESIAN_POINT('Ctrl Pts',(1.33579240652075,-3.11545561823331,-29.623043083994));
#30490=CARTESIAN_POINT('Ctrl Pts',(1.43128987071761,-3.07450982951157,-29.616950122423));
#30491=CARTESIAN_POINT('Ctrl Pts',(1.52482546507202,-3.02920241301288,-29.610857160852));
#30492=CARTESIAN_POINT('Ctrl Pts',(1.61598815786518,-2.97976296643533,-29.604764199281));
#30493=CARTESIAN_POINT('Ctrl Pts',(1.70729794924743,-2.93024374519762,-29.5986614062096));
#30494=CARTESIAN_POINT('Ctrl Pts',(1.79622682431919,-2.87657939595367,-29.5925586131381));
#30495=CARTESIAN_POINT('Ctrl Pts',(1.882391716187,-2.81904354158118,-29.5864558200667));
#30496=CARTESIAN_POINT('Ctrl Pts',(1.94756722992035,-2.77552316123222,-29.5818396397987));
#30497=CARTESIAN_POINT('Ctrl Pts',(2.01116192165579,-2.72978862040712,-29.5772234595306));
#30498=CARTESIAN_POINT('Ctrl Pts',(2.0730231287862,-2.6819731859244,-29.5726072792626));
#30499=CARTESIAN_POINT('Ctrl Pts',(2.1548036995478,-2.61876113907625,-29.5665046848489));
#30500=CARTESIAN_POINT('Ctrl Pts',(2.23382774027247,-2.55169894592992,-29.5604020904352));
#30501=CARTESIAN_POINT('Ctrl Pts',(2.30971157540194,-2.48105572306514,-29.5542994960215));
#30502=CARTESIAN_POINT('Ctrl Pts',(2.38549607407754,-2.41050497638105,-29.5482048902669));
#30503=CARTESIAN_POINT('Ctrl Pts',(2.4581482291904,-2.3363828085167,-29.5421102845122));
#30504=CARTESIAN_POINT('Ctrl Pts',(2.52731577703097,-2.25899978434491,-29.5360156787576));
#30505=CARTESIAN_POINT('Ctrl Pts',(2.59641255055622,-2.18169594081092,-29.5299273091869));
#30506=CARTESIAN_POINT('Ctrl Pts',(2.66203152358469,-2.10113819305185,-29.5238389396162));
#30507=CARTESIAN_POINT('Ctrl Pts',(2.72385643947098,-2.01767469123555,-29.5177505700455));
#30508=CARTESIAN_POINT('Ctrl Pts',(2.78563779983912,-1.93426998927392,-29.5116664897179));
#30509=CARTESIAN_POINT('Ctrl Pts',(2.84363016461202,-1.8479639466973,-29.5055824093902));
#30510=CARTESIAN_POINT('Ctrl Pts',(2.89755736718324,-1.75913796115658,-29.4994983290626));
#30511=CARTESIAN_POINT('Ctrl Pts',(2.95146485976785,-1.67034444084495,-29.4934164724205));
#30512=CARTESIAN_POINT('Ctrl Pts',(3.0013099214621,-1.57903317318219,-29.4873346157784));
#30513=CARTESIAN_POINT('Ctrl Pts',(3.04686001700828,-1.48561404787929,-29.4812527591363));
#30514=CARTESIAN_POINT('Ctrl Pts',(3.09240525321185,-1.3922048886485,-29.4751715513145));
#30515=CARTESIAN_POINT('Ctrl Pts',(3.13365624704176,-1.2966887032753,-29.4690903434927));
#30516=CARTESIAN_POINT('Ctrl Pts',(3.17042711307225,-1.19949863826367,-29.4630091356709));
#30517=CARTESIAN_POINT('Ctrl Pts',(3.20720357291047,-1.10229378810835,-29.4569270027388));
#30518=CARTESIAN_POINT('Ctrl Pts',(3.23949839956419,-1.00341495234551,-29.4508448698067));
#30519=CARTESIAN_POINT('Ctrl Pts',(3.26717473184124,-0.903312976834777,
-29.4447627368745));
#30520=CARTESIAN_POINT('Ctrl Pts',(3.29487974043413,-0.803107282527913,
-29.4386743020537));
#30521=CARTESIAN_POINT('Ctrl Pts',(3.31795658401251,-0.701676330474625,
-29.4325858672329));
#30522=CARTESIAN_POINT('Ctrl Pts',(3.33631897631765,-0.599483736862607,
-29.4264974324121));
#30523=CARTESIAN_POINT('Ctrl Pts',(3.3546912977617,-0.497235884412761,-29.4204057053779));
#30524=CARTESIAN_POINT('Ctrl Pts',(3.36834403386814,-0.394225993959921,
-29.4143139783436));
#30525=CARTESIAN_POINT('Ctrl Pts',(3.37724275221989,-0.290923452265745,
-29.4082222513093));
#30526=CARTESIAN_POINT('Ctrl Pts',(3.38615586636746,-0.187453794112863,
-29.4021206694561));
#30527=CARTESIAN_POINT('Ctrl Pts',(3.39029958255419,-0.0836909664586204,
-29.3960190876028));
#30528=CARTESIAN_POINT('Ctrl Pts',(3.38969161732259,0.01989477200076,-29.3899175057496));
#30529=CARTESIAN_POINT('Ctrl Pts',(3.38923040970286,0.0984757983311476,
-29.385288793618));
#30530=CARTESIAN_POINT('Ctrl Pts',(3.3860357536877,0.176954896702791,-29.3806600814864));
#30531=CARTESIAN_POINT('Ctrl Pts',(3.38013519819818,0.255129583548729,-29.3760313693548));
#30532=CARTESIAN_POINT('Ctrl Pts',(3.37235303818692,0.358233083371036,-29.369926625739));
#30533=CARTESIAN_POINT('Ctrl Pts',(3.35983614049466,0.461152792640079,-29.3638218821233));
#30534=CARTESIAN_POINT('Ctrl Pts',(3.34259823615956,0.563419997979316,-29.3577171385075));
#30535=CARTESIAN_POINT('Ctrl Pts',(3.32538289832877,0.665553323162041,-29.3516203867404));
#30536=CARTESIAN_POINT('Ctrl Pts',(3.30345891147442,0.767035424854807,-29.3455236349733));
#30537=CARTESIAN_POINT('Ctrl Pts',(3.27689189940138,0.867401027286458,-29.3394268832063));
#30538=CARTESIAN_POINT('Ctrl Pts',(3.2503520877535,0.967663871189969,-29.3333363735502));
#30539=CARTESIAN_POINT('Ctrl Pts',(3.21917881274537,1.06681207813027,-29.3272458638942));
#30540=CARTESIAN_POINT('Ctrl Pts',(3.1834888927682,1.16438976812815,-29.3211553542382));
#30541=CARTESIAN_POINT('Ctrl Pts',(3.14782421015841,1.26189845813911,-29.3150691513565));
#30542=CARTESIAN_POINT('Ctrl Pts',(3.10764938037095,1.35783843961796,-29.3089829484748));
#30543=CARTESIAN_POINT('Ctrl Pts',(3.06313104016448,1.45176902201448,-29.3028967455931));
#30544=CARTESIAN_POINT('Ctrl Pts',(3.01862904948541,1.54566510805234,-29.2968127778922));
#30545=CARTESIAN_POINT('Ctrl Pts',(2.96978690161386,1.63755287605232,-29.2907288101913));
#30546=CARTESIAN_POINT('Ctrl Pts',(2.91681903096719,1.7270123922797,-29.2846448424904));
#30547=CARTESIAN_POINT('Ctrl Pts',(2.86385693047201,1.81646216307168,-29.2785615375576));
#30548=CARTESIAN_POINT('Ctrl Pts',(2.80677021865848,1.90348384050798,-29.2724782326248));
#30549=CARTESIAN_POINT('Ctrl Pts',(2.74581841907227,1.98768364484479,-29.266394927692));
#30550=CARTESIAN_POINT('Ctrl Pts',(2.68485751476335,2.07189602659319,-29.2603107140608));
#30551=CARTESIAN_POINT('Ctrl Pts',(2.62003062617236,2.15328535166928,-29.2542265004296));
#30552=CARTESIAN_POINT('Ctrl Pts',(2.55163903494482,2.23148903153161,-29.2481422867984));
#30553=CARTESIAN_POINT('Ctrl Pts',(2.48317703270879,2.30977322421528,-29.2420518093033));
#30554=CARTESIAN_POINT('Ctrl Pts',(2.41114328059405,2.38486489977891,-29.2359613318082));
#30555=CARTESIAN_POINT('Ctrl Pts',(2.33587755638856,2.45643666803364,-29.2298708543132));
#30556=CARTESIAN_POINT('Ctrl Pts',(2.26057137087792,2.52804691179879,-29.2237771027026));
#30557=CARTESIAN_POINT('Ctrl Pts',(2.18203007520766,2.59613319908747,-29.2176833510921));
#30558=CARTESIAN_POINT('Ctrl Pts',(2.10062681002168,2.66040825203917,-29.2115895994816));
#30559=CARTESIAN_POINT('Ctrl Pts',(2.01909256895207,2.72478672199555,-29.2054860431722));
#30560=CARTESIAN_POINT('Ctrl Pts',(1.93468750697555,2.78534145861058,-29.1993824868629));
#30561=CARTESIAN_POINT('Ctrl Pts',(1.84781419885469,2.84182824058932,-29.1932789305535));
#30562=CARTESIAN_POINT('Ctrl Pts',(1.78222999385105,2.88447241714279,-29.1886711068513));
#30563=CARTESIAN_POINT('Ctrl Pts',(1.71523965533779,2.92479902033357,-29.1840632831491));
#30564=CARTESIAN_POINT('Ctrl Pts',(1.64702482028717,2.96272076035829,-29.179455459447));
#30565=CARTESIAN_POINT('Ctrl Pts',(1.55664606832032,3.01296378349692,-29.1733504918812));
#30566=CARTESIAN_POINT('Ctrl Pts',(1.4638153391217,3.05915135961099,-29.1672455243155));
#30567=CARTESIAN_POINT('Ctrl Pts',(1.3689316745371,3.10103710602583,-29.1611405567498));
#30568=CARTESIAN_POINT('Ctrl Pts',(1.27417189082164,3.14286816607613,-29.1550435598784));
#30569=CARTESIAN_POINT('Ctrl Pts',(1.17736488808481,3.180408391561,-29.148946563007));
#30570=CARTESIAN_POINT('Ctrl Pts',(1.07893537895798,3.21345662963308,-29.1428495661356));
#30571=CARTESIAN_POINT('Ctrl Pts',(0.980606310713293,3.24647114413776,-29.1367587908511));
#30572=CARTESIAN_POINT('Ctrl Pts',(0.880658431361001,3.27500265116174,-29.1306680155666));
#30573=CARTESIAN_POINT('Ctrl Pts',(0.779536764973355,3.29889792120867,-29.1245772402821));
#30574=CARTESIAN_POINT('Ctrl Pts',(0.678486113565275,3.32277641026123,-29.1184907423825));
#30575=CARTESIAN_POINT('Ctrl Pts',(0.576263728945264,3.34202503917259,-29.1124042444828));
#30576=CARTESIAN_POINT('Ctrl Pts',(0.473329354025469,3.35654053828013,-29.1063177465832));
#30577=CARTESIAN_POINT('Ctrl Pts',(0.370432478015325,3.37105074940306,-29.1002334659898));
#30578=CARTESIAN_POINT('Ctrl Pts',(0.2668245497823,3.38083119818105,-29.0941491853964));
#30579=CARTESIAN_POINT('Ctrl Pts',(0.162974268410279,3.38582995000283,-29.088064904803));
#30580=CARTESIAN_POINT('Ctrl Pts',(0.0591350030289799,3.39082817157853,
-29.0819812696039));
#30581=CARTESIAN_POINT('Ctrl Pts',(-0.0449461376778227,3.39104568435428,
-29.0758976344048));
#30582=CARTESIAN_POINT('Ctrl Pts',(-0.148797494856594,3.38648259526376,
-29.0698139992057));
#30583=CARTESIAN_POINT('Ctrl Pts',(-0.252664652339694,3.38191881192911,
-29.0637294384213));
#30584=CARTESIAN_POINT('Ctrl Pts',(-0.356301530027339,3.37257300040057,
-29.0576448776369));
#30585=CARTESIAN_POINT('Ctrl Pts',(-0.459239547455927,3.35849729798201,
-29.0515603168526));
#30586=CARTESIAN_POINT('Ctrl Pts',(-0.562283938322313,3.34440705010306,
-29.0454694684432));
#30587=CARTESIAN_POINT('Ctrl Pts',(-0.664627602662921,3.32557720835593,
-29.0393786200339));
#30588=CARTESIAN_POINT('Ctrl Pts',(-0.76581017663551,3.30211142087324,-29.0332877716245));
#30589=CARTESIAN_POINT('Ctrl Pts',(-0.867047368978681,3.27863296655449,
-29.0271936353742));
#30590=CARTESIAN_POINT('Ctrl Pts',(-0.967121811170322,3.25051369721142,
-29.0210994991238));
#30591=CARTESIAN_POINT('Ctrl Pts',(-1.06558828489369,3.21790718784699,-29.0150053628735));
#30592=CARTESIAN_POINT('Ctrl Pts',(-1.16421347436755,3.18524812083111,-29.0089014036309));
#30593=CARTESIAN_POINT('Ctrl Pts',(-1.26122511869676,3.14808751814462,-29.0027974443883));
#30594=CARTESIAN_POINT('Ctrl Pts',(-1.3561977631002,3.10662722093624,-28.9966934851457));
#30595=CARTESIAN_POINT('Ctrl Pts',(-1.42784229970525,3.07535080655755,-28.9920888399435));
#30596=CARTESIAN_POINT('Ctrl Pts',(-1.4983269104377,3.04162854815276,-28.9874841947413));
#30597=CARTESIAN_POINT('Ctrl Pts',(-1.567479148493,3.00556387081354,-28.9828795495391));
#30598=CARTESIAN_POINT('Ctrl Pts',(-1.65903176983785,2.95781681531374,-28.9767833283541));
#30599=CARTESIAN_POINT('Ctrl Pts',(-1.74855650684832,2.90580153269723,-28.9706871071691));
#30600=CARTESIAN_POINT('Ctrl Pts',(-1.83562875182568,2.84971439761441,-28.964590885984));
#30601=CARTESIAN_POINT('Ctrl Pts',(-1.92258668196672,2.79370089784063,-28.9585026683658));
#30602=CARTESIAN_POINT('Ctrl Pts',(-2.0070981636955,2.73362640301431,-28.9524144507476));
#30603=CARTESIAN_POINT('Ctrl Pts',(-2.0887621366013,2.66973365697794,-28.9463262331293));
#30604=CARTESIAN_POINT('Ctrl Pts',(-2.17034237264281,2.60590642548871,-28.940244258267));
#30605=CARTESIAN_POINT('Ctrl Pts',(-2.24908056991337,2.53826899052723,-28.9341622834047));
#30606=CARTESIAN_POINT('Ctrl Pts',(-2.32460443485265,2.46710747312787,-28.9280803085424));
#30607=CARTESIAN_POINT('Ctrl Pts',(-2.40007523589183,2.39599595459515,-28.9220026069427));
#30608=CARTESIAN_POINT('Ctrl Pts',(-2.47233588434936,2.32136557020203,-28.915924905343));
#30609=CARTESIAN_POINT('Ctrl Pts',(-2.54104764926716,2.24354226763256,-28.9098472037433));
#30610=CARTESIAN_POINT('Ctrl Pts',(-2.60973440863595,2.16574728647804,-28.9037717139376));
#30611=CARTESIAN_POINT('Ctrl Pts',(-2.6748745677829,2.08476201730779,-28.8976962241318));
#30612=CARTESIAN_POINT('Ctrl Pts',(-2.73616729782295,2.00094817044927,-28.891620734326));
#30613=CARTESIAN_POINT('Ctrl Pts',(-2.79745367670782,1.91714300838496,-28.8855458740627));
#30614=CARTESIAN_POINT('Ctrl Pts',(-2.85489316624182,1.83051019738962,-28.8794710137995));
#30615=CARTESIAN_POINT('Ctrl Pts',(-2.90822674487783,1.74144258098776,-28.8733961535362));
#30616=CARTESIAN_POINT('Ctrl Pts',(-2.96156867966017,1.6523610097369,-28.8673203414819));
#30617=CARTESIAN_POINT('Ctrl Pts',(-3.0108032052869,1.56084424291391,-28.8612445294276));
#30618=CARTESIAN_POINT('Ctrl Pts',(-3.05571643314041,1.46731119491935,-28.8551687173734));
#30619=CARTESIAN_POINT('Ctrl Pts',(-3.10067683507646,1.37367990558394,-28.8490865236611));
#30620=CARTESIAN_POINT('Ctrl Pts',(-3.14130668936545,1.27802849296878,-28.8430043299488));
#30621=CARTESIAN_POINT('Ctrl Pts',(-3.17743963820953,1.18079736112294,-28.8369221362365));
#30622=CARTESIAN_POINT('Ctrl Pts',(-3.21359235251758,1.08351304185413,-28.8308366154396));
#30623=CARTESIAN_POINT('Ctrl Pts',(-3.24524313126079,0.984647690411331,
-28.8247510946426));
#30624=CARTESIAN_POINT('Ctrl Pts',(-3.27227564826182,0.884656512038806,
-28.8186655738456));
#30625=CARTESIAN_POINT('Ctrl Pts',(-3.2993524765141,0.784501429793518,-28.8125700777644));
#30626=CARTESIAN_POINT('Ctrl Pts',(-3.32179582826501,0.683217252858073,
-28.8064745816832));
#30627=CARTESIAN_POINT('Ctrl Pts',(-3.33954056054869,0.581269220714567,
-28.800379085602));
#30628=CARTESIAN_POINT('Ctrl Pts',(-3.35319900700356,0.502797947327609,
-28.7956872702785));
#30629=CARTESIAN_POINT('Ctrl Pts',(-3.36407473000155,0.423933574638009,
-28.7909954549549));
#30630=CARTESIAN_POINT('Ctrl Pts',(-3.37215904810011,0.344888992019939,
-28.7863036396313));
#30631=CARTESIAN_POINT('Ctrl Pts',(-3.3838103417463,0.230968234326469,-28.7795416941708));
#30632=CARTESIAN_POINT('Ctrl Pts',(-3.38968948999923,0.116452751436606,
-28.7727797487102));
#30633=CARTESIAN_POINT('Ctrl Pts',(-3.38974953533829,0.00177487291182191,
-28.7660178032496));
#30634=CARTESIAN_POINT('',(2.57323442701465,2.20655152809232,-28.));
#30635=CARTESIAN_POINT('Ctrl Pts',(-3.38974953533873,0.00177487207047244,
-28.7660178032));
#30636=CARTESIAN_POINT('Ctrl Pts',(-3.38980310654502,-0.100538401451488,
-28.75998493283));
#30637=CARTESIAN_POINT('Ctrl Pts',(-3.38522025555718,-0.203029763549593,
-28.75395206246));
#30638=CARTESIAN_POINT('Ctrl Pts',(-3.37597896934322,-0.305239350432197,
-28.7479191920901));
#30639=CARTESIAN_POINT('Ctrl Pts',(-3.36674870944206,-0.407326985148261,
-28.7418935198865));
#30640=CARTESIAN_POINT('Ctrl Pts',(-3.35287109906797,-0.509133079755363,
-28.7358678476829));
#30641=CARTESIAN_POINT('Ctrl Pts',(-3.33437615323607,-0.610197288776856,
-28.7298421754793));
#30642=CARTESIAN_POINT('Ctrl Pts',(-3.31589815767161,-0.711168874365579,
-28.7238220256901));
#30643=CARTESIAN_POINT('Ctrl Pts',(-3.29281131851551,-0.811399497129672,
-28.717801875901));
#30644=CARTESIAN_POINT('Ctrl Pts',(-3.26519740258242,-0.91043450322856,
-28.7117817261118));
#30645=CARTESIAN_POINT('Ctrl Pts',(-3.2375970288672,-1.00942094129262,-28.7057645286811));
#30646=CARTESIAN_POINT('Ctrl Pts',(-3.20547410556064,-1.1072125061738,-28.6997473312505));
#30647=CARTESIAN_POINT('Ctrl Pts',(-3.16896118880233,-1.20336613146812,
-28.6937301338198));
#30648=CARTESIAN_POINT('Ctrl Pts',(-3.13245620321812,-1.29949887069771,
-28.6877142434182));
#30649=CARTESIAN_POINT('Ctrl Pts',(-3.09156327463266,-1.39399396796392,
-28.6816983530165));
#30650=CARTESIAN_POINT('Ctrl Pts',(-3.04646403832871,-1.48642588973348,
-28.6756824626148));
#30651=CARTESIAN_POINT('Ctrl Pts',(-3.00136227726844,-1.57886298604915,
-28.6696662354301));
#30652=CARTESIAN_POINT('Ctrl Pts',(-2.95205393406501,-1.66923628426913,
-28.6636500082454));
#30653=CARTESIAN_POINT('Ctrl Pts',(-2.89876730066561,-1.75714347709337,
-28.6576337810607));
#30654=CARTESIAN_POINT('Ctrl Pts',(-2.84543109922401,-1.84513244253425,
-28.6516119574894));
#30655=CARTESIAN_POINT('Ctrl Pts',(-2.78810944516356,-1.93065034629345,
-28.6455901339181));
#30656=CARTESIAN_POINT('Ctrl Pts',(-2.72707469177338,-2.01332279776223,
-28.6395683103468));
#30657=CARTESIAN_POINT('Ctrl Pts',(-2.66601051922395,-2.09603509790542,
-28.6335435842162));
#30658=CARTESIAN_POINT('Ctrl Pts',(-2.60122996006742,-2.17589887487336,
-28.6275188580857));
#30659=CARTESIAN_POINT('Ctrl Pts',(-2.53304517815146,-2.25257345894504,
-28.6214941319551));
#30660=CARTESIAN_POINT('Ctrl Pts',(-2.46475386927682,-2.32936783382664,
-28.6154599932293));
#30661=CARTESIAN_POINT('Ctrl Pts',(-2.39304802168692,-2.40296275122096,
-28.6094258545036));
#30662=CARTESIAN_POINT('Ctrl Pts',(-2.31827612471118,-2.47305496746314,
-28.6033917157778));
#30663=CARTESIAN_POINT('Ctrl Pts',(-2.26183713073789,-2.52596166543485,
-28.5988370537597));
#30664=CARTESIAN_POINT('Ctrl Pts',(-2.20365202008319,-2.57687349208777,
-28.5942823917416));
#30665=CARTESIAN_POINT('Ctrl Pts',(-2.14388196705614,-2.62567613650875,
-28.5897277297235));
#30666=CARTESIAN_POINT('Ctrl Pts',(-2.06370305261451,-2.6911427515339,-28.5836178496453));
#30667=CARTESIAN_POINT('Ctrl Pts',(-1.98039165559376,-2.75304047990566,
-28.5775079695672));
#30668=CARTESIAN_POINT('Ctrl Pts',(-1.89429830396667,-2.81105656259155,
-28.571398089489));
#30669=CARTESIAN_POINT('Ctrl Pts',(-1.8083158140953,-2.86899793840791,-28.5652960770571));
#30670=CARTESIAN_POINT('Ctrl Pts',(-1.71955884270337,-2.92306737006823,
-28.5591940646251));
#30671=CARTESIAN_POINT('Ctrl Pts',(-1.62841107528683,-2.97299216823442,
-28.5530920521932));
#30672=CARTESIAN_POINT('Ctrl Pts',(-1.53735482696757,-3.02286683821218,
-28.5469961666329));
#30673=CARTESIAN_POINT('Ctrl Pts',(-1.44391292853432,-3.0686049468868,-28.5409002810726));
#30674=CARTESIAN_POINT('Ctrl Pts',(-1.34849742419764,-3.10997745320321,
-28.5348043955122));
#30675=CARTESIAN_POINT('Ctrl Pts',(-1.2531470092126,-3.15132173654233,-28.5287126683667));
#30676=CARTESIAN_POINT('Ctrl Pts',(-1.1558260557273,-3.18830617072937,-28.5226209412211));
#30677=CARTESIAN_POINT('Ctrl Pts',(-1.05696983234893,-3.2207483347825,-28.5165292140755));
#30678=CARTESIAN_POINT('Ctrl Pts',(-0.95814844390792,-3.25317906687199,
-28.5104396335316));
#30679=CARTESIAN_POINT('Ctrl Pts',(-0.857793265508878,-3.28107057744885,
-28.5043500529876));
#30680=CARTESIAN_POINT('Ctrl Pts',(-0.756357358928734,-3.30428942559431,
-28.4982604724437));
#30681=CARTESIAN_POINT('Ctrl Pts',(-0.654931144185521,-3.32750605526213,
-28.4921714737374));
#30682=CARTESIAN_POINT('Ctrl Pts',(-0.552424822165616,-3.3460508153024,
-28.486082475031));
#30683=CARTESIAN_POINT('Ctrl Pts',(-0.449303478872774,-3.35984098528083,
-28.4799934763247));
#30684=CARTESIAN_POINT('Ctrl Pts',(-0.346165504000262,-3.37363337936052,
-28.4739034955746));
#30685=CARTESIAN_POINT('Ctrl Pts',(-0.242412733307144,-3.38266960316241,
-28.4678135148245));
#30686=CARTESIAN_POINT('Ctrl Pts',(-0.138516342137413,-3.38691870074569,
-28.4617235340745));
#30687=CARTESIAN_POINT('Ctrl Pts',(-0.0345117887296656,-3.39117222188882,
-28.4556272132972));
#30688=CARTESIAN_POINT('Ctrl Pts',(0.0696362570227238,-3.39062864685194,
-28.4495308925199));
#30689=CARTESIAN_POINT('Ctrl Pts',(0.173455666763486,-3.38530917261151,
-28.4434345717426));
#30690=CARTESIAN_POINT('Ctrl Pts',(0.277331697530255,-3.37998679723642,
-28.4373349261541));
#30691=CARTESIAN_POINT('Ctrl Pts',(0.380878310944875,-3.36988337545165,
-28.4312352805656));
#30692=CARTESIAN_POINT('Ctrl Pts',(0.48362951546565,-3.35507191491784,-28.4251356349771));
#30693=CARTESIAN_POINT('Ctrl Pts',(0.586546240260744,-3.34023659483881,
-28.419026163567));
#30694=CARTESIAN_POINT('Ctrl Pts',(0.688664577673534,-3.32067816601063,
-28.4129166921568));
#30695=CARTESIAN_POINT('Ctrl Pts',(0.789529504308436,-3.29652062398015,
-28.4068072207467));
#30696=CARTESIAN_POINT('Ctrl Pts',(0.864677904805932,-3.27852228992977,
-28.4022554204363));
#30697=CARTESIAN_POINT('Ctrl Pts',(0.939130799015132,-3.25797212364141,
-28.397703620126));
#30698=CARTESIAN_POINT('Ctrl Pts',(1.01270679071419,-3.23493895128507,-28.3931518198157));
#30699=CARTESIAN_POINT('Ctrl Pts',(1.11040033392321,-3.20435571119722,-28.3871079801062));
#30700=CARTESIAN_POINT('Ctrl Pts',(1.20688947698545,-3.16928585797825,-28.3810641403967));
#30701=CARTESIAN_POINT('Ctrl Pts',(1.30172715649947,-3.12984208428026,-28.3750203006872));
#30702=CARTESIAN_POINT('Ctrl Pts',(1.39643905301889,-3.09045062476793,-28.3689844769083));
#30703=CARTESIAN_POINT('Ctrl Pts',(1.48950343902635,-3.04669693812566,-28.3629486531294));
#30704=CARTESIAN_POINT('Ctrl Pts',(1.58048776448782,-2.99874365173222,-28.3569128293505));
#30705=CARTESIAN_POINT('Ctrl Pts',(1.67137870739474,-2.95083958261175,-28.3508832004919));
#30706=CARTESIAN_POINT('Ctrl Pts',(1.76019344897887,-2.89874468315972,-28.3448535716333));
#30707=CARTESIAN_POINT('Ctrl Pts',(1.84651973715302,-2.84266950643305,-28.3388239427747));
#30708=CARTESIAN_POINT('Ctrl Pts',(1.93278872440559,-2.78663155080522,-28.3327983162113));
#30709=CARTESIAN_POINT('Ctrl Pts',(2.01657217530537,-2.7266188048023,-28.3267726896479));
#30710=CARTESIAN_POINT('Ctrl Pts',(2.09748356663111,-2.66288710804879,-28.3207470630846));
#30711=CARTESIAN_POINT('Ctrl Pts',(2.17836758470594,-2.59917697245864,-28.3147234750597));
#30712=CARTESIAN_POINT('Ctrl Pts',(2.25638113037952,-2.53175065501087,-28.3086998870348));
#30713=CARTESIAN_POINT('Ctrl Pts',(2.33116853732715,-2.4609059943598,-28.3026762990099));
#30714=CARTESIAN_POINT('Ctrl Pts',(2.40595093707213,-2.39006607693472,-28.2966531142793));
#30715=CARTESIAN_POINT('Ctrl Pts',(2.47750731023465,-2.3158085714327,-28.2906299295486));
#30716=CARTESIAN_POINT('Ctrl Pts',(2.54551760259735,-2.2384693871856,-28.2846067448179));
#30717=CARTESIAN_POINT('Ctrl Pts',(2.61354179761439,-2.16111439327339,-28.2785823288286));
#30718=CARTESIAN_POINT('Ctrl Pts',(2.67801818359024,-2.08067679727522,-28.2725579128393));
#30719=CARTESIAN_POINT('Ctrl Pts',(2.73866656138667,-1.99752610196776,-28.2665334968501));
#30720=CARTESIAN_POINT('Ctrl Pts',(2.79938665850301,-1.91427707738036,-28.2605019567293));
#30721=CARTESIAN_POINT('Ctrl Pts',(2.85626945081757,-1.8283089007561,-28.2544704166086));
#30722=CARTESIAN_POINT('Ctrl Pts',(2.90907777540975,-1.74002056284317,-28.2484388764879));
#30723=CARTESIAN_POINT('Ctrl Pts',(2.96191806166619,-1.65167878937371,-28.242403685843));
#30724=CARTESIAN_POINT('Ctrl Pts',(3.01067876566425,-1.56101444423797,-28.2363684951982));
#30725=CARTESIAN_POINT('Ctrl Pts',(3.05516949359125,-1.46844966816347,-28.2303333045534));
#30726=CARTESIAN_POINT('Ctrl Pts',(3.09974159863611,-1.37571558367249,-28.2242870750598));
#30727=CARTESIAN_POINT('Ctrl Pts',(3.14002795762882,-1.28107452736866,-28.2182408455661));
#30728=CARTESIAN_POINT('Ctrl Pts',(3.175886884025,-1.18496732544741,-28.2121946160724));
#30729=CARTESIAN_POINT('Ctrl Pts',(3.20676398053332,-1.10221216105455,-28.2069883806842));
#30730=CARTESIAN_POINT('Ctrl Pts',(3.23435916229513,-1.01837035387577,-28.201782145296));
#30731=CARTESIAN_POINT('Ctrl Pts',(3.25861234957539,-0.933729413531954,
-28.1965759099078));
#30732=CARTESIAN_POINT('Ctrl Pts',(3.28780567586033,-0.83184793461674,-28.190309214869));
#30733=CARTESIAN_POINT('Ctrl Pts',(3.31225712048596,-0.728455522703703,
-28.1840425198302));
#30734=CARTESIAN_POINT('Ctrl Pts',(3.33181715661598,-0.624018827744321,
-28.1777758247914));
#30735=CARTESIAN_POINT('Ctrl Pts',(3.35134888363776,-0.519733283308555,
-28.171518199498));
#30736=CARTESIAN_POINT('Ctrl Pts',(3.36600321919982,-0.414406853895198,
-28.1652605742047));
#30737=CARTESIAN_POINT('Ctrl Pts',(3.37568072894995,-0.308520143095911,
-28.1590029489113));
#30738=CARTESIAN_POINT('Ctrl Pts',(3.38534642513137,-0.202762690749069,
-28.1527529624515));
#30739=CARTESIAN_POINT('Ctrl Pts',(3.39004735322447,-0.0964467143875391,
-28.1465029759917));
#30740=CARTESIAN_POINT('Ctrl Pts',(3.38973542977069,0.00993874525860727,
-28.1402529895319));
#30741=CARTESIAN_POINT('Ctrl Pts',(3.38942386891304,0.116200536886331,-28.134010268383));
#30742=CARTESIAN_POINT('Ctrl Pts',(3.38411106704277,0.222531252864325,-28.1277675472341));
#30743=CARTESIAN_POINT('Ctrl Pts',(3.37380092760016,0.328439284228145,-28.1215248260852));
#30744=CARTESIAN_POINT('Ctrl Pts',(3.36349780134744,0.434275274555289,-28.1152863513764));
#30745=CARTESIAN_POINT('Ctrl Pts',(3.34820414192129,0.539688756021538,-28.1090478766675));
#30746=CARTESIAN_POINT('Ctrl Pts',(3.32797584730017,0.644190827540035,-28.1028094019586));
#30747=CARTESIAN_POINT('Ctrl Pts',(3.30775716445643,0.748643243332921,-28.0965738915545));
#30748=CARTESIAN_POINT('Ctrl Pts',(3.28260859040427,0.852184719762061,-28.0903383811504));
#30749=CARTESIAN_POINT('Ctrl Pts',(3.25263743906703,0.954334717213748,-28.0841028707463));
#30750=CARTESIAN_POINT('Ctrl Pts',(3.2226743873289,1.05645710898496,-28.0778690454672));
#30751=CARTESIAN_POINT('Ctrl Pts',(3.18789146676026,1.15718838780062,-28.071635220188));
#30752=CARTESIAN_POINT('Ctrl Pts',(3.14844620259218,1.25606192995524,-28.0654013949088));
#30753=CARTESIAN_POINT('Ctrl Pts',(3.10899302898307,1.35495529792337,-28.0591663196425));
#30754=CARTESIAN_POINT('Ctrl Pts',(3.0648757872674,1.45198981188523,-28.0529312443762));
#30755=CARTESIAN_POINT('Ctrl Pts',(3.01630056916356,1.54671779551526,-28.0466961691099));
#30756=CARTESIAN_POINT('Ctrl Pts',(2.96772117818811,1.64145391678686,-28.0404605582172));
#30757=CARTESIAN_POINT('Ctrl Pts',(2.91468323604366,1.73388276038755,-28.0342249473245));
#30758=CARTESIAN_POINT('Ctrl Pts',(2.85743883369826,1.82358119483974,-28.0279893364318));
#30759=CARTESIAN_POINT('Ctrl Pts',(2.80015690628584,1.91333842874876,-28.0217496379478));
#30760=CARTESIAN_POINT('Ctrl Pts',(2.73866323120876,2.00036134475808,-28.0155099394639));
#30761=CARTESIAN_POINT('Ctrl Pts',(2.67325324860397,2.08425577397025,-28.00927024098));
#30762=CARTESIAN_POINT('Ctrl Pts',(2.64086032113565,2.12580273748017,-28.0061801606533));
#30763=CARTESIAN_POINT('Ctrl Pts',(2.60750755147691,2.16658292429367,-28.0030900803267));
#30764=CARTESIAN_POINT('Ctrl Pts',(2.57323442701465,2.20655152809233,-28.));
#30765=CARTESIAN_POINT('',(-2.57363857939818,2.20608012663486,-28.0000033383279));
#30766=CARTESIAN_POINT('Origin',(0.,0.,-28.));
#30767=CARTESIAN_POINT('',(-3.38974897692414,0.00263361762172135,-29.1089821967504));
#30768=CARTESIAN_POINT('Ctrl Pts',(-2.57363857939818,2.20608012663486,-28.0000033383279));
#30769=CARTESIAN_POINT('Ctrl Pts',(-2.50673445663565,2.28413124970314,-28.0060715002323));
#30770=CARTESIAN_POINT('Ctrl Pts',(-2.43615914058954,2.35927292180629,-28.0121396621368));
#30771=CARTESIAN_POINT('Ctrl Pts',(-2.36219674153845,2.43113792631457,-28.0182078240412));
#30772=CARTESIAN_POINT('Ctrl Pts',(-2.28833018792174,2.50290980333291,-28.0242681224147));
#30773=CARTESIAN_POINT('Ctrl Pts',(-2.21108558311393,2.57141315314271,-28.0303284207882));
#30774=CARTESIAN_POINT('Ctrl Pts',(-2.13078697233906,2.63631408239044,-28.0363887191617));
#30775=CARTESIAN_POINT('Ctrl Pts',(-2.04690586672721,2.70411054422213,-28.0427193956579));
#30776=CARTESIAN_POINT('Ctrl Pts',(-1.95969221025354,2.76797529752797,-28.049050072154));
#30777=CARTESIAN_POINT('Ctrl Pts',(-1.86955832191721,2.82757082023601,-28.0553807486502));
#30778=CARTESIAN_POINT('Ctrl Pts',(-1.78341967391273,2.88452473455106,-28.0614308139963));
#30779=CARTESIAN_POINT('Ctrl Pts',(-1.69461455007407,2.9375795375758,-28.0674808793424));
#30780=CARTESIAN_POINT('Ctrl Pts',(-1.60353534230482,2.98648279226239,-28.0735309446885));
#30781=CARTESIAN_POINT('Ctrl Pts',(-1.51248509611952,3.03537049657529,-28.0795790862203));
#30782=CARTESIAN_POINT('Ctrl Pts',(-1.41916258411661,3.0801090712017,-28.0856272277522));
#30783=CARTESIAN_POINT('Ctrl Pts',(-1.32398618142917,3.12049125201219,-28.0916753692841));
#30784=CARTESIAN_POINT('Ctrl Pts',(-1.22881467326578,3.16087135613613,-28.0977231997853));
#30785=CARTESIAN_POINT('Ctrl Pts',(-1.13178986282324,3.19689534332487,-28.1037710302866));
#30786=CARTESIAN_POINT('Ctrl Pts',(-1.03335064130715,3.22840386485491,-28.1098188607879));
#30787=CARTESIAN_POINT('Ctrl Pts',(-0.934890242212077,3.25991916492497,
-28.1158679923804));
#30788=CARTESIAN_POINT('Ctrl Pts',(-0.83501524001308,3.28691693803133,-28.1219171239729));
#30789=CARTESIAN_POINT('Ctrl Pts',(-0.734179284391769,3.30928781475259,
-28.1279662555654));
#30790=CARTESIAN_POINT('Ctrl Pts',(-0.633238313295393,3.33168198959438,
-28.1340216870181));
#30791=CARTESIAN_POINT('Ctrl Pts',(-0.531334814649758,3.34943955747195,
-28.1400771184709));
#30792=CARTESIAN_POINT('Ctrl Pts',(-0.428932011686522,3.36250240027432,
-28.1461325499236));
#30793=CARTESIAN_POINT('Ctrl Pts',(-0.326466514805168,3.37557324052181,
-28.1521916886843));
#30794=CARTESIAN_POINT('Ctrl Pts',(-0.223501535989294,3.38394359936853,
-28.158250827445));
#30795=CARTESIAN_POINT('Ctrl Pts',(-0.120502826735627,3.38760743464303,
-28.1643099662056));
#30796=CARTESIAN_POINT('Ctrl Pts',(-0.0173532184998645,3.39127663764512,
-28.1703779819501));
#30797=CARTESIAN_POINT('Ctrl Pts',(0.0858297871031276,3.39022556151545,
-28.1764459976945));
#30798=CARTESIAN_POINT('Ctrl Pts',(0.188583218928551,3.38450017462528,-28.182514013439));
#30799=CARTESIAN_POINT('Ctrl Pts',(0.221383298329125,3.38267256515997,-28.1844509939825));
#30800=CARTESIAN_POINT('Ctrl Pts',(0.254139669302539,3.380369055138,-28.186387974526));
#30801=CARTESIAN_POINT('Ctrl Pts',(0.286837486178399,3.37759223693785,-28.1883249550694));
#30802=CARTESIAN_POINT('Ctrl Pts',(0.390033927538939,3.36882841770038,-28.1944381919204));
#30803=CARTESIAN_POINT('Ctrl Pts',(0.492994991660657,3.35531667111484,-28.2005514287714));
#30804=CARTESIAN_POINT('Ctrl Pts',(0.595250891976339,3.33707678037251,-28.2066646656224));
#30805=CARTESIAN_POINT('Ctrl Pts',(0.697376283909894,3.31886016905586,-28.2127701001984));
#30806=CARTESIAN_POINT('Ctrl Pts',(0.798797885574264,3.29592748602308,-28.2188755347744));
#30807=CARTESIAN_POINT('Ctrl Pts',(0.899050041752592,3.26835036140936,-28.2249809693504));
#30808=CARTESIAN_POINT('Ctrl Pts',(0.999202596477312,3.24080063492652,-28.2310803381202));
#30809=CARTESIAN_POINT('Ctrl Pts',(1.0981876078073,3.20861575589782,-28.2371797068899));
#30810=CARTESIAN_POINT('Ctrl Pts',(1.19554948127657,3.17191842586144,-28.2432790756596));
#30811=CARTESIAN_POINT('Ctrl Pts',(1.29284624534107,3.1352456366564,-28.2493743655609));
#30812=CARTESIAN_POINT('Ctrl Pts',(1.38852163272792,3.09406654720112,-28.2554696554622));
#30813=CARTESIAN_POINT('Ctrl Pts',(1.4821358524182,3.04855348935796,-28.2615649453636));
#30814=CARTESIAN_POINT('Ctrl Pts',(1.57571783758205,3.00305610319236,-28.2676581364514));
#30815=CARTESIAN_POINT('Ctrl Pts',(1.66723968318424,2.95322790092455,-28.2737513275393));
#30816=CARTESIAN_POINT('Ctrl Pts',(1.75628294273086,2.89928875546618,-28.2798445186272));
#30817=CARTESIAN_POINT('Ctrl Pts',(1.8453183444163,2.84535437001233,-28.2859371720051));
#30818=CARTESIAN_POINT('Ctrl Pts',(1.93187523087929,2.78730998353031,-28.292029825383));
#30819=CARTESIAN_POINT('Ctrl Pts',(2.01556184633548,2.72542024394344,-28.2981224787608));
#30820=CARTESIAN_POINT('Ctrl Pts',(2.0992625071243,2.66352011724778,-28.3042161546839));
#30821=CARTESIAN_POINT('Ctrl Pts',(2.18009159727073,2.59777360818453,-28.3103098306069));
#30822=CARTESIAN_POINT('Ctrl Pts',(2.25768903275896,2.52848675967661,-28.31640350653));
#30823=CARTESIAN_POINT('Ctrl Pts',(2.33536774186066,2.4591273418562,-28.3225035648168));
#30824=CARTESIAN_POINT('Ctrl Pts',(2.40980771871058,2.38622046367609,-28.3286036231036));
#30825=CARTESIAN_POINT('Ctrl Pts',(2.48068450226313,2.31011027068656,-28.3347036813904));
#30826=CARTESIAN_POINT('Ctrl Pts',(2.5516002534467,2.23395823276884,-28.3408070934527));
#30827=CARTESIAN_POINT('Ctrl Pts',(2.6189486333138,2.15459969637648,-28.3469105055151));
#30828=CARTESIAN_POINT('Ctrl Pts',(2.68244565252103,2.07241173123756,-28.3530139175774));
#30829=CARTESIAN_POINT('Ctrl Pts',(2.74604501148576,1.99009130166916,-28.3591271666639));
#30830=CARTESIAN_POINT('Ctrl Pts',(2.80578036520327,1.90493268242848,-28.3652404157503));
#30831=CARTESIAN_POINT('Ctrl Pts',(2.86141108945429,1.8173419159993,-28.3713536648368));
#30832=CARTESIAN_POINT('Ctrl Pts',(2.90250437960307,1.75264038950135,-28.3758693982169));
#30833=CARTESIAN_POINT('Ctrl Pts',(2.94135890813768,1.68661236036022,-28.380385131597));
#30834=CARTESIAN_POINT('Ctrl Pts',(2.97789427619774,1.61942914086685,-28.3849008649772));
#30835=CARTESIAN_POINT('Ctrl Pts',(3.0272200738309,1.52872618466213,-28.3909974821102));
#30836=CARTESIAN_POINT('Ctrl Pts',(3.07248261068612,1.4356120533336,-28.3970940992431));
#30837=CARTESIAN_POINT('Ctrl Pts',(3.1134388129218,1.34048641197592,-28.4031907163761));
#30838=CARTESIAN_POINT('Ctrl Pts',(3.15434073453724,1.24548684380211,-28.4092792534591));
#30839=CARTESIAN_POINT('Ctrl Pts',(3.19094749939381,1.14848145556161,-28.4153677905421));
#30840=CARTESIAN_POINT('Ctrl Pts',(3.22306142240295,1.04989529474032,-28.4214563276251));
#30841=CARTESIAN_POINT('Ctrl Pts',(3.25514201628678,0.951411450615359,-28.4275385457787));
#30842=CARTESIAN_POINT('Ctrl Pts',(3.28273890800558,0.851350501379768,-28.4336207639322));
#30843=CARTESIAN_POINT('Ctrl Pts',(3.30570246866219,0.750157484252925,-28.4397029820857));
#30844=CARTESIAN_POINT('Ctrl Pts',(3.32864946020359,0.649037481881261,-28.4457808116788));
#30845=CARTESIAN_POINT('Ctrl Pts',(3.34696967410669,0.546787452627108,-28.4518586412719));
#30846=CARTESIAN_POINT('Ctrl Pts',(3.36056354374999,0.443866794115685,-28.4579364708651));
#30847=CARTESIAN_POINT('Ctrl Pts',(3.37415230825051,0.340984787192796,-28.4640120179449));
#30848=CARTESIAN_POINT('Ctrl Pts',(3.38301819993575,0.237433075937281,-28.4700875650247));
#30849=CARTESIAN_POINT('Ctrl Pts',(3.38711305058994,0.133679635783901,-28.4761631121046));
#30850=CARTESIAN_POINT('Ctrl Pts',(3.39120742930755,0.029938153342284,-28.4822379589701));
#30851=CARTESIAN_POINT('Ctrl Pts',(3.39053184347868,-0.0740045835416433,
-28.4883128058357));
#30852=CARTESIAN_POINT('Ctrl Pts',(3.385090187282,-0.177678041600797,-28.4943876527012));
#30853=CARTESIAN_POINT('Ctrl Pts',(3.37964774181468,-0.281366536702726,
-28.5004633806769));
#30854=CARTESIAN_POINT('Ctrl Pts',(3.36943787517377,-0.384785247373206,
-28.5065391086526));
#30855=CARTESIAN_POINT('Ctrl Pts',(3.35451648540345,-0.487467139052987,
-28.5126148366283));
#30856=CARTESIAN_POINT('Ctrl Pts',(3.33957969096815,-0.590255038293975,
-28.5186968371131));
#30857=CARTESIAN_POINT('Ctrl Pts',(3.31992172138404,-0.692304174517732,
-28.5247788375979));
#30858=CARTESIAN_POINT('Ctrl Pts',(3.29564991575129,-0.793156160732879,
-28.5308608380827));
#30859=CARTESIAN_POINT('Ctrl Pts',(3.27136507514973,-0.894062308657929,
-28.5369461048547));
#30860=CARTESIAN_POINT('Ctrl Pts',(3.24246158248668,-0.993769614335579,
-28.5430313716267));
#30861=CARTESIAN_POINT('Ctrl Pts',(3.20909657001154,-1.09183527459054,-28.5491166383986));
#30862=CARTESIAN_POINT('Ctrl Pts',(3.17567739682191,-1.19006012274419,-28.5552117832546));
#30863=CARTESIAN_POINT('Ctrl Pts',(3.13778239326417,-1.28663760299493,-28.5613069281106));
#30864=CARTESIAN_POINT('Ctrl Pts',(3.09561678262821,-1.38114510374927,-28.5674020729665));
#30865=CARTESIAN_POINT('Ctrl Pts',(3.06316098297479,-1.45388960961474,-28.5720936402727));
#30866=CARTESIAN_POINT('Ctrl Pts',(3.02817595905214,-1.52540811904442,-28.5767852075789));
#30867=CARTESIAN_POINT('Ctrl Pts',(2.99077316820085,-1.59551901238119,-28.581476774885));
#30868=CARTESIAN_POINT('Ctrl Pts',(2.94210189656725,-1.68675248069739,-28.5875817884829));
#30869=CARTESIAN_POINT('Ctrl Pts',(2.88917087800472,-1.77590930521859,-28.5936868020808));
#30870=CARTESIAN_POINT('Ctrl Pts',(2.83218164326374,-1.8625660262283,-28.5997918156787));
#30871=CARTESIAN_POINT('Ctrl Pts',(2.77526691130241,-1.94910945976154,-28.6058888481116));
#30872=CARTESIAN_POINT('Ctrl Pts',(2.71430474357666,-2.03315893378495,-28.6119858805445));
#30873=CARTESIAN_POINT('Ctrl Pts',(2.64954277448203,-2.11431505426463,-28.6180829129774));
#30874=CARTESIAN_POINT('Ctrl Pts',(2.5848470010219,-2.19538822203358,-28.6241737134051));
#30875=CARTESIAN_POINT('Ctrl Pts',(2.51635941472635,-2.2735735851106,-28.6302645138328));
#30876=CARTESIAN_POINT('Ctrl Pts',(2.4443707131458,-2.34850098556826,-28.6363553142605));
#30877=CARTESIAN_POINT('Ctrl Pts',(2.37243275292753,-2.4233755733166,-28.6424418215769));
#30878=CARTESIAN_POINT('Ctrl Pts',(2.29699888006311,-2.49499645796672,-28.6485283288932));
#30879=CARTESIAN_POINT('Ctrl Pts',(2.21839926144782,-2.5630274636273,-28.6546148362095));
#30880=CARTESIAN_POINT('Ctrl Pts',(2.13982840118596,-2.63103357782224,-28.6606991165694));
#30881=CARTESIAN_POINT('Ctrl Pts',(2.05809441998022,-2.69545214433512,-28.6667833969293));
#30882=CARTESIAN_POINT('Ctrl Pts',(1.97356286039723,-2.75598525006225,-28.6728676772892));
#30883=CARTESIAN_POINT('Ctrl Pts',(1.88904040141231,-2.81651183884509,-28.6789513026205));
#30884=CARTESIAN_POINT('Ctrl Pts',(1.80172131031927,-2.87315354999893,-28.6850349279518));
#30885=CARTESIAN_POINT('Ctrl Pts',(1.7120018516603,-2.92565458016009,-28.691118553283));
#30886=CARTESIAN_POINT('Ctrl Pts',(1.62226888471389,-2.97816351494993,-28.6972030945735));
#30887=CARTESIAN_POINT('Ctrl Pts',(1.53013520090068,-3.02653031436172,-28.7032876358639));
#30888=CARTESIAN_POINT('Ctrl Pts',(1.43602270857422,-3.07054455153465,-28.7093721771543));
#30889=CARTESIAN_POINT('Ctrl Pts',(1.34181319140568,-3.11460416498342,-28.7154629912747));
#30890=CARTESIAN_POINT('Ctrl Pts',(1.24562117938076,-3.15430207369077,-28.721553805395));
#30891=CARTESIAN_POINT('Ctrl Pts',(1.14788962550167,-3.18947557917687,-28.7276446195154));
#30892=CARTESIAN_POINT('Ctrl Pts',(1.05010544842518,-3.22466802370823,-28.7337387132123));
#30893=CARTESIAN_POINT('Ctrl Pts',(0.95078048645369,-3.25533108624429,-28.7398328069092));
#30894=CARTESIAN_POINT('Ctrl Pts',(0.85037205886202,-3.28135222492295,-28.7459269006062));
#30895=CARTESIAN_POINT('Ctrl Pts',(0.749801999855192,-3.30741525085718,
-28.7520308042066));
#30896=CARTESIAN_POINT('Ctrl Pts',(0.648145409439338,-3.3288213380325,-28.7581347078071));
#30897=CARTESIAN_POINT('Ctrl Pts',(0.545869191877263,-3.34550921204221,
-28.7642386114075));
#30898=CARTESIAN_POINT('Ctrl Pts',(0.46871358417293,-3.35809828789193,-28.768843302536));
#30899=CARTESIAN_POINT('Ctrl Pts',(0.391205542683911,-3.36800331474502,
-28.7734479936644));
#30900=CARTESIAN_POINT('Ctrl Pts',(0.313546054131859,-3.37521761290118,
-28.7780526847929));
#30901=CARTESIAN_POINT('Ctrl Pts',(0.210589936480036,-3.38478188049539,
-28.7841572977695));
#30902=CARTESIAN_POINT('Ctrl Pts',(0.107023913160425,-3.3896470357455,-28.7902619107461));
#30903=CARTESIAN_POINT('Ctrl Pts',(0.00331242799393805,-3.38974838156474,
-28.7963665237228));
#30904=CARTESIAN_POINT('Ctrl Pts',(-0.100263724207063,-3.38984959513797,
-28.8024631707988));
#30905=CARTESIAN_POINT('Ctrl Pts',(-0.203984537165262,-3.38519935749678,
-28.8085598178749));
#30906=CARTESIAN_POINT('Ctrl Pts',(-0.307380297863563,-3.37578471099466,
-28.814656464951));
#30907=CARTESIAN_POINT('Ctrl Pts',(-0.410670634049429,-3.36637966386596,
-28.8207468957563));
#30908=CARTESIAN_POINT('Ctrl Pts',(-0.513636153762811,-3.35221990668589,
-28.8268373265616));
#30909=CARTESIAN_POINT('Ctrl Pts',(-0.615807865942744,-3.33334452685933,
-28.8329277573669));
#30910=CARTESIAN_POINT('Ctrl Pts',(-0.717907984141793,-3.31448237342933,
-28.8390139204724));
#30911=CARTESIAN_POINT('Ctrl Pts',(-0.819214982005358,-3.29091124581986,
-28.845100083578));
#30912=CARTESIAN_POINT('Ctrl Pts',(-0.919266529428289,-3.26272188676462,
-28.8511862466836));
#30913=CARTESIAN_POINT('Ctrl Pts',(-1.01928172655826,-3.23454276934468,
-28.8572701985909));
#30914=CARTESIAN_POINT('Ctrl Pts',(-1.11804196899672,-3.20174887103431,
-28.8633541504982));
#30915=CARTESIAN_POINT('Ctrl Pts',(-1.21509741758321,-3.1644815259822,-28.8694381024054));
#30916=CARTESIAN_POINT('Ctrl Pts',(-1.31214267549895,-3.1272180939432,-28.8755214155073));
#30917=CARTESIAN_POINT('Ctrl Pts',(-1.40748309668015,-3.0854823023973,-28.8816047286091));
#30918=CARTESIAN_POINT('Ctrl Pts',(-1.50068710632903,-3.03946430664974,
-28.8876880417109));
#30919=CARTESIAN_POINT('Ctrl Pts',(-1.59390540550658,-2.99343925567493,
-28.893772287473));
#30920=CARTESIAN_POINT('Ctrl Pts',(-1.68498625925461,-2.94313088526703,
-28.8998565332351));
#30921=CARTESIAN_POINT('Ctrl Pts',(-1.77352187946848,-2.88877572780349,
-28.9059407789971));
#30922=CARTESIAN_POINT('Ctrl Pts',(-1.86214918643835,-2.83436428058847,
-28.9120313255538));
#30923=CARTESIAN_POINT('Ctrl Pts',(-1.94822563128211,-2.77589790111196,
-28.9181218721105));
#30924=CARTESIAN_POINT('Ctrl Pts',(-2.03137170533589,-2.71365695275965,
-28.9242124186671));
#30925=CARTESIAN_POINT('Ctrl Pts',(-2.11456275778207,-2.65138233477434,
-28.9303062599433));
#30926=CARTESIAN_POINT('Ctrl Pts',(-2.1948199518761,-2.58532935213631,-28.9364001012195));
#30927=CARTESIAN_POINT('Ctrl Pts',(-2.27179776314108,-2.51581795563335,
-28.9424939424957));
#30928=CARTESIAN_POINT('Ctrl Pts',(-2.34889984238038,-2.4461943444507,-28.9485976212731));
#30929=CARTESIAN_POINT('Ctrl Pts',(-2.42271165960536,-2.37310146742926,
-28.9547013000505));
#30930=CARTESIAN_POINT('Ctrl Pts',(-2.49292523092322,-2.29689548206409,
-28.9608049788279));
#30931=CARTESIAN_POINT('Ctrl Pts',(-2.54593181238301,-2.23936502612564,
-28.9654128507855));
#30932=CARTESIAN_POINT('Ctrl Pts',(-2.59688844964165,-2.18006108216403,
-28.9700207227431));
#30933=CARTESIAN_POINT('Ctrl Pts',(-2.64567876781292,-2.11914815905918,
-28.9746285947007));
#30934=CARTESIAN_POINT('Ctrl Pts',(-2.71006976820936,-2.03875835627035,
-28.9807098316381));
#30935=CARTESIAN_POINT('Ctrl Pts',(-2.77090798108598,-1.95528801259203,
-28.9867910685754));
#30936=CARTESIAN_POINT('Ctrl Pts',(-2.82788370594505,-1.86908501897331,
-28.9928723055128));
#30937=CARTESIAN_POINT('Ctrl Pts',(-2.8847877197454,-1.78299052257781,-28.9989458884547));
#30938=CARTESIAN_POINT('Ctrl Pts',(-2.93783866950888,-1.69417056537816,
-29.0050194713966));
#30939=CARTESIAN_POINT('Ctrl Pts',(-2.98676680436591,-1.60300627535822,
-29.0110930543385));
#30940=CARTESIAN_POINT('Ctrl Pts',(-3.03564623865997,-1.51193272560992,
-29.0171605919466));
#30941=CARTESIAN_POINT('Ctrl Pts',(-3.08041081135924,-1.41851985753198,
-29.0232281295547));
#30942=CARTESIAN_POINT('Ctrl Pts',(-3.12083437687428,-1.32317718186935,
-29.0292956671628));
#30943=CARTESIAN_POINT('Ctrl Pts',(-3.16122834708118,-1.2279043094472,-29.0353587625441));
#30944=CARTESIAN_POINT('Ctrl Pts',(-3.19728746135202,-1.13070483348132,
-29.0414218579254));
#30945=CARTESIAN_POINT('Ctrl Pts',(-3.22883222812558,-1.03201138807553,
-29.0474849533067));
#30946=CARTESIAN_POINT('Ctrl Pts',(-3.2603656937663,-0.933353300285324,
-29.0535458765417));
#30947=CARTESIAN_POINT('Ctrl Pts',(-3.28738789269004,-0.833202715478359,
-29.0596067997768));
#30948=CARTESIAN_POINT('Ctrl Pts',(-3.30976834383676,-0.732009953918703,
-29.0656677230119));
#30949=CARTESIAN_POINT('Ctrl Pts',(-3.33214418542468,-0.630838034386813,
-29.0717273979172));
#30950=CARTESIAN_POINT('Ctrl Pts',(-3.34988009184918,-0.528624786183428,
-29.0777870728226));
#30951=CARTESIAN_POINT('Ctrl Pts',(-3.36289636616285,-0.425832235685285,
-29.0838467477279));
#30952=CARTESIAN_POINT('Ctrl Pts',(-3.37591654326618,-0.323008863947966,
-29.0899082395615));
#30953=CARTESIAN_POINT('Ctrl Pts',(-3.38421421094914,-0.21960627064758,
-29.0959697313952));
#30954=CARTESIAN_POINT('Ctrl Pts',(-3.38776144183851,-0.116092530734182,
-29.1020312232288));
#30955=CARTESIAN_POINT('Ctrl Pts',(-3.38911736260653,-0.0765246440921415,
-29.1043482144027));
#30956=CARTESIAN_POINT('Ctrl Pts',(-3.38977972350901,-0.0369405421840939,
-29.1066652055765));
#30957=CARTESIAN_POINT('Ctrl Pts',(-3.38974897692414,0.00263361762172143,
-29.1089821967504));
#30958=CARTESIAN_POINT('',(-3.39460607963399,-0.000821927281527217,-30.3588436183143));
#30959=CARTESIAN_POINT('Ctrl Pts',(-3.38720500183428,0.00265191974547864,
-29.1089833849163));
#30960=CARTESIAN_POINT('Ctrl Pts',(-3.38984895601398,0.356633419419809,
-29.1297237581471));
#30961=CARTESIAN_POINT('Ctrl Pts',(-3.17696557429075,1.82585356689937,-29.2159894346803));
#30962=CARTESIAN_POINT('Ctrl Pts',(-1.06501084932491,3.84917142339401,-29.3677804145163));
#30963=CARTESIAN_POINT('Ctrl Pts',(2.62793364271971,3.00741003307344,-29.5643563244242));
#30964=CARTESIAN_POINT('Ctrl Pts',(3.95722561382568,-0.539375665666434,
-29.760932234332));
#30965=CARTESIAN_POINT('Ctrl Pts',(1.72720904884221,-3.6010077302552,-29.9575081442399));
#30966=CARTESIAN_POINT('Ctrl Pts',(-2.05632687273503,-3.42374860859984,
-30.1540840541477));
#30967=CARTESIAN_POINT('Ctrl Pts',(-3.37294674464125,-1.2066374231571,-30.2879087383179));
#30968=CARTESIAN_POINT('Ctrl Pts',(-3.39500475544003,-0.0479003925669444,
-30.3562081191854));
#30969=CARTESIAN_POINT('Ctrl Pts',(-3.39484736595381,-0.000830500879896085,
-30.3589821967504));
#30970=CARTESIAN_POINT('',(-3.38974868975108,0.00294214148269599,-32.8590963092955));
#30971=CARTESIAN_POINT('Ctrl Pts',(-3.38974993779964,-0.000649374565975133,
-30.3560545810355));
#30972=CARTESIAN_POINT('Ctrl Pts',(-3.38975358586039,0.0183935851200709,
-30.3572180084951));
#30973=CARTESIAN_POINT('Ctrl Pts',(-3.38959676423955,0.0374358997996179,
-30.3583882915823));
#30974=CARTESIAN_POINT('Ctrl Pts',(-3.38462768886899,0.335646200792595,
-30.3768133563173));
#30975=CARTESIAN_POINT('Ctrl Pts',(-3.34550345502142,0.613167531655111,
-30.3951989018399));
#30976=CARTESIAN_POINT('Ctrl Pts',(-3.2368976225608,1.01582230935899,-30.4216545317372));
#30977=CARTESIAN_POINT('Ctrl Pts',(-3.19291972730513,1.146591548526,-30.4302298245411));
#30978=CARTESIAN_POINT('Ctrl Pts',(-3.12382888221506,1.3168932102243,-30.4413320949894));
#30979=CARTESIAN_POINT('Ctrl Pts',(-3.10569832986211,1.35909999813467,-30.4440788642434));
#30980=CARTESIAN_POINT('Ctrl Pts',(-3.0734127628179,1.43023600271374,-30.4487022476129));
#30981=CARTESIAN_POINT('Ctrl Pts',(-3.05969352188649,1.4593548890198,-30.4505930464342));
#30982=CARTESIAN_POINT('Ctrl Pts',(-3.03098586910261,1.51810137848072,-30.4544057042695));
#30983=CARTESIAN_POINT('Ctrl Pts',(-3.01597274606492,1.54771303606426,-30.4563264647083));
#30984=CARTESIAN_POINT('Ctrl Pts',(-2.97665228767898,1.62252254202551,-30.4611793210982));
#30985=CARTESIAN_POINT('Ctrl Pts',(-2.95174878348213,1.66739849703661,-30.4640906333652));
#30986=CARTESIAN_POINT('Ctrl Pts',(-2.78939052236961,1.94492102040908,-30.4821331493347));
#30987=CARTESIAN_POINT('Ctrl Pts',(-2.62555401588435,2.16099346467813,-30.4962539515895));
#30988=CARTESIAN_POINT('Ctrl Pts',(-2.33298752888244,2.46380283459002,-30.5186929928453));
#30989=CARTESIAN_POINT('Ctrl Pts',(-2.22107088977081,2.56514913547031,-30.5268171500487));
#30990=CARTESIAN_POINT('Ctrl Pts',(-2.07835396388052,2.67802552438949,-30.5371561463535));
#30991=CARTESIAN_POINT('Ctrl Pts',(-2.05365093403885,2.69701568481328,-30.538945216027));
#30992=CARTESIAN_POINT('Ctrl Pts',(-2.01349493299563,2.72701356530531,-30.5418588296425));
#30993=CARTESIAN_POINT('Ctrl Pts',(-1.99820466793537,2.738237188038,-30.5429694810873));
#30994=CARTESIAN_POINT('Ctrl Pts',(-1.96941452280078,2.75900067700612,-30.5450646591374));
#30995=CARTESIAN_POINT('Ctrl Pts',(-1.95593743238517,2.76857129763282,-30.5460470446206));
#30996=CARTESIAN_POINT('Ctrl Pts',(-1.91937028056145,2.79413883664745,-30.5487156445718));
#30997=CARTESIAN_POINT('Ctrl Pts',(-1.89615093553784,2.80994762051065,-30.5504134536519));
#30998=CARTESIAN_POINT('Ctrl Pts',(-1.80036158778415,2.87343748353246,-30.5574223402428));
#30999=CARTESIAN_POINT('Ctrl Pts',(-1.72617317817206,2.9186073214435,-30.5628609836103));
#31000=CARTESIAN_POINT('Ctrl Pts',(-1.46565050443106,3.0638179648495,-30.581796064727));
#31001=CARTESIAN_POINT('Ctrl Pts',(-1.27173459714899,3.14925519353807,-30.5955804791992));
#31002=CARTESIAN_POINT('Ctrl Pts',(-0.938337451312478,3.26029350107068,
-30.6178862033972));
#31003=CARTESIAN_POINT('Ctrl Pts',(-0.802936044667959,3.29625428266166,
-30.6265990125933));
#31004=CARTESIAN_POINT('Ctrl Pts',(-0.620469483723358,3.33279899196888,
-30.637842705927));
#31005=CARTESIAN_POINT('Ctrl Pts',(-0.575072468011883,3.34093152726245,
-30.6406008571791));
#31006=CARTESIAN_POINT('Ctrl Pts',(-0.497698837645476,3.35316849685697,
-30.6452375052567));
#31007=CARTESIAN_POINT('Ctrl Pts',(-0.465804848341566,3.35774761570437,
-30.6471303836792));
#31008=CARTESIAN_POINT('Ctrl Pts',(-0.40097205263779,3.36611428938134,-30.6509425186538));
#31009=CARTESIAN_POINT('Ctrl Pts',(-0.368033252906537,3.36987472073429,
-30.6528607471546));
#31010=CARTESIAN_POINT('Ctrl Pts',(-0.284220177121389,3.37819958997654,
-30.6576976179));
#31011=CARTESIAN_POINT('Ctrl Pts',(-0.233287316671325,3.38209860725056,
-30.6605957628569));
#31012=CARTESIAN_POINT('Ctrl Pts',(0.0891574235648245,3.39946320171763,
-30.6787199088143));
#31013=CARTESIAN_POINT('Ctrl Pts',(0.361364906557596,3.381378977075,-30.6929200469411));
#31014=CARTESIAN_POINT('Ctrl Pts',(0.764319050930901,3.30534781892006,-30.7147773763137));
#31015=CARTESIAN_POINT('Ctrl Pts',(0.898429361952221,3.27144092983636,-30.7222198250094));
#31016=CARTESIAN_POINT('Ctrl Pts',(1.06585770564544,3.21803705276973,-30.7321297064945));
#31017=CARTESIAN_POINT('Ctrl Pts',(1.10143906864696,3.20603288459186,-30.7342725361819));
#31018=CARTESIAN_POINT('Ctrl Pts',(1.15593638274237,3.18663274114377,-30.7376219526686));
#31019=CARTESIAN_POINT('Ctrl Pts',(1.17499858567686,3.17965335004513,-30.7388063847505));
#31020=CARTESIAN_POINT('Ctrl Pts',(1.21084365028319,3.1661627799261,-30.7410599935874));
#31021=CARTESIAN_POINT('Ctrl Pts',(1.22763912509836,3.15968846819308,-30.7421271463286));
#31022=CARTESIAN_POINT('Ctrl Pts',(1.26481807522904,3.14501557903992,-30.744513497048));
#31023=CARTESIAN_POINT('Ctrl Pts',(1.28517494309795,3.1367519931313,-30.7458362356472));
#31024=CARTESIAN_POINT('Ctrl Pts',(1.35672408599625,3.10689422763244,-30.7505388243012));
#31025=CARTESIAN_POINT('Ctrl Pts',(1.40746202492807,3.08424089864925,-30.7539708610622));
#31026=CARTESIAN_POINT('Ctrl Pts',(1.70128762465155,2.94429450830231,-30.7743295317852));
#31027=CARTESIAN_POINT('Ctrl Pts',(1.93022654619818,2.79955124171538,-30.7920683964197));
#31028=CARTESIAN_POINT('Ctrl Pts',(2.23628508126793,2.55048585564335,-30.8169926153582));
#31029=CARTESIAN_POINT('Ctrl Pts',(2.32857919049858,2.4665104081326,-30.8247187570141));
#31030=CARTESIAN_POINT('Ctrl Pts',(2.44737772359241,2.34579258475137,-30.8349372444732));
#31031=CARTESIAN_POINT('Ctrl Pts',(2.47807946608571,2.31333590653276,-30.8376059556947));
#31032=CARTESIAN_POINT('Ctrl Pts',(2.52963885632384,2.2566245769547,-30.8421385967796));
#31033=CARTESIAN_POINT('Ctrl Pts',(2.55081065844471,2.23266484569021,-30.8440153797736));
#31034=CARTESIAN_POINT('Ctrl Pts',(2.59349955623754,2.18295460770493,-30.8478335258827));
#31035=CARTESIAN_POINT('Ctrl Pts',(2.61497966247934,2.15717691641315,-30.8497732830369));
#31036=CARTESIAN_POINT('Ctrl Pts',(2.66946478974455,2.08978077420758,-30.8547455137727));
#31037=CARTESIAN_POINT('Ctrl Pts',(2.70188131644235,2.04769717653687,-30.8577550206317));
#31038=CARTESIAN_POINT('Ctrl Pts',(2.88563712258405,1.79717730281712,-30.8751621516245));
#31039=CARTESIAN_POINT('Ctrl Pts',(3.0138089091122,1.57280440756817,-30.8886641721784));
#31040=CARTESIAN_POINT('Ctrl Pts',(3.17317778296728,1.20120034184514,-30.9101828213359));
#31041=CARTESIAN_POINT('Ctrl Pts',(3.22219382509087,1.0627317264624,-30.9180571031675));
#31042=CARTESIAN_POINT('Ctrl Pts',(3.27254393858055,0.884501223844759,-30.9284902939929));
#31043=CARTESIAN_POINT('Ctrl Pts',(3.28237481676887,0.847290710213697,-30.9306847139773));
#31044=CARTESIAN_POINT('Ctrl Pts',(3.29646496063004,0.790027594424019,-30.934097537345));
#31045=CARTESIAN_POINT('Ctrl Pts',(3.3011797000572,0.770089201540251,-30.9352924482041));
#31046=CARTESIAN_POINT('Ctrl Pts',(3.30968325137306,0.732614286937175,-30.9375527490426));
#31047=CARTESIAN_POINT('Ctrl Pts',(3.31351403276588,0.715088537662129,-30.9386158838828));
#31048=CARTESIAN_POINT('Ctrl Pts',(3.32166593970426,0.676321162212311,-30.9409801464701));
#31049=CARTESIAN_POINT('Ctrl Pts',(3.32592275572679,0.655066942645862,-30.9422845680587));
#31050=CARTESIAN_POINT('Ctrl Pts',(3.34001226484938,0.581037841138695,-30.9468529935358));
#31051=CARTESIAN_POINT('Ctrl Pts',(3.34879448592506,0.528073613371486,-30.9501655784687));
#31052=CARTESIAN_POINT('Ctrl Pts',(3.38452860039689,0.275539848205004,-30.9661010284483));
#31053=CARTESIAN_POINT('Ctrl Pts',(3.39491817418889,0.0740432031104546,
-30.9792051319548));
#31054=CARTESIAN_POINT('Ctrl Pts',(3.38163810647879,-0.279671140503619,
-31.0019063365813));
#31055=CARTESIAN_POINT('Ctrl Pts',(3.36562139752001,-0.431617184740064,
-31.011564881812));
#31056=CARTESIAN_POINT('Ctrl Pts',(3.32793447347453,-0.647865681019166,
-31.0250482061445));
#31057=CARTESIAN_POINT('Ctrl Pts',(3.31450435326363,-0.713400046439247,
-31.0291007808305));
#31058=CARTESIAN_POINT('Ctrl Pts',(3.290816242993,-0.813786298513853,-31.0352586647297));
#31059=CARTESIAN_POINT('Ctrl Pts',(3.28192333621835,-0.848939957908778,
-31.0374055805387));
#31060=CARTESIAN_POINT('Ctrl Pts',(3.26431562386488,-0.914125753838241,
-31.0413705777434));
#31061=CARTESIAN_POINT('Ctrl Pts',(3.25574607288868,-0.944192772074268,
-31.0431930101717));
#31062=CARTESIAN_POINT('Ctrl Pts',(3.23554107049048,-1.01153522880078,-31.0472622047982));
#31063=CARTESIAN_POINT('Ctrl Pts',(3.22367494195662,-1.04873713834653,-31.0495013597448));
#31064=CARTESIAN_POINT('Ctrl Pts',(3.18473935515363,-1.16389384009055,-31.0564119852642));
#31065=CARTESIAN_POINT('Ctrl Pts',(3.15546384164881,-1.24107333208645,-31.0610131287288));
#31066=CARTESIAN_POINT('Ctrl Pts',(3.02033272395213,-1.561523262308,-31.0801133717575));
#31067=CARTESIAN_POINT('Ctrl Pts',(2.88894199897272,-1.79297903821589,-31.0938220249885));
#31068=CARTESIAN_POINT('Ctrl Pts',(2.66873258781607,-2.09276426137196,-31.1138838507305));
#31069=CARTESIAN_POINT('Ctrl Pts',(2.60152728493106,-2.17574074135049,-31.1197370653941));
#31070=CARTESIAN_POINT('Ctrl Pts',(2.51118570885472,-2.27710263487643,-31.1274739734095));
#31071=CARTESIAN_POINT('Ctrl Pts',(2.49156666228204,-2.29855291897373,-31.129146974005));
#31072=CARTESIAN_POINT('Ctrl Pts',(2.45899196872442,-2.33326102979367,-31.1319183014254));
#31073=CARTESIAN_POINT('Ctrl Pts',(2.44619864511566,-2.34667013097372,-31.133005133312));
#31074=CARTESIAN_POINT('Ctrl Pts',(2.42155200053846,-2.37208252938787,-31.13509748181));
#31075=CARTESIAN_POINT('Ctrl Pts',(2.40971787143615,-2.38410347319309,-31.1361014268424));
#31076=CARTESIAN_POINT('Ctrl Pts',(2.37661642666656,-2.41722922550645,-31.1389063488815));
#31077=CARTESIAN_POINT('Ctrl Pts',(2.35515876809471,-2.43814064632731,-31.1407209612995));
#31078=CARTESIAN_POINT('Ctrl Pts',(2.25366893908093,-2.53445698889195,-31.1492748622876));
#31079=CARTESIAN_POINT('Ctrl Pts',(2.17028077094357,-2.60621819292162,-31.1562192221584));
#31080=CARTESIAN_POINT('Ctrl Pts',(1.91336028027547,-2.80642414761847,-31.1770409533759));
#31081=CARTESIAN_POINT('Ctrl Pts',(1.73086873725762,-2.9225106954594,-31.1910779954124));
#31082=CARTESIAN_POINT('Ctrl Pts',(1.43637285272958,-3.07252245211751,-31.2118770165785));
#31083=CARTESIAN_POINT('Ctrl Pts',(1.33158442983635,-3.11936668329667,-31.2189621857435));
#31084=CARTESIAN_POINT('Ctrl Pts',(1.18398532194336,-3.17655193541285,-31.2285011635569));
#31085=CARTESIAN_POINT('Ctrl Pts',(1.1430565847263,-3.19150831877507,-31.2311016341303));
#31086=CARTESIAN_POINT('Ctrl Pts',(1.07178142141577,-3.21600692490374,-31.2355555292295));
#31087=CARTESIAN_POINT('Ctrl Pts',(1.04156880579328,-3.22591854841439,-31.237420664576));
#31088=CARTESIAN_POINT('Ctrl Pts',(0.978849006700675,-3.24552152358349,
-31.2412472727363));
#31089=CARTESIAN_POINT('Ctrl Pts',(0.946326761894156,-3.25515300986888,
-31.2432066539072));
#31090=CARTESIAN_POINT('Ctrl Pts',(0.860754032928103,-3.27910451233216,
-31.2483007943268));
#31091=CARTESIAN_POINT('Ctrl Pts',(0.807489367090337,-3.29262589731823,
-31.2514102832812));
#31092=CARTESIAN_POINT('Ctrl Pts',(0.492708646638066,-3.36443516720367,
-31.2694722150127));
#31093=CARTESIAN_POINT('Ctrl Pts',(0.225363753175854,-3.39284610137639,
-31.2834540394444));
#31094=CARTESIAN_POINT('Ctrl Pts',(-0.177568226748785,-3.38778802702845,
-31.3049473012839));
#31095=CARTESIAN_POINT('Ctrl Pts',(-0.312354514032439,-3.37802700749997,
-31.3122280911118));
#31096=CARTESIAN_POINT('Ctrl Pts',(-0.483051111407701,-3.35536133102859,
-31.3219419687302));
#31097=CARTESIAN_POINT('Ctrl Pts',(-0.519831307236549,-3.34986017823292,
-31.324064799933));
#31098=CARTESIAN_POINT('Ctrl Pts',(-0.57646385365794,-3.34043464134589,
-31.3273896225132));
#31099=CARTESIAN_POINT('Ctrl Pts',(-0.596385091183429,-3.33693556216593,
-31.3285699686353));
#31100=CARTESIAN_POINT('Ctrl Pts',(-0.633999875348368,-3.32998111020143,
-31.3308211221208));
#31101=CARTESIAN_POINT('Ctrl Pts',(-0.651699041172491,-3.3265625409341,
-31.331889997046));
#31102=CARTESIAN_POINT('Ctrl Pts',(-0.695153995144886,-3.31780918677776,
-31.3345369701652));
#31103=CARTESIAN_POINT('Ctrl Pts',(-0.720876260432146,-3.3123155345849,
-31.3361233488398));
#31104=CARTESIAN_POINT('Ctrl Pts',(-0.815382451359608,-3.29097837628167,
-31.3420176290571));
#31105=CARTESIAN_POINT('Ctrl Pts',(-0.883726996536045,-3.2732877148343,
-31.3464088891587));
#31106=CARTESIAN_POINT('Ctrl Pts',(-1.15069441629301,-3.19521432818874,
-31.3639480880346));
#31107=CARTESIAN_POINT('Ctrl Pts',(-1.34414885486117,-3.1187748856563,-31.3774813509711));
#31108=CARTESIAN_POINT('Ctrl Pts',(-1.67265408044434,-2.95269397310375,
-31.4009737300191));
#31109=CARTESIAN_POINT('Ctrl Pts',(-1.8105999990087,-2.87017634948374,-31.4110255271459));
#31110=CARTESIAN_POINT('Ctrl Pts',(-1.98123214383969,-2.75088953250633,
-31.4236232491918));
#31111=CARTESIAN_POINT('Ctrl Pts',(-2.01969365205259,-2.72277651001239,
-31.4264757348992));
#31112=CARTESIAN_POINT('Ctrl Pts',(-2.08337439829182,-2.67413762220135,
-31.4312227803155));
#31113=CARTESIAN_POINT('Ctrl Pts',(-2.10891313394441,-2.65404340741461,
-31.4331333760073));
#31114=CARTESIAN_POINT('Ctrl Pts',(-2.15964403504852,-2.61293295846624,
-31.4369440892849));
#31115=CARTESIAN_POINT('Ctrl Pts',(-2.18482791607657,-2.59191205289224,
-31.4388437315206));
#31116=CARTESIAN_POINT('Ctrl Pts',(-2.2470661261945,-2.53841021860493,-31.4435612846616));
#31117=CARTESIAN_POINT('Ctrl Pts',(-2.28372541499067,-2.50548023100485,
-31.4463608035753));
#31118=CARTESIAN_POINT('Ctrl Pts',(-2.45952312509443,-2.34050069784782,
-31.4599145126943));
#31119=CARTESIAN_POINT('Ctrl Pts',(-2.58800306304386,-2.19760047538392,
-31.4702014995828));
#31120=CARTESIAN_POINT('Ctrl Pts',(-2.80117968844916,-1.91570047109187,
-31.4889814926882));
#31121=CARTESIAN_POINT('Ctrl Pts',(-2.88929913646434,-1.78001725553925,
-31.4974854665794));
#31122=CARTESIAN_POINT('Ctrl Pts',(-3.0063804044293,-1.56798722171135,-31.5107048219017));
#31123=CARTESIAN_POINT('Ctrl Pts',(-3.04282476609623,-1.49603563394987,
-31.5151816000568));
#31124=CARTESIAN_POINT('Ctrl Pts',(-3.08791348911589,-1.39853968837005,
-31.5213230846099));
#31125=CARTESIAN_POINT('Ctrl Pts',(-3.09887121004895,-1.3740888266969,-31.5228694658023));
#31126=CARTESIAN_POINT('Ctrl Pts',(-3.11674643476429,-1.33290082348334,
-31.5254887807842));
#31127=CARTESIAN_POINT('Ctrl Pts',(-3.12382196957048,-1.31623297210885,
-31.5265527020305));
#31128=CARTESIAN_POINT('Ctrl Pts',(-3.13843874201812,-1.28101840006851,
-31.5288100932665));
#31129=CARTESIAN_POINT('Ctrl Pts',(-3.14594967364051,-1.2624604887601,-31.5300050893711));
#31130=CARTESIAN_POINT('Ctrl Pts',(-3.16657198964786,-1.21018014684543,
-31.5333843687216));
#31131=CARTESIAN_POINT('Ctrl Pts',(-3.17930811826689,-1.17631365587963,
-31.5355882500344));
#31132=CARTESIAN_POINT('Ctrl Pts',(-3.25903044485002,-0.953566054130738,
-31.5501507697102));
#31133=CARTESIAN_POINT('Ctrl Pts',(-3.30969138629977,-0.759276356119579,
-31.5631406951041));
#31134=CARTESIAN_POINT('Ctrl Pts',(-3.37397414946623,-0.376681038970963,
-31.5881030590623));
#31135=CARTESIAN_POINT('Ctrl Pts',(-3.38964994078012,-0.18941699283998,
-31.6000439579888));
#31136=CARTESIAN_POINT('Ctrl Pts',(-3.38978312762711,0.0615147941664754,
-31.6154282675448));
#31137=CARTESIAN_POINT('Ctrl Pts',(-3.38804286396248,0.124820145480946,
-31.6192598203274));
#31138=CARTESIAN_POINT('Ctrl Pts',(-3.38253750698137,0.2239094912087,-31.6251815825254));
#31139=CARTESIAN_POINT('Ctrl Pts',(-3.37997471952741,0.259743122505757,
-31.6273075993727));
#31140=CARTESIAN_POINT('Ctrl Pts',(-3.3741402368697,0.326410161288458,-31.6312357700132));
#31141=CARTESIAN_POINT('Ctrl Pts',(-3.37101422179426,0.357252209755165,
-31.6330421747588));
#31142=CARTESIAN_POINT('Ctrl Pts',(-3.36295968665067,0.427149187713094,
-31.6371131890979));
#31143=CARTESIAN_POINT('Ctrl Pts',(-3.35777304254378,0.46617020530461,-31.6393696396726));
#31144=CARTESIAN_POINT('Ctrl Pts',(-3.33932622318197,0.588587283645547,
-31.6464045742842));
#31145=CARTESIAN_POINT('Ctrl Pts',(-3.32362880756328,0.671585956597162,
-31.651108833398));
#31146=CARTESIAN_POINT('Ctrl Pts',(-3.27739247631794,0.874266210733162,
-31.6625141662718));
#31147=CARTESIAN_POINT('Ctrl Pts',(-3.24338325313892,0.993030929851279,
-31.6691230888089));
#31148=CARTESIAN_POINT('Ctrl Pts',(-3.1379873819616,1.29724452423116,-31.6862442555137));
#31149=CARTESIAN_POINT('Ctrl Pts',(-3.05666034620139,1.47872372431097,-31.6966421048332));
#31150=CARTESIAN_POINT('Ctrl Pts',(-2.93219055899067,1.70173554570051,-31.7107787541576));
#31151=CARTESIAN_POINT('Ctrl Pts',(-2.90320223456133,1.75073167176077,-31.7139771063007));
#31152=CARTESIAN_POINT('Ctrl Pts',(-2.86123199463675,1.81775902758378,-31.7185152066177));
#31153=CARTESIAN_POINT('Ctrl Pts',(-2.849284439942,1.83642983382003,-31.7197973638296));
#31154=CARTESIAN_POINT('Ctrl Pts',(-2.82728133788243,1.87008311138499,-31.7221438584359));
#31155=CARTESIAN_POINT('Ctrl Pts',(-2.81728748102431,1.88510526156291,-31.7232043707742));
#31156=CARTESIAN_POINT('Ctrl Pts',(-2.79586161058957,1.91676034651899,-31.7254682511059));
#31157=CARTESIAN_POINT('Ctrl Pts',(-2.78440038023395,1.93337188589797,-31.726673343539));
#31158=CARTESIAN_POINT('Ctrl Pts',(-2.7515255730235,1.98012092380728,-31.7301111764313));
#31159=CARTESIAN_POINT('Ctrl Pts',(-2.72976691925459,2.01001098979437,-31.7323645531217));
#31160=CARTESIAN_POINT('Ctrl Pts',(-2.6274154052913,2.14588454376703,-31.7428434427406));
#31161=CARTESIAN_POINT('Ctrl Pts',(-2.5411158452899,2.24741117268509,-31.7513412359955));
#31162=CARTESIAN_POINT('Ctrl Pts',(-2.26819701550289,2.5326142250237,-31.7767190618677));
#31163=CARTESIAN_POINT('Ctrl Pts',(-2.0660095510784,2.70009185771265,-31.7936126499004));
#31164=CARTESIAN_POINT('Ctrl Pts',(-1.79665773550346,2.87505919633643,-31.8132402997515));
#31165=CARTESIAN_POINT('Ctrl Pts',(-1.74592067088237,2.90614969928204,-31.8168308718305));
#31166=CARTESIAN_POINT('Ctrl Pts',(-1.66423033155405,2.95329561085724,-31.8224480814199));
#31167=CARTESIAN_POINT('Ctrl Pts',(-1.63380441738222,2.97023581925327,-31.8245054388823));
#31168=CARTESIAN_POINT('Ctrl Pts',(-1.5753745936035,3.00159818893879,-31.8283923021979));
#31169=CARTESIAN_POINT('Ctrl Pts',(-1.54742032582661,3.01610464522101,-31.8302245892822));
#31170=CARTESIAN_POINT('Ctrl Pts',(-1.48224308591919,3.04878268597412,-31.8344360829827));
#31171=CARTESIAN_POINT('Ctrl Pts',(-1.4448807483035,3.06666598550343,-31.836805305535));
#31172=CARTESIAN_POINT('Ctrl Pts',(-1.31805167502983,3.12453945903911,-31.8447070252748));
#31173=CARTESIAN_POINT('Ctrl Pts',(-1.22717814192728,3.16133565592759,-31.8501349281128));
#31174=CARTESIAN_POINT('Ctrl Pts',(-0.986111908821109,3.24698288881799,
-31.8640751206751));
#31175=CARTESIAN_POINT('Ctrl Pts',(-0.833878446965317,3.28937138779607,
-31.8724232977448));
#31176=CARTESIAN_POINT('Ctrl Pts',(-0.506442979825628,3.35634170408778,
-31.890164647432));
#31177=CARTESIAN_POINT('Ctrl Pts',(-0.331164349304396,3.37814030561119,
-31.8995398491931));
#31178=CARTESIAN_POINT('Ctrl Pts',(-0.117553032608832,3.38791853982606,
-31.9115987182643));
#31179=CARTESIAN_POINT('Ctrl Pts',(-0.0800755107179769,3.38901142207123,
-31.913738332117));
#31180=CARTESIAN_POINT('Ctrl Pts',(-0.0223027143843366,3.38973734361808,
-31.9170837959744));
#31181=CARTESIAN_POINT('Ctrl Pts',(-0.00201488321266023,3.38981010751676,
-31.9182675736157));
#31182=CARTESIAN_POINT('Ctrl Pts',(0.0362765871823664,3.38960370143624,
-31.9205207864142));
#31183=CARTESIAN_POINT('Ctrl Pts',(0.0542792560688647,3.38936320699878,
-31.921588212222));
#31184=CARTESIAN_POINT('Ctrl Pts',(0.098436095638436,3.38842145000747,-31.9242252253323));
#31185=CARTESIAN_POINT('Ctrl Pts',(0.124585379097539,3.38756077128252,-31.9258029486986));
#31186=CARTESIAN_POINT('Ctrl Pts',(0.225616488988718,3.38306409652593,-31.9319543071364));
#31187=CARTESIAN_POINT('Ctrl Pts',(0.300375523299408,3.37724716842197,-31.9366239480884));
#31188=CARTESIAN_POINT('Ctrl Pts',(0.514852363709143,3.35338165008466,-31.9502518840086));
#31189=CARTESIAN_POINT('Ctrl Pts',(0.653718906426079,3.32909758153468,-31.9593545271832));
#31190=CARTESIAN_POINT('Ctrl Pts',(0.989310970128799,3.24859945502809,-31.9815659663391));
#31191=CARTESIAN_POINT('Ctrl Pts',(1.18326424187125,3.18308668880355,-31.9945659487405));
#31192=CARTESIAN_POINT('Ctrl Pts',(1.42227296697476,3.07746505795901,-32.0105037632757));
#31193=CARTESIAN_POINT('Ctrl Pts',(1.47380227550438,3.05312282948597,-32.0139374851677));
#31194=CARTESIAN_POINT('Ctrl Pts',(1.55534919393424,3.01205443055906,-32.0193699712372));
#31195=CARTESIAN_POINT('Ctrl Pts',(1.58576711087045,2.99615183304998,-32.0213960619647));
#31196=CARTESIAN_POINT('Ctrl Pts',(1.64375118639079,2.96470708365515,-32.0252593338896));
#31197=CARTESIAN_POINT('Ctrl Pts',(1.67135138484922,2.94923561315491,-32.0270987050851));
#31198=CARTESIAN_POINT('Ctrl Pts',(1.73552636554924,2.91207163013642,-32.0313788423397));
#31199=CARTESIAN_POINT('Ctrl Pts',(1.77191801240698,2.89007261667187,-32.0338085054089));
#31200=CARTESIAN_POINT('Ctrl Pts',(1.89768126572133,2.8107790876379,-32.0422245505969));
#31201=CARTESIAN_POINT('Ctrl Pts',(1.98477085140624,2.74997467757229,-32.0480855612713));
#31202=CARTESIAN_POINT('Ctrl Pts',(2.21393355248003,2.57341004853675,-32.0637920611664));
#31203=CARTESIAN_POINT('Ctrl Pts',(2.34970155506746,2.45007046090556,-32.0734064596452));
#31204=CARTESIAN_POINT('Ctrl Pts',(2.57014801469695,2.21454176109213,-32.0905967447949));
#31205=CARTESIAN_POINT('Ctrl Pts',(2.65906876710816,2.10694149250063,-32.0981020864618));
#31206=CARTESIAN_POINT('Ctrl Pts',(2.76310286252025,1.96394148972013,-32.1080709398795));
#31207=CARTESIAN_POINT('Ctrl Pts',(2.78460059642656,1.93333982615192,-32.1102041800757));
#31208=CARTESIAN_POINT('Ctrl Pts',(2.81708420911127,1.88543398810376,-32.1135539007433));
#31209=CARTESIAN_POINT('Ctrl Pts',(2.82842741694695,1.86837444469237,-32.1147487141164));
#31210=CARTESIAN_POINT('Ctrl Pts',(2.84941285908234,1.83618443932647,-32.117008950484));
#31211=CARTESIAN_POINT('Ctrl Pts',(2.85909067812979,1.8210786295864,-32.1180721204738));
#31212=CARTESIAN_POINT('Ctrl Pts',(2.8823611629749,1.78411371815477,-32.1206789683108));
#31213=CARTESIAN_POINT('Ctrl Pts',(2.89582542962505,1.76217553789551,-32.1222303431389));
#31214=CARTESIAN_POINT('Ctrl Pts',(2.94570527484293,1.67878753559441,-32.1281369079505));
#31215=CARTESIAN_POINT('Ctrl Pts',(2.98042331006988,1.61634855318705,-32.132579024001));
#31216=CARTESIAN_POINT('Ctrl Pts',(3.07234527818099,1.43798535665711,-32.1452297597084));
#31217=CARTESIAN_POINT('Ctrl Pts',(3.12492931626678,1.31981883226846,-32.1535629874766));
#31218=CARTESIAN_POINT('Ctrl Pts',(3.24880426378119,0.992228474152067,-32.176119208664));
#31219=CARTESIAN_POINT('Ctrl Pts',(3.3065788698723,0.778336777817994,-32.1902337703155));
#31220=CARTESIAN_POINT('Ctrl Pts',(3.35248530657016,0.504438051843582,-32.2071684646287));
#31221=CARTESIAN_POINT('Ctrl Pts',(3.36044900439171,0.448328609347779,-32.2105823844214));
#31222=CARTESIAN_POINT('Ctrl Pts',(3.37096480876573,0.358015257199794,-32.2159915193428));
#31223=CARTESIAN_POINT('Ctrl Pts',(3.37441095293715,0.323928256234341,-32.218013643369));
#31224=CARTESIAN_POINT('Ctrl Pts',(3.3800465500495,0.258249420312573,-32.2218741079838));
#31225=CARTESIAN_POINT('Ctrl Pts',(3.38231122830191,0.226667813291584,-32.2237145611959));
#31226=CARTESIAN_POINT('Ctrl Pts',(3.3865887272523,0.152456024550003,-32.2280043714101));
#31227=CARTESIAN_POINT('Ctrl Pts',(3.3882396699065,0.109809910105548,-32.2304424681138));
#31228=CARTESIAN_POINT('Ctrl Pts',(3.39121134650218,-0.0401882388950468,
-32.2389336755888));
#31229=CARTESIAN_POINT('Ctrl Pts',(3.38823803065253,-0.147564949478124,
-32.2448581995395));
#31230=CARTESIAN_POINT('Ctrl Pts',(3.36610672161663,-0.441358165040796,
-32.2608460982377));
#31231=CARTESIAN_POINT('Ctrl Pts',(3.33659166492752,-0.62660097884051,-32.2706663102546));
#31232=CARTESIAN_POINT('Ctrl Pts',(3.25714029832741,-0.950114912834011,
-32.2884352569169));
#31233=CARTESIAN_POINT('Ctrl Pts',(3.2132478738,-1.08936260214783,-32.2963064735893));
#31234=CARTESIAN_POINT('Ctrl Pts',(3.14929521940141,-1.25431688309618,-32.3063599861259));
#31235=CARTESIAN_POINT('Ctrl Pts',(3.13766154034045,-1.28314112082145,-32.3081448760513));
#31236=CARTESIAN_POINT('Ctrl Pts',(3.11829954372731,-1.32927505674184,-32.3110533355167));
#31237=CARTESIAN_POINT('Ctrl Pts',(3.1108192804485,-1.34668763553904,-32.3121631006307));
#31238=CARTESIAN_POINT('Ctrl Pts',(3.09562955989563,-1.38124437711319,-32.3143912659401));
#31239=CARTESIAN_POINT('Ctrl Pts',(3.08792272816441,-1.39838892493502,-32.315509501979));
#31240=CARTESIAN_POINT('Ctrl Pts',(3.06739895524313,-1.44304888086376,-32.318454249752));
#31241=CARTESIAN_POINT('Ctrl Pts',(3.05435455372184,-1.47045725694347,-32.320293355575));
#31242=CARTESIAN_POINT('Ctrl Pts',(2.98395928949409,-1.61338983658263,-32.3300384998974));
#31243=CARTESIAN_POINT('Ctrl Pts',(2.92042174311111,-1.72573777021295,-32.3382291574329));
#31244=CARTESIAN_POINT('Ctrl Pts',(2.69361283367331,-2.07823914721996,-32.3651213095349));
#31245=CARTESIAN_POINT('Ctrl Pts',(2.50585382551528,-2.30116920387337,-32.3839268416348));
#31246=CARTESIAN_POINT('Ctrl Pts',(2.25290887969975,-2.53330154638374,-32.4048001253975));
#31247=CARTESIAN_POINT('Ctrl Pts',(2.21301573554108,-2.568224478344,-32.407986713381));
#31248=CARTESIAN_POINT('Ctrl Pts',(2.14657718375927,-2.62368744553067,-32.4131274901556));
#31249=CARTESIAN_POINT('Ctrl Pts',(2.12051815003745,-2.64479343486468,-32.4151039633982));
#31250=CARTESIAN_POINT('Ctrl Pts',(2.06900042786337,-2.6852681727254,-32.4189359783705));
#31251=CARTESIAN_POINT('Ctrl Pts',(2.04357237033501,-2.70467003514258,-32.4207926903968));
#31252=CARTESIAN_POINT('Ctrl Pts',(1.98192580392429,-2.75034117936147,-32.425214084892));
#31253=CARTESIAN_POINT('Ctrl Pts',(1.94545392811741,-2.77625931278211,-32.4277653615304));
#31254=CARTESIAN_POINT('Ctrl Pts',(1.80491013733798,-2.8720043419099,-32.4373686253088));
#31255=CARTESIAN_POINT('Ctrl Pts',(1.69750361703348,-2.93676611928618,-32.4442388628275));
#31256=CARTESIAN_POINT('Ctrl Pts',(1.34415497828158,-3.123942761491,-32.4657902318559));
#31257=CARTESIAN_POINT('Ctrl Pts',(1.08687652711141,-3.22249015303326,-32.4798868563597));
#31258=CARTESIAN_POINT('Ctrl Pts',(0.769552245225484,-3.30165993559616,
-32.4980623491101));
#31259=CARTESIAN_POINT('Ctrl Pts',(0.718256367792776,-3.31319727398392,
-32.5010266801109));
#31260=CARTESIAN_POINT('Ctrl Pts',(0.644004175609585,-3.32809258626547,
-32.5053817130149));
#31261=CARTESIAN_POINT('Ctrl Pts',(0.621247062055888,-3.33241559001659,
-32.5067250631894));
#31262=CARTESIAN_POINT('Ctrl Pts',(0.581023092180704,-3.33963031317349,
-32.509117432149));
#31263=CARTESIAN_POINT('Ctrl Pts',(0.563575052827663,-3.34261897321262,
-32.5101612348143));
#31264=CARTESIAN_POINT('Ctrl Pts',(0.524552456121503,-3.34898889524847,
-32.5125097540141));
#31265=CARTESIAN_POINT('Ctrl Pts',(0.50296822981662,-3.35229843596043,-32.5138180573591));
#31266=CARTESIAN_POINT('Ctrl Pts',(0.436285988334247,-3.36186444418595,
-32.5178854159327));
#31267=CARTESIAN_POINT('Ctrl Pts',(0.39109435450394,-3.36742079155512,-32.5206777677869));
#31268=CARTESIAN_POINT('Ctrl Pts',(0.114982040658503,-3.39573624603538,
-32.5379027112432));
#31269=CARTESIAN_POINT('Ctrl Pts',(-0.117654664896214,-3.39564404651224,
-32.5530651210382));
#31270=CARTESIAN_POINT('Ctrl Pts',(-0.517842806298667,-3.35428736911374,
-32.578799343628));
#31271=CARTESIAN_POINT('Ctrl Pts',(-0.685691389440883,-3.3240405318538,
-32.5894941377782));
#31272=CARTESIAN_POINT('Ctrl Pts',(-0.897627094507028,-3.26910284516409,
-32.6027542036788));
#31273=CARTESIAN_POINT('Ctrl Pts',(-0.944413978038173,-3.25589471822949,
-32.6056671839362));
#31274=CARTESIAN_POINT('Ctrl Pts',(-1.01903147845844,-3.23308599954552,
-32.6102919403707));
#31275=CARTESIAN_POINT('Ctrl Pts',(-1.04704800175423,-3.22412170948235,
-32.6120236053747));
#31276=CARTESIAN_POINT('Ctrl Pts',(-1.10535487052155,-3.20462538044818,
-32.6156186140622));
#31277=CARTESIAN_POINT('Ctrl Pts',(-1.13561968478087,-3.19402586916629,
-32.6174795781308));
#31278=CARTESIAN_POINT('Ctrl Pts',(-1.20819941916067,-3.16744451709117,
-32.6219326170104));
#31279=CARTESIAN_POINT('Ctrl Pts',(-1.25035428585623,-3.15104189697381,
-32.6245107660179));
#31280=CARTESIAN_POINT('Ctrl Pts',(-1.41256033509321,-3.084158960479,-32.6344136924874));
#31281=CARTESIAN_POINT('Ctrl Pts',(-1.52999665373768,-3.0276192075684,-32.6415405300569));
#31282=CARTESIAN_POINT('Ctrl Pts',(-1.76616463944526,-2.89665564350464,
-32.6560718204154));
#31283=CARTESIAN_POINT('Ctrl Pts',(-1.8841220704842,-2.82135361801482,-32.6634438310438));
#31284=CARTESIAN_POINT('Ctrl Pts',(-2.11924823593796,-2.64991457901812,
-32.6789217512281));
#31285=CARTESIAN_POINT('Ctrl Pts',(-2.23529825359217,-2.55278156768532,
-32.6870223784718));
#31286=CARTESIAN_POINT('Ctrl Pts',(-2.37185952638152,-2.42200863642846,
-32.69767502404));
#31287=CARTESIAN_POINT('Ctrl Pts',(-2.39880820687299,-2.39532093594945,
-32.6998374277481));
#31288=CARTESIAN_POINT('Ctrl Pts',(-2.43969310712116,-2.35345000104187,
-32.7032232790171));
#31289=CARTESIAN_POINT('Ctrl Pts',(-2.45394890706871,-2.33858163829019,
-32.7044243185735));
#31290=CARTESIAN_POINT('Ctrl Pts',(-2.4803439031346,-2.31054537032509,-32.706688768304));
#31291=CARTESIAN_POINT('Ctrl Pts',(-2.49251561042367,-2.29740977253695,
-32.7077497902968));
#31292=CARTESIAN_POINT('Ctrl Pts',(-2.5217767051608,-2.26532523254966,-32.710340781097));
#31293=CARTESIAN_POINT('Ctrl Pts',(-2.53875705177506,-2.24627885761541,
-32.711878214781));
#31294=CARTESIAN_POINT('Ctrl Pts',(-2.60126714011425,-2.17454886619738,
-32.7176599079028));
#31295=CARTESIAN_POINT('Ctrl Pts',(-2.64538277147758,-2.12066078960656,
-32.7219866406303));
#31296=CARTESIAN_POINT('Ctrl Pts',(-2.76316635254191,-1.96738752660349,
-32.7341630345344));
#31297=CARTESIAN_POINT('Ctrl Pts',(-2.83310125761782,-1.86527125512021,
-32.7421280416902));
#31298=CARTESIAN_POINT('Ctrl Pts',(-3.01570796189553,-1.56459164389676,
-32.7647866628734));
#31299=CARTESIAN_POINT('Ctrl Pts',(-3.11415140262951,-1.35813482925953,
-32.7793827059522));
#31300=CARTESIAN_POINT('Ctrl Pts',(-3.21036196650114,-1.08960455034356,
-32.7967818562704));
#31301=CARTESIAN_POINT('Ctrl Pts',(-3.22825203253292,-1.03539916600064,
-32.8002212944883));
#31302=CARTESIAN_POINT('Ctrl Pts',(-3.25470122570166,-0.947894610968836,
-32.8056605203366));
#31303=CARTESIAN_POINT('Ctrl Pts',(-3.26413695295494,-0.914873949533435,
-32.807687755527));
#31304=CARTESIAN_POINT('Ctrl Pts',(-3.28129748812828,-0.851171227284105,
-32.8115518459151));
#31305=CARTESIAN_POINT('Ctrl Pts',(-3.2890976801872,-0.820513383675932,
-32.8133909133239));
#31306=CARTESIAN_POINT('Ctrl Pts',(-3.30636380053194,-0.74844348222983,
-32.8176683040146));
#31307=CARTESIAN_POINT('Ctrl Pts',(-3.31548283813274,-0.70695332569466,
-32.8200955689807));
#31308=CARTESIAN_POINT('Ctrl Pts',(-3.33789481238578,-0.594983969278794,
-32.8265599203939));
#31309=CARTESIAN_POINT('Ctrl Pts',(-3.34973529178031,-0.524234790278472,
-32.8305532037746));
#31310=CARTESIAN_POINT('Ctrl Pts',(-3.37971578929821,-0.301986095678115,
-32.8428764286686));
#31311=CARTESIAN_POINT('Ctrl Pts',(-3.38988114114937,-0.149605677499533,
-32.8509992266607));
#31312=CARTESIAN_POINT('Ctrl Pts',(-3.38974872291658,0.00294244548350111,
-32.859096383374));
#31313=CARTESIAN_POINT('',(-3.38974995202214,-0.000570320900454691,-35.3620086083019));
#31314=CARTESIAN_POINT('Ctrl Pts',(-3.38974872318309,0.00294213844468618,
-32.8590963670765));
#31315=CARTESIAN_POINT('Ctrl Pts',(-3.38957866884684,0.198868156207286,
-32.8694959947181));
#31316=CARTESIAN_POINT('Ctrl Pts',(-3.37242232301567,0.394398350512979,
-32.8798156181844));
#31317=CARTESIAN_POINT('Ctrl Pts',(-3.33313537108559,0.617709245412695,
-32.8925278884542));
#31318=CARTESIAN_POINT('Ctrl Pts',(-3.32737786332044,0.648006592528334,
-32.894273105052));
#31319=CARTESIAN_POINT('Ctrl Pts',(-3.31596013979505,0.703918576631977,
-32.8975387115144));
#31320=CARTESIAN_POINT('Ctrl Pts',(-3.31041437408373,0.729554379380284,
-32.8990536090901));
#31321=CARTESIAN_POINT('Ctrl Pts',(-3.30055880730922,0.772684379337358,
-32.9016359558564));
#31322=CARTESIAN_POINT('Ctrl Pts',(-3.29640589675622,0.790213733915254,
-32.9026949915034));
#31323=CARTESIAN_POINT('Ctrl Pts',(-3.28728614573419,0.827384602266697,
-32.9049621111853));
#31324=CARTESIAN_POINT('Ctrl Pts',(-3.28228271071418,0.847015729224043,
-32.9061720128739));
#31325=CARTESIAN_POINT('Ctrl Pts',(-3.26755553328994,0.902707482043506,
-32.909637894282));
#31326=CARTESIAN_POINT('Ctrl Pts',(-3.25741163036675,0.938652856744965,
-32.9119150157372));
#31327=CARTESIAN_POINT('Ctrl Pts',(-3.19363817663677,1.15113968372738,-32.9255861175308));
#31328=CARTESIAN_POINT('Ctrl Pts',(-3.12626398020651,1.323220216345,-32.9375076425619));
#31329=CARTESIAN_POINT('Ctrl Pts',(-2.97822509841098,1.62599209145817,-32.9592094683079));
#31330=CARTESIAN_POINT('Ctrl Pts',(-2.90204073986036,1.75836319971557,-32.9689816557687));
#31331=CARTESIAN_POINT('Ctrl Pts',(-2.76374814515095,1.96502839308152,-32.9845064626342));
#31332=CARTESIAN_POINT('Ctrl Pts',(-2.70692753078343,2.04259305868081,-32.9904039982188));
#31333=CARTESIAN_POINT('Ctrl Pts',(-2.6211770957806,2.14977413477992,-32.9986532948203));
#31334=CARTESIAN_POINT('Ctrl Pts',(-2.59488759754773,2.18143456846072,-33.001103614409));
#31335=CARTESIAN_POINT('Ctrl Pts',(-2.5474927236205,2.23644261433742,-33.0053870409631));
#31336=CARTESIAN_POINT('Ctrl Pts',(-2.52662691652593,2.25998921840134,-33.0072294053604));
#31337=CARTESIAN_POINT('Ctrl Pts',(-2.48188991857644,2.30907978787897,-33.011090907111));
#31338=CARTESIAN_POINT('Ctrl Pts',(-2.45794517609485,2.33455192203991,-33.0131066939468));
#31339=CARTESIAN_POINT('Ctrl Pts',(-2.39171888237064,2.40285399489646,-33.0185493776631));
#31340=CARTESIAN_POINT('Ctrl Pts',(-2.34868305766029,2.44493661133928,-33.0219439673234));
#31341=CARTESIAN_POINT('Ctrl Pts',(-2.1133402605214,2.66311472301906,-33.0398233995884));
#31342=CARTESIAN_POINT('Ctrl Pts',(-1.90232570433707,2.81772074200772,-33.0534249805982));
#31343=CARTESIAN_POINT('Ctrl Pts',(-1.56015434101048,3.01230504697545,-33.0744304859596));
#31344=CARTESIAN_POINT('Ctrl Pts',(-1.44088863834648,3.07113937230117,-33.0816020837599));
#31345=CARTESIAN_POINT('Ctrl Pts',(-1.28445919895993,3.13718570874788,-33.0911835336884));
#31346=CARTESIAN_POINT('Ctrl Pts',(-1.25019721851796,3.15099607866703,-33.0932926378725));
#31347=CARTESIAN_POINT('Ctrl Pts',(-1.19688439897962,3.17147912762038,-33.0966005732746));
#31348=CARTESIAN_POINT('Ctrl Pts',(-1.1779871932423,3.17854656245025,-33.0977781059149));
#31349=CARTESIAN_POINT('Ctrl Pts',(-1.14207033862947,3.19161496064862,-33.1000276191938));
#31350=CARTESIAN_POINT('Ctrl Pts',(-1.1250640855269,3.19764936499773,-33.1010977309092));
#31351=CARTESIAN_POINT('Ctrl Pts',(-1.08304309323718,3.21218316602493,-33.1037530954693));
#31352=CARTESIAN_POINT('Ctrl Pts',(-1.05797590562231,3.22052634247081,-33.1053467502759));
#31353=CARTESIAN_POINT('Ctrl Pts',(-0.964746968840573,3.25035008771109,
-33.1113027622695));
#31354=CARTESIAN_POINT('Ctrl Pts',(-0.896012165114405,3.26996532337549,
-33.115750637736));
#31355=CARTESIAN_POINT('Ctrl Pts',(-0.581828885308255,3.34897617773903,
-33.1361875176625));
#31356=CARTESIAN_POINT('Ctrl Pts',(-0.33082662813074,3.38300639984154,-33.1527311279377));
#31357=CARTESIAN_POINT('Ctrl Pts',(0.0435898422567594,3.39166400082765,
-33.1763644577356));
#31358=CARTESIAN_POINT('Ctrl Pts',(0.165612339454509,3.38789943257147,-33.1839172779407));
#31359=CARTESIAN_POINT('Ctrl Pts',(0.331404875001098,3.37380290817119,-33.193953109855));
#31360=CARTESIAN_POINT('Ctrl Pts',(0.375555479367614,3.36917402563424,-33.1966041947997));
#31361=CARTESIAN_POINT('Ctrl Pts',(0.451283049186981,3.35972734719554,-33.2011164399241));
#31362=CARTESIAN_POINT('Ctrl Pts',(0.482905399583395,3.35532810858078,-33.2029901562619));
#31363=CARTESIAN_POINT('Ctrl Pts',(0.54771237002634,3.34537709322387,-33.2068101369835));
#31364=CARTESIAN_POINT('Ctrl Pts',(0.580886005924621,3.33977668437849,-33.2087546740464));
#31365=CARTESIAN_POINT('Ctrl Pts',(0.666645530648735,3.32398216690663,-33.2137566853829));
#31366=CARTESIAN_POINT('Ctrl Pts',(0.719083919677958,3.31303372501736,-33.2167906374287));
#31367=CARTESIAN_POINT('Ctrl Pts',(1.051316999132,3.23540745781591,-33.2358990552825));
#31368=CARTESIAN_POINT('Ctrl Pts',(1.32191154160378,3.13459454853511,-33.2508204427465));
#31369=CARTESIAN_POINT('Ctrl Pts',(1.69197484666758,2.94017527281209,-33.2731970795905));
#31370=CARTESIAN_POINT('Ctrl Pts',(1.80380800333793,2.87292181622552,-33.2802776265961));
#31371=CARTESIAN_POINT('Ctrl Pts',(1.93659994096173,2.7822492796301,-33.2894230377376));
#31372=CARTESIAN_POINT('Ctrl Pts',(1.96148841441477,2.76475920276684,-33.2911710611914));
#31373=CARTESIAN_POINT('Ctrl Pts',(2.00138093772629,2.7359154327832,-33.2940341499721));
#31374=CARTESIAN_POINT('Ctrl Pts',(2.0165322899965,2.72476721995828,-33.2951361834862));
#31375=CARTESIAN_POINT('Ctrl Pts',(2.04674874983643,2.70214419054493,-33.2973652021991));
#31376=CARTESIAN_POINT('Ctrl Pts',(2.06181202094502,2.69066809991932,-33.2984922457848));
#31377=CARTESIAN_POINT('Ctrl Pts',(2.10129022621982,2.6600651045834,-33.30148635143));
#31378=CARTESIAN_POINT('Ctrl Pts',(2.12553964540491,2.64072869561797,-33.3033667417317));
#31379=CARTESIAN_POINT('Ctrl Pts',(2.25679852348598,2.53308401193048,-33.3137577625229));
#31380=CARTESIAN_POINT('Ctrl Pts',(2.35856613850709,2.4386088768473,-33.3225956154495));
#31381=CARTESIAN_POINT('Ctrl Pts',(2.54603097230073,2.24183762419599,-33.3400577281402));
#31382=CARTESIAN_POINT('Ctrl Pts',(2.63206243720546,2.14017722431417,-33.348660850376));
#31383=CARTESIAN_POINT('Ctrl Pts',(2.77530323336927,1.94917069204475,-33.3638871783714));
#31384=CARTESIAN_POINT('Ctrl Pts',(2.83472522296516,1.86169552257456,-33.3705467941004));
#31385=CARTESIAN_POINT('Ctrl Pts',(2.92979231201171,1.70661329945789,-33.3817852073502));
#31386=CARTESIAN_POINT('Ctrl Pts',(2.96741820017876,1.64031781556161,-33.3864235667379));
#31387=CARTESIAN_POINT('Ctrl Pts',(3.02039556579916,1.5391741693539,-33.3932576355401));
#31388=CARTESIAN_POINT('Ctrl Pts',(3.03744570458595,1.50524757563404,-33.3955106928335));
#31389=CARTESIAN_POINT('Ctrl Pts',(3.06746920513162,1.44291792209281,-33.3995807433197));
#31390=CARTESIAN_POINT('Ctrl Pts',(3.08062681348076,1.4146087749619,-33.4014038303834));
#31391=CARTESIAN_POINT('Ctrl Pts',(3.10858143611425,1.35222274311065,-33.4053678223855));
#31392=CARTESIAN_POINT('Ctrl Pts',(3.1232132044165,1.31807599436185,-33.4075030335856));
#31393=CARTESIAN_POINT('Ctrl Pts',(3.16357460837197,1.21943487838255,-33.4135782327898));
#31394=CARTESIAN_POINT('Ctrl Pts',(3.18788863150178,1.15437978807924,-33.4174722390013));
#31395=CARTESIAN_POINT('Ctrl Pts',(3.28990248112387,0.853555334395103,-33.4350461858672));
#31396=CARTESIAN_POINT('Ctrl Pts',(3.34355605048408,0.610452166633055,-33.4479886636889));
#31397=CARTESIAN_POINT('Ctrl Pts',(3.38402099983914,0.23545043532618,-33.4681352554235));
#31398=CARTESIAN_POINT('Ctrl Pts',(3.39052704336033,0.106562978730718,-33.4751066392919));
#31399=CARTESIAN_POINT('Ctrl Pts',(3.38943548683829,-0.0588438593883352,
-33.4844451816288));
#31400=CARTESIAN_POINT('Ctrl Pts',(3.38860607986942,-0.0953107055720004,
-33.4865286472478));
#31401=CARTESIAN_POINT('Ctrl Pts',(3.38640792825984,-0.151821088923058,
-33.4898050306639));
#31402=CARTESIAN_POINT('Ctrl Pts',(3.38544914787157,-0.171878803259563,
-33.4909772908814));
#31403=CARTESIAN_POINT('Ctrl Pts',(3.38330002324623,-0.209775173124198,
-33.4932117517844));
#31404=CARTESIAN_POINT('Ctrl Pts',(3.38214667163084,-0.227614820294416,
-33.4942720210313));
#31405=CARTESIAN_POINT('Ctrl Pts',(3.37924351783717,-0.26760413441439,-33.4966666046545));
#31406=CARTESIAN_POINT('Ctrl Pts',(3.37741693247253,-0.289747360750057,
-33.4980048174597));
#31407=CARTESIAN_POINT('Ctrl Pts',(3.37009055105826,-0.369040780045293,
-33.5028370649734));
#31408=CARTESIAN_POINT('Ctrl Pts',(3.36335690972538,-0.426064475356408,
-33.5063870217699));
#31409=CARTESIAN_POINT('Ctrl Pts',(3.31703629659566,-0.747908371550464,
-33.5267500540963));
#31410=CARTESIAN_POINT('Ctrl Pts',(3.24762896243497,-1.00747945967103,-33.5443411831996));
#31411=CARTESIAN_POINT('Ctrl Pts',(3.10230691174956,-1.37170118010862,-33.5691078137422));
#31412=CARTESIAN_POINT('Ctrl Pts',(3.04989263227307,-1.48459852164717,-33.5768141087772));
#31413=CARTESIAN_POINT('Ctrl Pts',(2.97038993195384,-1.63376294591257,-33.5870117226861));
#31414=CARTESIAN_POINT('Ctrl Pts',(2.9486171303427,-1.67273877620257,-33.5896784474023));
#31415=CARTESIAN_POINT('Ctrl Pts',(2.90994236706701,-1.73886811106582,-33.594208789621));
#31416=CARTESIAN_POINT('Ctrl Pts',(2.89341481812748,-1.76623262374934,-33.5960852266785));
#31417=CARTESIAN_POINT('Ctrl Pts',(2.85874643571015,-1.82183979749035,-33.5999035726923));
#31418=CARTESIAN_POINT('Ctrl Pts',(2.84056822242917,-1.85005505907499,-33.6018438621193));
#31419=CARTESIAN_POINT('Ctrl Pts',(2.79252068678727,-1.92225374287121,-33.6068194048722));
#31420=CARTESIAN_POINT('Ctrl Pts',(2.76202980001436,-1.96581358477319,-33.6098316299965));
#31421=CARTESIAN_POINT('Ctrl Pts',(2.55895521573008,-2.24187121186073,-33.6290318828746));
#31422=CARTESIAN_POINT('Ctrl Pts',(2.35822015009203,-2.45215008703459,-33.644046316049));
#31423=CARTESIAN_POINT('Ctrl Pts',(2.03266072350545,-2.71577441501087,-33.66647647633));
#31424=CARTESIAN_POINT('Ctrl Pts',(1.92755529004081,-2.79135533015354,-33.6735037019972));
#31425=CARTESIAN_POINT('Ctrl Pts',(1.79276813939869,-2.87703144063635,-33.6825880708323));
#31426=CARTESIAN_POINT('Ctrl Pts',(1.76691930133804,-2.89297831983318,-33.6843334691911));
#31427=CARTESIAN_POINT('Ctrl Pts',(1.72472846438684,-2.91823067344946,-33.6871933323607));
#31428=CARTESIAN_POINT('Ctrl Pts',(1.7085166108802,-2.92775161114048,-33.6882948200472));
#31429=CARTESIAN_POINT('Ctrl Pts',(1.67580924936994,-2.94659590525321,-33.6905239381613));
#31430=CARTESIAN_POINT('Ctrl Pts',(1.65931313132667,-2.95591677207997,-33.6916516428141));
#31431=CARTESIAN_POINT('Ctrl Pts',(1.61556752419028,-2.98015295310937,-33.6946494479529));
#31432=CARTESIAN_POINT('Ctrl Pts',(1.58819023387242,-2.99483249650858,-33.6965329324586));
#31433=CARTESIAN_POINT('Ctrl Pts',(1.43417981086195,-3.07470638109278,-33.7071533340132));
#31434=CARTESIAN_POINT('Ctrl Pts',(1.30374680507852,-3.13224013398883,-33.7162352510922));
#31435=CARTESIAN_POINT('Ctrl Pts',(0.991988016320563,-3.24690288187274,
-33.7375873191414));
#31436=CARTESIAN_POINT('Ctrl Pts',(0.808679744261229,-3.29734214961956,
-33.7498625336535));
#31437=CARTESIAN_POINT('Ctrl Pts',(0.515875549986654,-3.35200771303694,
-33.7685575933023));
#31438=CARTESIAN_POINT('Ctrl Pts',(0.408750135695405,-3.36675070969322,
-33.775218007896));
#31439=CARTESIAN_POINT('Ctrl Pts',(0.258499667809446,-3.38014965848058,
-33.7843004630683));
#31440=CARTESIAN_POINT('Ctrl Pts',(0.215835624946258,-3.3831418865376,-33.7868509298278));
#31441=CARTESIAN_POINT('Ctrl Pts',(0.141492719894735,-3.38694376729331,
-33.7912475597717));
#31442=CARTESIAN_POINT('Ctrl Pts',(0.109838688705697,-3.38811803745276,
-33.7931046085018));
#31443=CARTESIAN_POINT('Ctrl Pts',(0.0439598811176838,-3.38963769235233,
-33.7969400305457));
#31444=CARTESIAN_POINT('Ctrl Pts',(0.00973688866917836,-3.3899087705436,
-33.7989159259696));
#31445=CARTESIAN_POINT('Ctrl Pts',(-0.080960575403858,-3.3892536161392,
-33.804112141181));
#31446=CARTESIAN_POINT('Ctrl Pts',(-0.13741891611573,-3.38743431493963,
-33.8073052006884));
#31447=CARTESIAN_POINT('Ctrl Pts',(-0.418287936822755,-3.3713494130525,
-33.8230238930198));
#31448=CARTESIAN_POINT('Ctrl Pts',(-0.640934407026466,-3.33619167029793,
-33.8349084265437));
#31449=CARTESIAN_POINT('Ctrl Pts',(-0.981118889564493,-3.24713465271878,
-33.853576931239));
#31450=CARTESIAN_POINT('Ctrl Pts',(-1.10185977840245,-3.20817383771495,
-33.8603209193196));
#31451=CARTESIAN_POINT('Ctrl Pts',(-1.28603381854589,-3.1371184567035,-33.8711575933531));
#31452=CARTESIAN_POINT('Ctrl Pts',(-1.35112460440021,-3.10963923367563,
-33.8751001673527));
#31453=CARTESIAN_POINT('Ctrl Pts',(-1.43860594519594,-3.06944222389113,
-33.8806147491272));
#31454=CARTESIAN_POINT('Ctrl Pts',(-1.46178395586088,-3.05847187539271,
-33.8820970073651));
#31455=CARTESIAN_POINT('Ctrl Pts',(-1.50094949792565,-3.03938760602815,
-33.8846415242646));
#31456=CARTESIAN_POINT('Ctrl Pts',(-1.51700096358366,-3.03140800314464,
-33.8856959474534));
#31457=CARTESIAN_POINT('Ctrl Pts',(-1.55130389997304,-3.01401442373805,
-33.8879753911136));
#31458=CARTESIAN_POINT('Ctrl Pts',(-1.56953342889787,-3.00456178252967,
-33.8892025200976));
#31459=CARTESIAN_POINT('Ctrl Pts',(-1.62091720148741,-2.97732229379212,
-33.8927039224996));
#31460=CARTESIAN_POINT('Ctrl Pts',(-1.65386183810675,-2.95914876028468,
-33.8949994256224));
#31461=CARTESIAN_POINT('Ctrl Pts',(-1.81284582266028,-2.86796289152058,
-33.9063011959732));
#31462=CARTESIAN_POINT('Ctrl Pts',(-1.934384475333,-2.78743097472684,-33.9156309140578));
#31463=CARTESIAN_POINT('Ctrl Pts',(-2.15239428135991,-2.62183569639369,
-33.9332521156799));
#31464=CARTESIAN_POINT('Ctrl Pts',(-2.24995789486095,-2.5386049520326,-33.941520479365));
#31465=CARTESIAN_POINT('Ctrl Pts',(-2.4473319423018,-2.34988871627047,-33.9588792498742));
#31466=CARTESIAN_POINT('Ctrl Pts',(-2.54556462969428,-2.24310495068206,
-33.9679153428951));
#31467=CARTESIAN_POINT('Ctrl Pts',(-2.66590769863997,-2.09415990671961,
-33.9794897570944));
#31468=CARTESIAN_POINT('Ctrl Pts',(-2.69439960228897,-2.05737227460727,
-33.9822734032208));
#31469=CARTESIAN_POINT('Ctrl Pts',(-2.74136944304887,-1.99407657726352,
-33.9869398289304));
#31470=CARTESIAN_POINT('Ctrl Pts',(-2.76024156809812,-1.96787052723638,
-33.9888374327708));
#31471=CARTESIAN_POINT('Ctrl Pts',(-2.79766495426263,-1.91430617016825,
-33.9926487411673));
#31472=CARTESIAN_POINT('Ctrl Pts',(-2.81619630786475,-1.8869382015794,-33.994561572194));
#31473=CARTESIAN_POINT('Ctrl Pts',(-2.86205476548722,-1.81703147911282,
-33.9993640824283));
#31474=CARTESIAN_POINT('Ctrl Pts',(-2.88883639316144,-1.77414360803328,
-34.0022338772806));
#31475=CARTESIAN_POINT('Ctrl Pts',(-3.05520077975636,-1.49396679694007,
-34.020531227001));
#31476=CARTESIAN_POINT('Ctrl Pts',(-3.16639252441545,-1.24103021760397,
-34.0348996042033));
#31477=CARTESIAN_POINT('Ctrl Pts',(-3.28831183410698,-0.836165232795949,
-34.0574463648084));
#31478=CARTESIAN_POINT('Ctrl Pts',(-3.32157799672088,-0.692298984761503,
-34.0654022834829));
#31479=CARTESIAN_POINT('Ctrl Pts',(-3.35037701063691,-0.516085070735116,
-34.0755489351574));
#31480=CARTESIAN_POINT('Ctrl Pts',(-3.35496528964148,-0.485363446006798,
-34.0773326563309));
#31481=CARTESIAN_POINT('Ctrl Pts',(-3.36167147105276,-0.43580841250091,
-34.0802396765024));
#31482=CARTESIAN_POINT('Ctrl Pts',(-3.36405483759344,-0.417012066758022,
-34.0813491957314));
#31483=CARTESIAN_POINT('Ctrl Pts',(-3.36822372475534,-0.381769120537876,
-34.0834440356721));
#31484=CARTESIAN_POINT('Ctrl Pts',(-3.37004667018608,-0.365327433925368,
-34.0844272409039));
#31485=CARTESIAN_POINT('Ctrl Pts',(-3.37464780142137,-0.320858992556897,
-34.087101199132));
#31486=CARTESIAN_POINT('Ctrl Pts',(-3.37719709385888,-0.29281043892541,
-34.0888036252799));
#31487=CARTESIAN_POINT('Ctrl Pts',(-3.38624523605637,-0.177308788198433,
-34.0958702750957));
#31488=CARTESIAN_POINT('Ctrl Pts',(-3.38969829837649,-0.0896566665961387,
-34.1013646723238));
#31489=CARTESIAN_POINT('Ctrl Pts',(-3.38986499262025,0.19622356003253,-34.1195194495297));
#31490=CARTESIAN_POINT('Ctrl Pts',(-3.37259756120772,0.394052114179757,
-34.1324249634223));
#31491=CARTESIAN_POINT('Ctrl Pts',(-3.31234492261008,0.735392055258899,
-34.1544906165657));
#31492=CARTESIAN_POINT('Ctrl Pts',(-3.2769745204564,0.879702997720911,-34.1637602107885));
#31493=CARTESIAN_POINT('Ctrl Pts',(-3.21785727187418,1.06680971605334,-34.1756353193021));
#31494=CARTESIAN_POINT('Ctrl Pts',(-3.20249875485041,1.11206585444116,-34.1784971490572));
#31495=CARTESIAN_POINT('Ctrl Pts',(-3.17619591121179,1.1845005706199,-34.1830627896972));
#31496=CARTESIAN_POINT('Ctrl Pts',(-3.16584766920085,1.21188724039255,-34.1847855454195));
#31497=CARTESIAN_POINT('Ctrl Pts',(-3.14337838573098,1.26909952519826,-34.1883783677504));
#31498=CARTESIAN_POINT('Ctrl Pts',(-3.13118458828062,1.29889355165416,-34.1902458352731));
#31499=CARTESIAN_POINT('Ctrl Pts',(-3.10055815166929,1.37078658483829,-34.1947458834263));
#31500=CARTESIAN_POINT('Ctrl Pts',(-3.08169000842965,1.41269377036442,-34.1973637612878));
#31501=CARTESIAN_POINT('Ctrl Pts',(-3.00273330698203,1.57894495535171,-34.2077440297647));
#31502=CARTESIAN_POINT('Ctrl Pts',(-2.93592171848532,1.6999539588631,-34.2152809706273));
#31503=CARTESIAN_POINT('Ctrl Pts',(-2.78756965916299,1.9336760536422,-34.2301414609723));
#31504=CARTESIAN_POINT('Ctrl Pts',(-2.70611237850348,2.04611921764427,-34.2374503637462));
#31505=CARTESIAN_POINT('Ctrl Pts',(-2.526915263411,2.26399257682621,-34.252472741218));
#31506=CARTESIAN_POINT('Ctrl Pts',(-2.42890958920908,2.36882966747253,-34.2601777563289));
#31507=CARTESIAN_POINT('Ctrl Pts',(-2.29725315033719,2.49287824440455,-34.2703734605083));
#31508=CARTESIAN_POINT('Ctrl Pts',(-2.26950943323998,2.51816216103339,-34.2725143350504));
#31509=CARTESIAN_POINT('Ctrl Pts',(-2.22596178515698,2.55654456245038,-34.2758735158974));
#31510=CARTESIAN_POINT('Ctrl Pts',(-2.21044833637498,2.56996966414165,-34.2770699622021));
#31511=CARTESIAN_POINT('Ctrl Pts',(-2.18114871188186,2.59486356512339,-34.2793312869031));
#31512=CARTESIAN_POINT('Ctrl Pts',(-2.16739192096898,2.60636506081742,-34.2803938766907));
#31513=CARTESIAN_POINT('Ctrl Pts',(-2.13371275474353,2.63407183731994,-34.2829964885894));
#31514=CARTESIAN_POINT('Ctrl Pts',(-2.11369650202648,2.65016066944794,-34.284544145777));
#31515=CARTESIAN_POINT('Ctrl Pts',(-2.03770255909218,2.70983513744212,-34.2904171095247));
#31516=CARTESIAN_POINT('Ctrl Pts',(-1.98054695187105,2.75188491476045,-34.29482813212));
#31517=CARTESIAN_POINT('Ctrl Pts',(-1.81691705377377,2.86452958928056,-34.3073497153043));
#31518=CARTESIAN_POINT('Ctrl Pts',(-1.70771047857385,2.93094521640858,-34.3155823397102));
#31519=CARTESIAN_POINT('Ctrl Pts',(-1.39794646147904,3.09613213965208,-34.3381927643107));
#31520=CARTESIAN_POINT('Ctrl Pts',(-1.19094028928378,3.18150530386029,-34.3524638279715));
#31521=CARTESIAN_POINT('Ctrl Pts',(-0.922863179302594,3.26219663220974,
-34.3695336105765));
#31522=CARTESIAN_POINT('Ctrl Pts',(-0.868308411390444,3.27713966571272,
-34.3729408330519));
#31523=CARTESIAN_POINT('Ctrl Pts',(-0.780166540973884,3.29892669935651,
-34.3783420690312));
#31524=CARTESIAN_POINT('Ctrl Pts',(-0.746806930282671,3.30663828323955,
-34.3803628507207));
#31525=CARTESIAN_POINT('Ctrl Pts',(-0.682376401614594,3.32050754739192,
-34.3842223758094));
#31526=CARTESIAN_POINT('Ctrl Pts',(-0.651324929650731,3.32673772049028,
-34.3860632055121));
#31527=CARTESIAN_POINT('Ctrl Pts',(-0.578185287944982,3.34034913326486,
-34.3903563437231));
#31528=CARTESIAN_POINT('Ctrl Pts',(-0.536035371616945,3.34737163616403,
-34.3927973378157));
#31529=CARTESIAN_POINT('Ctrl Pts',(-0.387144033458921,3.36929347115258,
-34.4013145772699));
#31530=CARTESIAN_POINT('Ctrl Pts',(-0.279832129318265,3.37989879741465,
-34.407261111356));
#31531=CARTESIAN_POINT('Ctrl Pts',(0.0162888364614813,3.39496036038646,
-34.4233481261632));
#31532=CARTESIAN_POINT('Ctrl Pts',(0.205236842147306,3.38879035950003,-34.4332410926898));
#31533=CARTESIAN_POINT('Ctrl Pts',(0.535591867762952,3.35026039985449,-34.4509882791587));
#31534=CARTESIAN_POINT('Ctrl Pts',(0.677272857068071,3.32451450141487,-34.4587575406116));
#31535=CARTESIAN_POINT('Ctrl Pts',(0.847033040975952,3.28236282430959,-34.4686973678093));
#31536=CARTESIAN_POINT('Ctrl Pts',(0.877086165916422,3.27446032134965,-34.4704817761839));
#31537=CARTESIAN_POINT('Ctrl Pts',(0.925283917335664,3.26107556237097,-34.473389642628));
#31538=CARTESIAN_POINT('Ctrl Pts',(0.943499255967374,3.25585215690295,-34.4744993064328));
#31539=CARTESIAN_POINT('Ctrl Pts',(0.979696012736823,3.24514316926176,-34.4767274766792));
#31540=CARTESIAN_POINT('Ctrl Pts',(0.997677465724576,3.2396601827859,-34.4778458218761));
#31541=CARTESIAN_POINT('Ctrl Pts',(1.04457920921106,3.2249311928968,-34.4807911841795));
#31542=CARTESIAN_POINT('Ctrl Pts',(1.0734219563561,3.21544586144648,-34.4826308044277));
#31543=CARTESIAN_POINT('Ctrl Pts',(1.2242683493533,3.16358225111707,-34.4923874122592));
#31544=CARTESIAN_POINT('Ctrl Pts',(1.34389454423919,3.1146472177287,-34.5005897915081));
#31545=CARTESIAN_POINT('Ctrl Pts',(1.72202210299792,2.93412253094872,-34.5274727874733));
#31546=CARTESIAN_POINT('Ctrl Pts',(1.96657109824326,2.77616427900633,-34.5462559396613));
#31547=CARTESIAN_POINT('Ctrl Pts',(2.2285851371409,2.55472714592498,-34.5671144135563));
#31548=CARTESIAN_POINT('Ctrl Pts',(2.26831695113063,2.51951606195062,-34.5703053172204));
#31549=CARTESIAN_POINT('Ctrl Pts',(2.33178286696648,2.46055258032382,-34.5754511906831));
#31550=CARTESIAN_POINT('Ctrl Pts',(2.35601892117614,2.43735621165582,-34.5774285298408));
#31551=CARTESIAN_POINT('Ctrl Pts',(2.40267621904569,2.39135410105182,-34.5812610067906));
#31552=CARTESIAN_POINT('Ctrl Pts',(2.42512687988977,2.36858336741602,-34.5831173338275));
#31553=CARTESIAN_POINT('Ctrl Pts',(2.47817683671519,2.31323194349525,-34.587535821545));
#31554=CARTESIAN_POINT('Ctrl Pts',(2.50846091470029,2.28035667389836,-34.5900846240504));
#31555=CARTESIAN_POINT('Ctrl Pts',(2.6208639491699,2.15338625817068,-34.5996611177607));
#31556=CARTESIAN_POINT('Ctrl Pts',(2.69841485700287,2.05537385074105,-34.6065084660344));
#31557=CARTESIAN_POINT('Ctrl Pts',(2.92675341583585,1.73151851596639,-34.627868749138));
#31558=CARTESIAN_POINT('Ctrl Pts',(3.05590866610436,1.49179038285107,-34.641812778129));
#31559=CARTESIAN_POINT('Ctrl Pts',(3.17497918389823,1.18864186072428,-34.6598756371091));
#31560=CARTESIAN_POINT('Ctrl Pts',(3.19363812211422,1.13755755074913,-34.6629360347239));
#31561=CARTESIAN_POINT('Ctrl Pts',(3.21803978615924,1.06541057383332,-34.6673097554696));
#31562=CARTESIAN_POINT('Ctrl Pts',(3.22482098102185,1.04470538611959,-34.6685708116522));
#31563=CARTESIAN_POINT('Ctrl Pts',(3.23682770593384,1.00681383645763,-34.6708916776225));
#31564=CARTESIAN_POINT('Ctrl Pts',(3.24211717801349,0.98964836873316,-34.6719479791831));
#31565=CARTESIAN_POINT('Ctrl Pts',(3.25312675478436,0.952884133955721,-34.6742219621565));
#31566=CARTESIAN_POINT('Ctrl Pts',(3.25880653168419,0.933274770969195,-34.6754416485859));
#31567=CARTESIAN_POINT('Ctrl Pts',(3.27458375400896,0.876903459717626,-34.6789649282103));
#31568=CARTESIAN_POINT('Ctrl Pts',(3.28423831468145,0.840021947107023,-34.681290714281));
#31569=CARTESIAN_POINT('Ctrl Pts',(3.32723231452811,0.663691881831474,-34.6924832295635));
#31570=CARTESIAN_POINT('Ctrl Pts',(3.35232188866183,0.522392143099672,-34.7016620793814));
#31571=CARTESIAN_POINT('Ctrl Pts',(3.39787408297614,0.118546318921703,-34.7278167189869));
#31572=CARTESIAN_POINT('Ctrl Pts',(3.39683557008148,-0.14543756773046,-34.7447406300557));
#31573=CARTESIAN_POINT('Ctrl Pts',(3.35898735129977,-0.458638414500808,
-34.7639107261228));
#31574=CARTESIAN_POINT('Ctrl Pts',(3.35150412743073,-0.510456423024906,
-34.7670560265971));
#31575=CARTESIAN_POINT('Ctrl Pts',(3.33728503183569,-0.595020379461398,
-34.7721480466641));
#31576=CARTESIAN_POINT('Ctrl Pts',(3.33126001244793,-0.627875372821941,
-34.7741162439637));
#31577=CARTESIAN_POINT('Ctrl Pts',(3.31850249708846,-0.692079408598487,
-34.7779440259821));
#31578=CARTESIAN_POINT('Ctrl Pts',(3.31180890851199,-0.723432503409318,
-34.779804597304));
#31579=CARTESIAN_POINT('Ctrl Pts',(3.29461194556609,-0.798735684208286,
-34.7842547468235));
#31580=CARTESIAN_POINT('Ctrl Pts',(3.2836724861106,-0.84258046477976,-34.7868304467869));
#31581=CARTESIAN_POINT('Ctrl Pts',(3.2379347793336,-1.01144550313212,-34.7967053535089));
#31582=CARTESIAN_POINT('Ctrl Pts',(3.19684449558154,-1.13465127065709,-34.8038081690403));
#31583=CARTESIAN_POINT('Ctrl Pts',(3.09611256668366,-1.38734538738263,-34.8184482761359));
#31584=CARTESIAN_POINT('Ctrl Pts',(3.03517161476951,-1.51603900686257,-34.8259464623072));
#31585=CARTESIAN_POINT('Ctrl Pts',(2.89397856132622,-1.77133848810336,-34.8414679968559));
#31586=CARTESIAN_POINT('Ctrl Pts',(2.81306310590148,-1.89721369027721,-34.8494831617403));
#31587=CARTESIAN_POINT('Ctrl Pts',(2.7016094239725,-2.0477162012003,-34.8600356287492));
#31588=CARTESIAN_POINT('Ctrl Pts',(2.67859808864502,-2.07772643857734,-34.8621919721336));
#31589=CARTESIAN_POINT('Ctrl Pts',(2.64229922340208,-2.12346020036185,-34.8655703170097));
#31590=CARTESIAN_POINT('Ctrl Pts',(2.62936178248234,-2.13945903877328,-34.8667700653561));
#31591=CARTESIAN_POINT('Ctrl Pts',(2.6048886661817,-2.1691659810227,-34.8690336274041));
#31592=CARTESIAN_POINT('Ctrl Pts',(2.59338873263631,-2.18290193153236,-34.8700950808327));
#31593=CARTESIAN_POINT('Ctrl Pts',(2.56521653358994,-2.21601503265293,-34.8726892958089));
#31594=CARTESIAN_POINT('Ctrl Pts',(2.54843315455329,-2.23529569848921,-34.8742295695073));
#31595=CARTESIAN_POINT('Ctrl Pts',(2.48488437643595,-2.30665422771724,-34.8800364518458));
#31596=CARTESIAN_POINT('Ctrl Pts',(2.43673010987006,-2.35746667650125,-34.8843864222713));
#31597=CARTESIAN_POINT('Ctrl Pts',(2.29844416648062,-2.49462027990646,-34.8966572761193));
#31598=CARTESIAN_POINT('Ctrl Pts',(2.20506598488657,-2.57752934795268,-34.9046953315908));
#31599=CARTESIAN_POINT('Ctrl Pts',(1.92872128571085,-2.7968623166099,-34.9274196290776));
#31600=CARTESIAN_POINT('Ctrl Pts',(1.73623457465289,-2.92026059402176,-34.9420035506775));
#31601=CARTESIAN_POINT('Ctrl Pts',(1.48259538617798,-3.04884948356767,-34.9593387994373));
#31602=CARTESIAN_POINT('Ctrl Pts',(1.43177182244399,-3.07304446174398,-34.9627288631305));
#31603=CARTESIAN_POINT('Ctrl Pts',(1.34914788102612,-3.10988318747088,-34.968109859079));
#31604=CARTESIAN_POINT('Ctrl Pts',(1.31771919912988,-3.12332990318589,-34.9701272002548));
#31605=CARTESIAN_POINT('Ctrl Pts',(1.25677293888865,-3.14832192936303,-34.9739843424391));
#31606=CARTESIAN_POINT('Ctrl Pts',(1.22728642329919,-3.15993312038952,-34.9758261619595));
#31607=CARTESIAN_POINT('Ctrl Pts',(1.15754195820792,-3.18627351746299,-34.980127961157));
#31608=CARTESIAN_POINT('Ctrl Pts',(1.11715841451135,-3.20065612383089,-34.9825764855907));
#31609=CARTESIAN_POINT('Ctrl Pts',(0.973288417892133,-3.24884054868211,
-34.9911618952961));
#31610=CARTESIAN_POINT('Ctrl Pts',(0.868454568037573,-3.27842109829037,
-34.9971660981783));
#31611=CARTESIAN_POINT('Ctrl Pts',(0.606095365092284,-3.33897841490783,
-35.0117682317079));
#31612=CARTESIAN_POINT('Ctrl Pts',(0.447452281209644,-3.36391391680284,
-35.0202244245797));
#31613=CARTESIAN_POINT('Ctrl Pts',(0.118544636904989,-3.39192463404747,
-35.0377696114158));
#31614=CARTESIAN_POINT('Ctrl Pts',(-0.0513757646744192,-3.39360483469187,
-35.0468449935368));
#31615=CARTESIAN_POINT('Ctrl Pts',(-0.252244515554937,-3.38049965355785,
-35.0582757641332));
#31616=CARTESIAN_POINT('Ctrl Pts',(-0.283770878104262,-3.37799928072184,
-35.0600907254119));
#31617=CARTESIAN_POINT('Ctrl Pts',(-0.334240136233976,-3.37328506345338,
-35.0630362274157));
#31618=CARTESIAN_POINT('Ctrl Pts',(-0.35320804733597,-3.37135175042932,
-35.0641523236043));
#31619=CARTESIAN_POINT('Ctrl Pts',(-0.390739298204573,-3.36720616167878,
-35.0663804760888));
#31620=CARTESIAN_POINT('Ctrl Pts',(-0.409302557241863,-3.36500013460346,
-35.0674921892218));
#31621=CARTESIAN_POINT('Ctrl Pts',(-0.457465896708807,-3.35887206601575,
-35.0704000266512));
#31622=CARTESIAN_POINT('Ctrl Pts',(-0.487033599472257,-3.35471231893777,
-35.0722082031989));
#31623=CARTESIAN_POINT('Ctrl Pts',(-0.634443566264481,-3.33198406586412,
-35.0813254680643));
#31624=CARTESIAN_POINT('Ctrl Pts',(-0.75129431770149,-3.30759556292489,
-35.0888785579196));
#31625=CARTESIAN_POINT('Ctrl Pts',(-1.1131567996652,-3.2119037072286,-35.1128495592457));
#31626=CARTESIAN_POINT('Ctrl Pts',(-1.3515992252719,-3.11907870056493,-35.1294288132987));
#31627=CARTESIAN_POINT('Ctrl Pts',(-1.6480641028837,-2.96321896690237,-35.1501657119898));
#31628=CARTESIAN_POINT('Ctrl Pts',(-1.71741537342769,-2.92357109233622,
-35.1550342867275));
#31629=CARTESIAN_POINT('Ctrl Pts',(-1.818116873072,-2.86117911333031,-35.1621309962846));
#31630=CARTESIAN_POINT('Ctrl Pts',(-1.85057918786169,-2.84029078366784,
-35.1644232613473));
#31631=CARTESIAN_POINT('Ctrl Pts',(-1.90865493207414,-2.80150266354938,
-35.1685342756865));
#31632=CARTESIAN_POINT('Ctrl Pts',(-1.9343907301161,-2.78379478822542,-35.1703597491713));
#31633=CARTESIAN_POINT('Ctrl Pts',(-1.98974337551054,-2.74457029965302,
-35.1742958737963));
#31634=CARTESIAN_POINT('Ctrl Pts',(-2.01926406716062,-2.72292445838318,
-35.1764013914196));
#31635=CARTESIAN_POINT('Ctrl Pts',(-2.10317144685449,-2.65928477105043,
-35.1824093302879));
#31636=CARTESIAN_POINT('Ctrl Pts',(-2.1566409619468,-2.61610899317284,-35.1862664841598));
#31637=CARTESIAN_POINT('Ctrl Pts',(-2.27780629553214,-2.51202860981317,
-35.1951125434662));
#31638=CARTESIAN_POINT('Ctrl Pts',(-2.34443480454401,-2.44996247710945,
-35.2000580986521));
#31639=CARTESIAN_POINT('Ctrl Pts',(-2.50427398751017,-2.2885686365677,-35.2122632748618));
#31640=CARTESIAN_POINT('Ctrl Pts',(-2.59414900486868,-2.18616699521902,
-35.2194410224671));
#31641=CARTESIAN_POINT('Ctrl Pts',(-2.76923251318593,-1.96063116302429,
-35.2346316477654));
#31642=CARTESIAN_POINT('Ctrl Pts',(-2.85293268298594,-1.83670636187101,
-35.2426419561871));
#31643=CARTESIAN_POINT('Ctrl Pts',(-2.94722773916401,-1.67501741597873,
-35.2531887617117));
#31644=CARTESIAN_POINT('Ctrl Pts',(-2.96572714265961,-1.64204048653617,
-35.2553447916394));
#31645=CARTESIAN_POINT('Ctrl Pts',(-2.993434702066,-1.59065302421324,-35.2587227481022));
#31646=CARTESIAN_POINT('Ctrl Pts',(-3.00303377971475,-1.57245554154213,
-35.2599224294812));
#31647=CARTESIAN_POINT('Ctrl Pts',(-3.02068045963614,-1.53825082117741,
-35.2621859450144));
#31648=CARTESIAN_POINT('Ctrl Pts',(-3.02876772364012,-1.52226543320539,
-35.2632474203345));
#31649=CARTESIAN_POINT('Ctrl Pts',(-3.0480871732751,-1.48331493392726,-35.2658418009273));
#31650=CARTESIAN_POINT('Ctrl Pts',(-3.05918682996894,-1.46028574675723,
-35.2673822207929));
#31651=CARTESIAN_POINT('Ctrl Pts',(-3.09970711482363,-1.37372578036355,
-35.2731904068348));
#31652=CARTESIAN_POINT('Ctrl Pts',(-3.12741613132221,-1.3094173233164,-35.2775415810053));
#31653=CARTESIAN_POINT('Ctrl Pts',(-3.19893862914404,-1.12817635351619,
-35.2898173422398));
#31654=CARTESIAN_POINT('Ctrl Pts',(-3.23831293849903,-1.00961238079984,
-35.2978591966103));
#31655=CARTESIAN_POINT('Ctrl Pts',(-3.3316208885491,-0.666346559360019,
-35.3207711574687));
#31656=CARTESIAN_POINT('Ctrl Pts',(-3.36927060381493,-0.437904382366628,
-35.3355340534069));
#31657=CARTESIAN_POINT('Ctrl Pts',(-3.38592720710908,-0.166156663714583,
-35.3521105615618));
#31658=CARTESIAN_POINT('Ctrl Pts',(-3.38770051919659,-0.124885959207531,
-35.3546035224054));
#31659=CARTESIAN_POINT('Ctrl Pts',(-3.3894016571878,-0.0559236771259651,
-35.3587290930678));
#31660=CARTESIAN_POINT('Ctrl Pts',(-3.38974529532265,-0.0282478036078279,
-35.3603740052445));
#31661=CARTESIAN_POINT('Ctrl Pts',(-3.38974995202214,-0.000570320900454691,
-35.3620086083019));
#31662=CARTESIAN_POINT('',(-3.38974881917027,-0.00282938752709428,-37.858982196792));
#31663=CARTESIAN_POINT('Ctrl Pts',(-3.38974995218624,-0.000569344707213824,
-35.3620086659549));
#31664=CARTESIAN_POINT('Ctrl Pts',(-3.38975291771051,0.0170867178207382,
-35.3630514143067));
#31665=CARTESIAN_POINT('Ctrl Pts',(-3.38961793660862,0.0347428412226555,
-35.3640899355741));
#31666=CARTESIAN_POINT('Ctrl Pts',(-3.38899648935759,0.0749413677413,-35.3664450366862));
#31667=CARTESIAN_POINT('Ctrl Pts',(-3.38842305138582,0.0974816613336302,
-35.3677589012831));
#31668=CARTESIAN_POINT('Ctrl Pts',(-3.38633786802073,0.156339478828068,
-35.3711730432985));
#31669=CARTESIAN_POINT('Ctrl Pts',(-3.3844667875467,0.192641891672846,-35.3732622228711));
#31670=CARTESIAN_POINT('Ctrl Pts',(-3.37743126570341,0.296588443641161,
-35.3792016301057));
#31671=CARTESIAN_POINT('Ctrl Pts',(-3.3708196476492,0.364118664350168,-35.3830080450371));
#31672=CARTESIAN_POINT('Ctrl Pts',(-3.32893255581873,0.690566233059449,
-35.4012302280557));
#31673=CARTESIAN_POINT('Ctrl Pts',(-3.26583046453775,0.945001076324621,
-35.4148059003865));
#31674=CARTESIAN_POINT('Ctrl Pts',(-3.12885695894632,1.31045759471189,-35.4357052014358));
#31675=CARTESIAN_POINT('Ctrl Pts',(-3.07673056159079,1.42855442965356,-35.4427134383941));
#31676=CARTESIAN_POINT('Ctrl Pts',(-3.00418794873899,1.57040798658966,-35.4517760667065));
#31677=CARTESIAN_POINT('Ctrl Pts',(-2.99000526293708,1.5972460261098,-35.4535205171969));
#31678=CARTESIAN_POINT('Ctrl Pts',(-2.96645955391385,1.64038901469365,-35.4563792159617));
#31679=CARTESIAN_POINT('Ctrl Pts',(-2.95731761825868,1.65681347058994,-35.4574805068459));
#31680=CARTESIAN_POINT('Ctrl Pts',(-2.93868551465495,1.68964246526695,-35.4597096638239));
#31681=CARTESIAN_POINT('Ctrl Pts',(-2.92919345198542,1.70604510416031,-35.4608376098902));
#31682=CARTESIAN_POINT('Ctrl Pts',(-2.90377139414472,1.74913774743499,-35.4638367621322));
#31683=CARTESIAN_POINT('Ctrl Pts',(-2.88761131132333,1.77568914379793,-35.4657213726169));
#31684=CARTESIAN_POINT('Ctrl Pts',(-2.79371509358002,1.925290908049,-35.4765340046787));
#31685=CARTESIAN_POINT('Ctrl Pts',(-2.70848803534926,2.04344666711543,-35.4858225056777));
#31686=CARTESIAN_POINT('Ctrl Pts',(-2.49671376131709,2.30042887305412,-35.5072343596712));
#31687=CARTESIAN_POINT('Ctrl Pts',(-2.36567915252082,2.43497930434765,-35.5193545716203));
#31688=CARTESIAN_POINT('Ctrl Pts',(-2.14312537729774,2.62848944785032,-35.5378597078768));
#31689=CARTESIAN_POINT('Ctrl Pts',(-2.05875642223739,2.69508233904294,-35.5444785533682));
#31690=CARTESIAN_POINT('Ctrl Pts',(-1.9366388379265,2.7823832883132,-35.5535160555926));
#31691=CARTESIAN_POINT('Ctrl Pts',(-1.90145082295967,2.80654801625459,-35.5560614154846));
#31692=CARTESIAN_POINT('Ctrl Pts',(-1.83938084509652,2.84747003974829,-35.5604522228099));
#31693=CARTESIAN_POINT('Ctrl Pts',(-1.81270361429481,2.86452670223781,-35.5623084719832));
#31694=CARTESIAN_POINT('Ctrl Pts',(-1.75667504342926,2.89925356448393,-35.5661449399777));
#31695=CARTESIAN_POINT('Ctrl Pts',(-1.727286855693,2.9168576723787,-35.5681226397859));
#31696=CARTESIAN_POINT('Ctrl Pts',(-1.64860768004616,2.96238186472672,-35.573329987948));
#31697=CARTESIAN_POINT('Ctrl Pts',(-1.59887414346704,2.98951761661171,-35.5765321555945));
#31698=CARTESIAN_POINT('Ctrl Pts',(-1.35146687251281,3.1165675104746,-35.592069603623));
#31699=CARTESIAN_POINT('Ctrl Pts',(-1.14500893308432,3.19819016642658,-35.6037865171123));
#31700=CARTESIAN_POINT('Ctrl Pts',(-0.80807874034587,3.2945469530148,-35.6223880282357));
#31701=CARTESIAN_POINT('Ctrl Pts',(-0.682192001087079,3.32289654697456,
-35.6292418622242));
#31702=CARTESIAN_POINT('Ctrl Pts',(-0.484632845259992,3.35568541660366,
-35.6402306232104));
#31703=CARTESIAN_POINT('Ctrl Pts',(-0.413914906674825,3.36513992153181,
-35.6442103810439));
#31704=CARTESIAN_POINT('Ctrl Pts',(-0.317359659589477,3.37495924121354,
-35.6497687830793));
#31705=CARTESIAN_POINT('Ctrl Pts',(-0.291734908290365,3.3772707458406,-35.6512558174739));
#31706=CARTESIAN_POINT('Ctrl Pts',(-0.248203797306119,3.3806984094119,-35.6538058378971));
#31707=CARTESIAN_POINT('Ctrl Pts',(-0.230310605959728,3.38196449943124,
-35.6548608984204));
#31708=CARTESIAN_POINT('Ctrl Pts',(-0.191955347339183,3.38437263649069,
-35.6571383839676));
#31709=CARTESIAN_POINT('Ctrl Pts',(-0.171492631767347,3.38547119739737,
-35.6583628673194));
#31710=CARTESIAN_POINT('Ctrl Pts',(-0.11363498725822,3.388051461454,-35.6618493321668));
#31711=CARTESIAN_POINT('Ctrl Pts',(-0.0762247436628929,3.38909946117314,
-35.6641322770748));
#31712=CARTESIAN_POINT('Ctrl Pts',(0.101436125963169,3.39113349095388,-35.6750863124207));
#31713=CARTESIAN_POINT('Ctrl Pts',(0.241633038560804,3.38403356193318,-35.6840573052982));
#31714=CARTESIAN_POINT('Ctrl Pts',(0.558759621458789,3.34816433810946,-35.7045910175322));
#31715=CARTESIAN_POINT('Ctrl Pts',(0.734686026237222,3.31400988494271,-35.7161446332566));
#31716=CARTESIAN_POINT('Ctrl Pts',(1.01182980042781,3.23703870454008,-35.7342023409552));
#31717=CARTESIAN_POINT('Ctrl Pts',(1.11510604435908,3.20293012950349,-35.7409028220947));
#31718=CARTESIAN_POINT('Ctrl Pts',(1.25656151834535,3.14853834176111,-35.7500285574717));
#31719=CARTESIAN_POINT('Ctrl Pts',(1.29625586888896,3.13240506833449,-35.752583909069));
#31720=CARTESIAN_POINT('Ctrl Pts',(1.36475676568306,3.10303850566469,-35.7569861124891));
#31721=CARTESIAN_POINT('Ctrl Pts',(1.39370263897547,3.09014595966006,-35.7588439301141));
#31722=CARTESIAN_POINT('Ctrl Pts',(1.45349798159029,3.06250185589898,-35.7626783760108));
#31723=CARTESIAN_POINT('Ctrl Pts',(1.48431365699262,3.04768553008071,-35.764652565434));
#31724=CARTESIAN_POINT('Ctrl Pts',(1.56528243301119,3.0072359024034,-35.7698382555006));
#31725=CARTESIAN_POINT('Ctrl Pts',(1.61503087642678,2.98081409002974,-35.7730227036185));
#31726=CARTESIAN_POINT('Ctrl Pts',(1.90260353620049,2.818767664648,-35.7914679314374));
#31727=CARTESIAN_POINT('Ctrl Pts',(2.12394099874499,2.6559803891965,-35.8057163167276));
#31728=CARTESIAN_POINT('Ctrl Pts',(2.4239696065906,2.37358174640973,-35.8277296163595));
#31729=CARTESIAN_POINT('Ctrl Pts',(2.51874155615987,2.272763182921,-35.8352129235487));
#31730=CARTESIAN_POINT('Ctrl Pts',(2.62673437512369,2.1428058391625,-35.8448191651196));
#31731=CARTESIAN_POINT('Ctrl Pts',(2.64606098020176,2.11889393095564,-35.8465853068881));
#31732=CARTESIAN_POINT('Ctrl Pts',(2.67672589852464,2.07987979841184,-35.8494706819188));
#31733=CARTESIAN_POINT('Ctrl Pts',(2.68826834238122,2.0649394165042,-35.8505765042623));
#31734=CARTESIAN_POINT('Ctrl Pts',(2.71109427013734,2.03487809512877,-35.8528049736035));
#31735=CARTESIAN_POINT('Ctrl Pts',(2.72237751951488,2.01975780900952,-35.8539275708698));
#31736=CARTESIAN_POINT('Ctrl Pts',(2.7516775638514,1.97980226987503,-35.8568968086561));
#31737=CARTESIAN_POINT('Ctrl Pts',(2.76948402349501,1.95481573140963,-35.8587564049866));
#31738=CARTESIAN_POINT('Ctrl Pts',(2.85973313458692,1.82446713598509,-35.8684573417746));
#31739=CARTESIAN_POINT('Ctrl Pts',(2.92650577685155,1.71531694425535,-35.8765766886657));
#31740=CARTESIAN_POINT('Ctrl Pts',(3.08202248402718,1.42547491934944,-35.8976780570107));
#31741=CARTESIAN_POINT('Ctrl Pts',(3.16114815575196,1.24015890195404,-35.9107186135274));
#31742=CARTESIAN_POINT('Ctrl Pts',(3.25776348113121,0.943254337566089,-35.9303398133329));
#31743=CARTESIAN_POINT('Ctrl Pts',(3.28693308231621,0.835958483269102,-35.9371953042471));
#31744=CARTESIAN_POINT('Ctrl Pts',(3.32003938624461,0.685277151700812,-35.9464880584979));
#31745=CARTESIAN_POINT('Ctrl Pts',(3.32849236888023,0.642965867880995,-35.9490619804585));
#31746=CARTESIAN_POINT('Ctrl Pts',(3.34175655011935,0.569275827759441,-35.9534854182481));
#31747=CARTESIAN_POINT('Ctrl Pts',(3.34693888166077,0.537970289131252,-35.9553462056115));
#31748=CARTESIAN_POINT('Ctrl Pts',(3.35677328294944,0.47290505017467,-35.9591771855472));
#31749=CARTESIAN_POINT('Ctrl Pts',(3.36135738442838,0.43913860602872,-35.9611450849676));
#31750=CARTESIAN_POINT('Ctrl Pts',(3.37209591025473,0.349972375166795,-35.9662919184249));
#31751=CARTESIAN_POINT('Ctrl Pts',(3.37739457745438,0.294478943869608,-35.9694445619635));
#31752=CARTESIAN_POINT('Ctrl Pts',(3.40012405595376,-0.0272575366014145,
-35.9874764569558));
#31753=CARTESIAN_POINT('Ctrl Pts',(3.38744161374581,-0.294674942972111,
-36.0013988635261));
#31754=CARTESIAN_POINT('Ctrl Pts',(3.32136563213738,-0.690708506732728,
-36.0228160547917));
#31755=CARTESIAN_POINT('Ctrl Pts',(3.29130146008207,-0.822116934412209,
-36.03007982314));
#31756=CARTESIAN_POINT('Ctrl Pts',(3.24307756610912,-0.987032458026619,
-36.0397730594453));
#31757=CARTESIAN_POINT('Ctrl Pts',(3.23206597784166,-1.0225137907367,-36.0418937634142));
#31758=CARTESIAN_POINT('Ctrl Pts',(3.21416459467101,-1.07701430337186,-36.0452159703073));
#31759=CARTESIAN_POINT('Ctrl Pts',(3.20768363928058,-1.09616580725634,-36.0463958819132));
#31760=CARTESIAN_POINT('Ctrl Pts',(3.19509987967942,-1.13228393278525,-36.0486467893349));
#31761=CARTESIAN_POINT('Ctrl Pts',(3.18903242051825,-1.14926163652814,-36.0497158626368));
#31762=CARTESIAN_POINT('Ctrl Pts',(3.17377481149534,-1.19090355814875,-36.0523641535892));
#31763=CARTESIAN_POINT('Ctrl Pts',(3.16443237271307,-1.21551038823812,-36.0539516705828));
#31764=CARTESIAN_POINT('Ctrl Pts',(3.12893441450875,-1.30582382773512,-36.0598554938788));
#31765=CARTESIAN_POINT('Ctrl Pts',(3.10101240869683,-1.37081257914646,-36.0642554892892));
#31766=CARTESIAN_POINT('Ctrl Pts',(2.96385617729914,-1.6643695609491,-36.084688331463));
#31767=CARTESIAN_POINT('Ctrl Pts',(2.83124558311262,-1.88112471373453,-36.1012865895793));
#31768=CARTESIAN_POINT('Ctrl Pts',(2.6007449782222,-2.17748543488276,-36.1249797342027));
#31769=CARTESIAN_POINT('Ctrl Pts',(2.52061402688376,-2.26976374271456,-36.1325411133424));
#31770=CARTESIAN_POINT('Ctrl Pts',(2.40478894039566,-2.38942810891008,-36.1425859948302));
#31771=CARTESIAN_POINT('Ctrl Pts',(2.37328357910542,-2.42072341824658,-36.1452379737754));
#31772=CARTESIAN_POINT('Ctrl Pts',(2.31808235183769,-2.47344266355873,-36.1497512631183));
#31773=CARTESIAN_POINT('Ctrl Pts',(2.294682470455,-2.49516670040847,-36.1516251444605));
#31774=CARTESIAN_POINT('Ctrl Pts',(2.2460070190642,-2.53909214525705,-36.1554450577285));
#31775=CARTESIAN_POINT('Ctrl Pts',(2.22070084121954,-2.56125444710339,-36.1573893683854));
#31776=CARTESIAN_POINT('Ctrl Pts',(2.15427188189128,-2.6177058657963,-36.1623899192092));
#31777=CARTESIAN_POINT('Ctrl Pts',(2.11265841796573,-2.65140456864205,-36.1654226649753));
#31778=CARTESIAN_POINT('Ctrl Pts',(1.86883305616828,-2.83946820692365,-36.1826689239435));
#31779=CARTESIAN_POINT('Ctrl Pts',(1.65055822265646,-2.97166356119366,-36.1960143329014));
#31780=CARTESIAN_POINT('Ctrl Pts',(1.28447274730785,-3.14048663145417,-36.2174625177599));
#31781=CARTESIAN_POINT('Ctrl Pts',(1.1454684806342,-3.19380971652053,-36.2254370029875));
#31782=CARTESIAN_POINT('Ctrl Pts',(0.966464736469511,-3.24928429156306,
-36.2359915812267));
#31783=CARTESIAN_POINT('Ctrl Pts',(0.929310538727336,-3.26010492981414,
-36.2381976070474));
#31784=CARTESIAN_POINT('Ctrl Pts',(0.872173889432924,-3.27568912965052,
-36.2416246885382));
#31785=CARTESIAN_POINT('Ctrl Pts',(0.852318724550081,-3.28091135400362,
-36.2428219461697));
#31786=CARTESIAN_POINT('Ctrl Pts',(0.815039043511313,-3.29035527365504,
-36.2450838105314));
#31787=CARTESIAN_POINT('Ctrl Pts',(0.797626588703601,-3.29461958939148,
-36.2461461109411));
#31788=CARTESIAN_POINT('Ctrl Pts',(0.755218990477658,-3.3046493498504,-36.2487466263342));
#31789=CARTESIAN_POINT('Ctrl Pts',(0.730191005138493,-3.31026948419533,
-36.2502924458802));
#31790=CARTESIAN_POINT('Ctrl Pts',(0.640819120970191,-3.329275469935,-36.2558458677938));
#31791=CARTESIAN_POINT('Ctrl Pts',(0.576155774284394,-3.34107283756328,
-36.2599253220164));
#31792=CARTESIAN_POINT('Ctrl Pts',(0.25541767885469,-3.39000167294133,-36.2803342803101));
#31793=CARTESIAN_POINT('Ctrl Pts',(-0.00398814605230557,-3.39960966097446,
-36.2973052599942));
#31794=CARTESIAN_POINT('Ctrl Pts',(-0.384604737145773,-3.37010576771504,
-36.3214043662639));
#31795=CARTESIAN_POINT('Ctrl Pts',(-0.506636573493728,-3.35393178806398,
-36.3290225551889));
#31796=CARTESIAN_POINT('Ctrl Pts',(-0.671256265252023,-3.3229203853085,
-36.3391273503782));
#31797=CARTESIAN_POINT('Ctrl Pts',(-0.714817114836644,-3.31382281267955,
-36.3417851366238));
#31798=CARTESIAN_POINT('Ctrl Pts',(-0.789320514613876,-3.29672541709016,
-36.346305115707));
#31799=CARTESIAN_POINT('Ctrl Pts',(-0.82035141690064,-3.28914107430005,
-36.3481799778022));
#31800=CARTESIAN_POINT('Ctrl Pts',(-0.883799976141665,-3.27267963660726,
-36.3519991869666));
#31801=CARTESIAN_POINT('Ctrl Pts',(-0.916202161966396,-3.26375674905641,
-36.3539418534187));
#31802=CARTESIAN_POINT('Ctrl Pts',(-0.999720855458628,-3.23941558747661,
-36.3589322959125));
#31803=CARTESIAN_POINT('Ctrl Pts',(-1.05061629678126,-3.223268677506,-36.3619567653099));
#31804=CARTESIAN_POINT('Ctrl Pts',(-1.37392680855188,-3.11222405602653,
-36.381105359474));
#31805=CARTESIAN_POINT('Ctrl Pts',(-1.63365451148497,-2.9840895650487,-36.3960674469637));
#31806=CARTESIAN_POINT('Ctrl Pts',(-1.98230938712216,-2.75276964665447,
-36.4184674235656));
#31807=CARTESIAN_POINT('Ctrl Pts',(-2.08636100829852,-2.67476776392646,
-36.4255245949722));
#31808=CARTESIAN_POINT('Ctrl Pts',(-2.20890389594356,-2.57139508772896,
-36.4346432399871));
#31809=CARTESIAN_POINT('Ctrl Pts',(-2.23187363266353,-2.55148369985361,
-36.4363901063229));
#31810=CARTESIAN_POINT('Ctrl Pts',(-2.26861513026565,-2.51875845071746,
-36.4392517641279));
#31811=CARTESIAN_POINT('Ctrl Pts',(-2.28255396088171,-2.50613370045288,
-36.4403535475563));
#31812=CARTESIAN_POINT('Ctrl Pts',(-2.30862471872654,-2.48212283686028,
-36.4424465385982));
#31813=CARTESIAN_POINT('Ctrl Pts',(-2.32077931911639,-2.47076206773626,
-36.4434358053059));
#31814=CARTESIAN_POINT('Ctrl Pts',(-2.35367410233178,-2.43955880370968,
-36.4461488812855));
#31815=CARTESIAN_POINT('Ctrl Pts',(-2.37424621315771,-2.41954205111799,
-36.4478849414556));
#31816=CARTESIAN_POINT('Ctrl Pts',(-2.46043420647661,-2.33352312116177,
-36.4553175230928));
#31817=CARTESIAN_POINT('Ctrl Pts',(-2.52356710335471,-2.26509889671435,
-36.4611607262966));
#31818=CARTESIAN_POINT('Ctrl Pts',(-2.73333483079591,-2.01808166833021,
-36.4817790773549));
#31819=CARTESIAN_POINT('Ctrl Pts',(-2.86449060378868,-1.82715035841029,
-36.4968538516686));
#31820=CARTESIAN_POINT('Ctrl Pts',(-3.03175149545973,-1.52079335139829,
-36.518847473521));
#31821=CARTESIAN_POINT('Ctrl Pts',(-3.08285550873292,-1.4143324346848,-36.5261445085339));
#31822=CARTESIAN_POINT('Ctrl Pts',(-3.14523174932234,-1.26485329195309,
-36.5359093168795));
#31823=CARTESIAN_POINT('Ctrl Pts',(-3.16136705448322,-1.22396700305792,
-36.5385332802285));
#31824=CARTESIAN_POINT('Ctrl Pts',(-3.18781798111594,-1.15292508678705,
-36.5430142105183));
#31825=CARTESIAN_POINT('Ctrl Pts',(-3.19851163163598,-1.12291726375779,
-36.544883279457));
#31826=CARTESIAN_POINT('Ctrl Pts',(-3.21967195490185,-1.06078221592646,
-36.5487065322976));
#31827=CARTESIAN_POINT('Ctrl Pts',(-3.23008448871297,-1.0286402292572,-36.5506587968162));
#31828=CARTESIAN_POINT('Ctrl Pts',(-3.25597007481545,-0.944463048939245,
-36.5557088521758));
#31829=CARTESIAN_POINT('Ctrl Pts',(-3.27067709468231,-0.892201420740232,
-36.5587822146736));
#31830=CARTESIAN_POINT('Ctrl Pts',(-3.35448665182334,-0.564380297930336,
-36.577721452716));
#31831=CARTESIAN_POINT('Ctrl Pts',(-3.38997308429562,-0.281412539648163,
-36.5924713748989));
#31832=CARTESIAN_POINT('Ctrl Pts',(-3.38964502994714,0.134382255907334,
-36.6147175253541));
#31833=CARTESIAN_POINT('Ctrl Pts',(-3.38186496413727,0.265960181732457,
-36.6218630082191));
#31834=CARTESIAN_POINT('Ctrl Pts',(-3.36284433729166,0.427356445404911,
-36.6311010535003));
#31835=CARTESIAN_POINT('Ctrl Pts',(-3.35881852960865,0.45792304174268,-36.6328719083191));
#31836=CARTESIAN_POINT('Ctrl Pts',(-3.35165350531222,0.507130139371208,
-36.635763094996));
#31837=CARTESIAN_POINT('Ctrl Pts',(-3.34877421887896,0.525807371207814,
-36.636869917773));
#31838=CARTESIAN_POINT('Ctrl Pts',(-3.34271126427504,0.563064651079814,
-36.6390983960983));
#31839=CARTESIAN_POINT('Ctrl Pts',(-3.33952847397364,0.581644161505239,
-36.6402199738387));
#31840=CARTESIAN_POINT('Ctrl Pts',(-3.33077258558937,0.630313817552062,
-36.6431832628485));
#31841=CARTESIAN_POINT('Ctrl Pts',(-3.32494679575552,0.660356107646768,
-36.6450378394294));
#31842=CARTESIAN_POINT('Ctrl Pts',(-3.29130386271036,0.822095951276855,
-36.6551452485449));
#31843=CARTESIAN_POINT('Ctrl Pts',(-3.25606967429916,0.952117015032049,
-36.663707625182));
#31844=CARTESIAN_POINT('Ctrl Pts',(-3.12402600083044,1.34508590943447,-36.6903271700678));
#31845=CARTESIAN_POINT('Ctrl Pts',(-3.0022912561801,1.59846509655454,-36.7084444283449));
#31846=CARTESIAN_POINT('Ctrl Pts',(-2.82095570685706,1.88033213273115,-36.7288563368684));
#31847=CARTESIAN_POINT('Ctrl Pts',(-2.79002312231579,1.9259313421964,-36.7321724237843));
#31848=CARTESIAN_POINT('Ctrl Pts',(-2.73825557165496,1.9983777974681,-36.7374661863661));
#31849=CARTESIAN_POINT('Ctrl Pts',(-2.71810548114049,2.02569990747675,-36.7394687402356));
#31850=CARTESIAN_POINT('Ctrl Pts',(-2.67830055027909,2.07800900967378,-36.7433162078615));
#31851=CARTESIAN_POINT('Ctrl Pts',(-2.658698040425,2.10303117235099,-36.7451628409474));
#31852=CARTESIAN_POINT('Ctrl Pts',(-2.61144485759412,2.16163190433837,-36.7495046618866));
#31853=CARTESIAN_POINT('Ctrl Pts',(-2.58349380022731,2.19496167646852,-36.7519877463303));
#31854=CARTESIAN_POINT('Ctrl Pts',(-2.47996468053917,2.31369489752438,-36.7608954913466));
#31855=CARTESIAN_POINT('Ctrl Pts',(-2.40072807146449,2.39581238245582,-36.7671729056432));
#31856=CARTESIAN_POINT('Ctrl Pts',(-2.16211110744881,2.61935405554379,-36.7848681418337));
#31857=CARTESIAN_POINT('Ctrl Pts',(-1.99336134398793,2.74995419251636,-36.7959601642627));
#31858=CARTESIAN_POINT('Ctrl Pts',(-1.71767262796747,2.92452819447855,-36.8135108449752));
#31859=CARTESIAN_POINT('Ctrl Pts',(-1.61889043833329,2.98034455534081,-36.8197082594451));
#31860=CARTESIAN_POINT('Ctrl Pts',(-1.49058127941906,3.04458194698583,-36.8278728509619));
#31861=CARTESIAN_POINT('Ctrl Pts',(-1.46347798122677,3.05770238063039,-36.8296038041403));
#31862=CARTESIAN_POINT('Ctrl Pts',(-1.41922355361421,3.07840234672147,-36.8324459480174));
#31863=CARTESIAN_POINT('Ctrl Pts',(-1.40217737988125,3.08620399007489,-36.8335444616942));
#31864=CARTESIAN_POINT('Ctrl Pts',(-1.36772187313736,3.101629107635,-36.8357741312093));
#31865=CARTESIAN_POINT('Ctrl Pts',(-1.35031146193354,3.10924832735753,-36.8369054488389));
#31866=CARTESIAN_POINT('Ctrl Pts',(-1.30402269784433,3.12904331381351,-36.8399237918581));
#31867=CARTESIAN_POINT('Ctrl Pts',(-1.27503860891919,3.14096540099801,-36.8418245155952));
#31868=CARTESIAN_POINT('Ctrl Pts',(-1.09878793836135,3.2106215156838,-36.8534296862701));
#31869=CARTESIAN_POINT('Ctrl Pts',(-0.947804513571259,3.25838663270074,
-36.8635590588152));
#31870=CARTESIAN_POINT('Ctrl Pts',(-0.541947128908081,3.3561803098806,-36.8904307750818));
#31871=CARTESIAN_POINT('Ctrl Pts',(-0.283659340571229,3.38780622133096,
-36.9071049852191));
#31872=CARTESIAN_POINT('Ctrl Pts',(0.028601019194524,3.39004160278234,-36.9260883361332));
#31873=CARTESIAN_POINT('Ctrl Pts',(0.0814713242028275,3.3891832317419,-36.9292660798254));
#31874=CARTESIAN_POINT('Ctrl Pts',(0.167776993736235,3.38576110567015,-36.9343962788525));
#31875=CARTESIAN_POINT('Ctrl Pts',(0.20123109377197,3.38393758082886,-36.936370848953));
#31876=CARTESIAN_POINT('Ctrl Pts',(0.266570915737505,3.37940359098133,-36.9402015784962));
#31877=CARTESIAN_POINT('Ctrl Pts',(0.298456049845389,3.37673700073289,-36.9420588707245));
#31878=CARTESIAN_POINT('Ctrl Pts',(0.374908411209628,3.36925181286649,-36.9464855740466));
#31879=CARTESIAN_POINT('Ctrl Pts',(0.419427706690148,3.36399981549961,-36.9490414864963));
#31880=CARTESIAN_POINT('Ctrl Pts',(0.588813788426818,3.34060205154497,-36.958696713878));
#31881=CARTESIAN_POINT('Ctrl Pts',(0.712741471448899,3.31637266219298,-36.9656115015557));
#31882=CARTESIAN_POINT('Ctrl Pts',(1.10739320832131,3.21606192873369,-36.9875518149668));
#31883=CARTESIAN_POINT('Ctrl Pts',(1.37004875909919,3.11324724875624,-37.0019599825599));
#31884=CARTESIAN_POINT('Ctrl Pts',(1.65518564131769,2.95848867263242,-37.0200676992201));
#31885=CARTESIAN_POINT('Ctrl Pts',(1.69298723811098,2.93702036054477,-37.0225246485086));
#31886=CARTESIAN_POINT('Ctrl Pts',(1.74900394862664,2.9037665458636,-37.0262664440408));
#31887=CARTESIAN_POINT('Ctrl Pts',(1.76753702866057,2.89252273379275,-37.02752135839));
#31888=CARTESIAN_POINT('Ctrl Pts',(1.80120748356269,2.87165082565038,-37.0298347818789));
#31889=CARTESIAN_POINT('Ctrl Pts',(1.81637831050721,2.8620790846298,-37.0308898363355));
#31890=CARTESIAN_POINT('Ctrl Pts',(1.84871017616473,2.84131929844363,-37.0331668332758));
#31891=CARTESIAN_POINT('Ctrl Pts',(1.86584607493384,2.83009594343037,-37.0343908267452));
#31892=CARTESIAN_POINT('Ctrl Pts',(1.91486815830668,2.79734962829294,-37.0379397423622));
#31893=CARTESIAN_POINT('Ctrl Pts',(1.94649010216414,2.77543888813075,-37.0402873377969));
#31894=CARTESIAN_POINT('Ctrl Pts',(2.09678807954769,2.66746598535107,-37.0517034879291));
#31895=CARTESIAN_POINT('Ctrl Pts',(2.21016306019687,2.57430920279654,-37.0610971714343));
#31896=CARTESIAN_POINT('Ctrl Pts',(2.50534313806257,2.29785705000134,-37.0871307831423));
#31897=CARTESIAN_POINT('Ctrl Pts',(2.67284807145013,2.10066998830198,-37.1037064956791));
#31898=CARTESIAN_POINT('Ctrl Pts',(2.84592087232235,1.84226950158106,-37.122616509712));
#31899=CARTESIAN_POINT('Ctrl Pts',(2.87442059997411,1.79747857179091,-37.1258074389278));
#31900=CARTESIAN_POINT('Ctrl Pts',(2.9191962781746,1.72331757151225,-37.1309533648295));
#31901=CARTESIAN_POINT('Ctrl Pts',(2.93610788900042,1.69434381020086,-37.1329307312326));
#31902=CARTESIAN_POINT('Ctrl Pts',(2.96829402639579,1.63727152518879,-37.136763263519));
#31903=CARTESIAN_POINT('Ctrl Pts',(2.98360647281516,1.60919855564406,-37.1386196186196));
#31904=CARTESIAN_POINT('Ctrl Pts',(3.01936366127919,1.54137782299547,-37.1430381781634));
#31905=CARTESIAN_POINT('Ctrl Pts',(3.03942424184145,1.5014336657723,-37.1455870244209));
#31906=CARTESIAN_POINT('Ctrl Pts',(3.1125202644816,1.34841362839067,-37.1551639302261));
#31907=CARTESIAN_POINT('Ctrl Pts',(3.16008498417495,1.23282958786549,-37.1620116384824));
#31908=CARTESIAN_POINT('Ctrl Pts',(3.29044171502856,0.858533473587456,-37.1833768406599));
#31909=CARTESIAN_POINT('Ctrl Pts',(3.34859577502072,0.592424749464088,-37.1973250982588));
#31910=CARTESIAN_POINT('Ctrl Pts',(3.37955854481869,0.268210537440614,-37.2153890060495));
#31911=CARTESIAN_POINT('Ctrl Pts',(3.38342059865414,0.214049645652439,-37.2184446951969));
#31912=CARTESIAN_POINT('Ctrl Pts',(3.38700690646354,0.138070557565989,-37.2228128932157));
#31913=CARTESIAN_POINT('Ctrl Pts',(3.38782396716887,0.116309836825469,-37.2240733226089));
#31914=CARTESIAN_POINT('Ctrl Pts',(3.38893230618268,0.0765870004195238,
-37.2263936415217));
#31915=CARTESIAN_POINT('Ctrl Pts',(3.38929056984387,0.0586273664766807,
-37.2274500364975));
#31916=CARTESIAN_POINT('Ctrl Pts',(3.38975124619518,0.0202296472509258,
-37.2297254251249));
#31917=CARTESIAN_POINT('Ctrl Pts',(3.3898115965596,-0.000207515682062414,
-37.2309464411633));
#31918=CARTESIAN_POINT('Ctrl Pts',(3.38945450111496,-0.0588433031554558,
-37.2344757666043));
#31919=CARTESIAN_POINT('Ctrl Pts',(3.38857614958776,-0.0970348709187651,
-37.2368063564077));
#31920=CARTESIAN_POINT('Ctrl Pts',(3.38130764675895,-0.279124357383077,
-37.2480448577335));
#31921=CARTESIAN_POINT('Ctrl Pts',(3.36639553878297,-0.422524148933205,
-37.2572672815859));
#31922=CARTESIAN_POINT('Ctrl Pts',(3.29882244385854,-0.822604964105486,
-37.2833789204256));
#31923=CARTESIAN_POINT('Ctrl Pts',(3.22548223248983,-1.07480909643512,-37.3002134041277));
#31924=CARTESIAN_POINT('Ctrl Pts',(3.10344517744663,-1.36447447444007,-37.3193155616264));
#31925=CARTESIAN_POINT('Ctrl Pts',(3.08193473080824,-1.41238852106913,-37.3224711068088));
#31926=CARTESIAN_POINT('Ctrl Pts',(3.04491767319536,-1.48996634181312,-37.327575689948));
#31927=CARTESIAN_POINT('Ctrl Pts',(3.03007039471902,-1.51993317562204,-37.3295463900245));
#31928=CARTESIAN_POINT('Ctrl Pts',(3.0001286867717,-1.57818257771385,-37.3333764321052));
#31929=CARTESIAN_POINT('Ctrl Pts',(2.9850717517939,-1.60648035308957,-37.3352368012902));
#31930=CARTESIAN_POINT('Ctrl Pts',(2.94786720200301,-1.67407232364282,-37.3396822079954));
#31931=CARTESIAN_POINT('Ctrl Pts',(2.9253320054658,-1.71314684495043,-37.3422534649262));
#31932=CARTESIAN_POINT('Ctrl Pts',(2.83544442130496,-1.86205744407763,-37.3520722221862));
#31933=CARTESIAN_POINT('Ctrl Pts',(2.76262873746929,-1.96847401954336,-37.3591264971512));
#31934=CARTESIAN_POINT('Ctrl Pts',(2.54869887984869,-2.24578541067506,-37.3779814784511));
#31935=CARTESIAN_POINT('Ctrl Pts',(2.39663278900657,-2.40739733275429,-37.3894824164829));
#31936=CARTESIAN_POINT('Ctrl Pts',(2.16219186096096,-2.61216657409743,-37.4063826502896));
#31937=CARTESIAN_POINT('Ctrl Pts',(2.09215842396768,-2.66858736059527,-37.4113477134018));
#31938=CARTESIAN_POINT('Ctrl Pts',(1.99720371625967,-2.739048407721,-37.4180922980394));
#31939=CARTESIAN_POINT('Ctrl Pts',(1.97422573337326,-2.75565627492988,-37.4197253842781));
#31940=CARTESIAN_POINT('Ctrl Pts',(1.9374886271607,-2.78151354779837,-37.4223424989463));
#31941=CARTESIAN_POINT('Ctrl Pts',(1.92386482105408,-2.79095394479073,-37.4233143590809));
#31942=CARTESIAN_POINT('Ctrl Pts',(1.89457615652055,-2.81093270745134,-37.4254077230467));
#31943=CARTESIAN_POINT('Ctrl Pts',(1.87889147060741,-2.82144082029587,-37.4265312048687));
#31944=CARTESIAN_POINT('Ctrl Pts',(1.83739598882599,-2.84874169111144,-37.4295081505959));
#31945=CARTESIAN_POINT('Ctrl Pts',(1.81144327154188,-2.86531435828851,-37.4313747132205));
#31946=CARTESIAN_POINT('Ctrl Pts',(1.66636464947796,-2.95519868299341,-37.4418192660119));
#31947=CARTESIAN_POINT('Ctrl Pts',(1.54302397050206,-3.0214302193212,-37.4507314924348));
#31948=CARTESIAN_POINT('Ctrl Pts',(1.18920684961266,-3.18409735966954,-37.4757566309404));
#31949=CARTESIAN_POINT('Ctrl Pts',(0.951601901919277,-3.26300075000567,
-37.4918994151223));
#31950=CARTESIAN_POINT('Ctrl Pts',(0.646451305857619,-3.32812237777288,
-37.5110946502849));
#31951=CARTESIAN_POINT('Ctrl Pts',(0.585082491678947,-3.33945760328811,
-37.5148851748929));
#31952=CARTESIAN_POINT('Ctrl Pts',(0.485097299231768,-3.35508437577289,
-37.5209494477165));
#31953=CARTESIAN_POINT('Ctrl Pts',(0.446660793380559,-3.36041736702635,
-37.5232543213384));
#31954=CARTESIAN_POINT('Ctrl Pts',(0.377142923058058,-3.3688489471352,-37.5273773248536));
#31955=CARTESIAN_POINT('Ctrl Pts',(0.346094688333628,-3.37218009243607,
-37.5292024057419));
#31956=CARTESIAN_POINT('Ctrl Pts',(0.278774327175527,-3.37846325499104,
-37.5331260413979));
#31957=CARTESIAN_POINT('Ctrl Pts',(0.242491537308451,-3.38126116879864,
-37.5352196616802));
#31958=CARTESIAN_POINT('Ctrl Pts',(0.138639672853667,-3.38758931095215,
-37.5411569896988));
#31959=CARTESIAN_POINT('Ctrl Pts',(0.0709988340015097,-3.38968174063348,
-37.5449570835341));
#31960=CARTESIAN_POINT('Ctrl Pts',(-0.144585117383982,-3.38989399499833,
-37.5569040719003));
#31961=CARTESIAN_POINT('Ctrl Pts',(-0.292365903960096,-3.38035693357025,
-37.5648393572385));
#31962=CARTESIAN_POINT('Ctrl Pts',(-0.633042949054784,-3.33585579927932,
-37.5831120860962));
#31963=CARTESIAN_POINT('Ctrl Pts',(-0.824455675476544,-3.29377280567498,
-37.5933589924194));
#31964=CARTESIAN_POINT('Ctrl Pts',(-1.06912127716108,-3.21730834237275,
-37.6075128512475));
#31965=CARTESIAN_POINT('Ctrl Pts',(-1.12658631302324,-3.19763907741666,
-37.61091853786));
#31966=CARTESIAN_POINT('Ctrl Pts',(-1.20680522870482,-3.16775083396876,
-37.6158282263968));
#31967=CARTESIAN_POINT('Ctrl Pts',(-1.23002490280063,-3.15880719040272,
-37.6172680669754));
#31968=CARTESIAN_POINT('Ctrl Pts',(-1.26969868965705,-3.14302207593275,
-37.6197638466993));
#31969=CARTESIAN_POINT('Ctrl Pts',(-1.28620085178479,-3.13630513316568,
-37.6208127360023));
#31970=CARTESIAN_POINT('Ctrl Pts',(-1.32197039865203,-3.12141590972688,
-37.623110716201));
#31971=CARTESIAN_POINT('Ctrl Pts',(-1.34121534750172,-3.11319520081861,
-37.6243623844137));
#31972=CARTESIAN_POINT('Ctrl Pts',(-1.39767531321073,-3.08845698392812,
-37.6280770738331));
#31973=CARTESIAN_POINT('Ctrl Pts',(-1.43466909143979,-3.07144707079296,
-37.6305659687822));
#31974=CARTESIAN_POINT('Ctrl Pts',(-1.52121557982254,-3.02974793743015,
-37.636504449244));
#31975=CARTESIAN_POINT('Ctrl Pts',(-1.57048714084827,-3.00450311656284,
-37.6399766673075));
#31976=CARTESIAN_POINT('Ctrl Pts',(-1.76205821626018,-2.90034962716536,
-37.6537830714612));
#31977=CARTESIAN_POINT('Ctrl Pts',(-1.89921668415575,-2.81244584686513,
-37.6643368784493));
#31978=CARTESIAN_POINT('Ctrl Pts',(-2.18182813356151,-2.6011894220381,-37.6869842258551));
#31979=CARTESIAN_POINT('Ctrl Pts',(-2.3242943375951,-2.47471899656818,-37.6989877503608));
#31980=CARTESIAN_POINT('Ctrl Pts',(-2.48958259269312,-2.3010518469099,-37.7135210577582));
#31981=CARTESIAN_POINT('Ctrl Pts',(-2.52295880653563,-2.26440728119153,
-37.7164931014224));
#31982=CARTESIAN_POINT('Ctrl Pts',(-2.57711333152257,-2.20226521766441,
-37.7213812921138));
#31983=CARTESIAN_POINT('Ctrl Pts',(-2.59834487820743,-2.17717459548613,
-37.7233156263737));
#31984=CARTESIAN_POINT('Ctrl Pts',(-2.63981483415775,-2.12669613243248,
-37.727131575908));
#31985=CARTESIAN_POINT('Ctrl Pts',(-2.66006006891108,-2.10131847519678,
-37.7290133453237));
#31986=CARTESIAN_POINT('Ctrl Pts',(-2.70896848118451,-2.03817135756529,
-37.7336091891634));
#31987=CARTESIAN_POINT('Ctrl Pts',(-2.7372101902285,-2.00008334806539,-37.73630698418));
#31988=CARTESIAN_POINT('Ctrl Pts',(-2.85547402634553,-1.83338857114872,
-37.7478182860818));
#31989=CARTESIAN_POINT('Ctrl Pts',(-2.93730550228126,-1.69920245896067,
-37.7563325558353));
#31990=CARTESIAN_POINT('Ctrl Pts',(-3.11366602735139,-1.35892806351722,
-37.7768110689235));
#31991=CARTESIAN_POINT('Ctrl Pts',(-3.19740005487362,-1.14813724232075,
-37.7885726330847));
#31992=CARTESIAN_POINT('Ctrl Pts',(-3.27578789840572,-0.873576055458517,
-37.8043542459391));
#31993=CARTESIAN_POINT('Ctrl Pts',(-3.29056750668246,-0.816141003013135,
-37.8076822222157));
#31994=CARTESIAN_POINT('Ctrl Pts',(-3.30883525247797,-0.736555778015129,
-37.8123662693966));
#31995=CARTESIAN_POINT('Ctrl Pts',(-3.31362221438587,-0.714711764245834,
-37.8136593771637));
#31996=CARTESIAN_POINT('Ctrl Pts',(-3.32185796490979,-0.675267603920695,
-37.8160103588926));
#31997=CARTESIAN_POINT('Ctrl Pts',(-3.32538392814486,-0.65768411674763,
-37.8170641235992));
#31998=CARTESIAN_POINT('Ctrl Pts',(-3.33256597997833,-0.620333087254208,
-37.8193159618654));
#31999=CARTESIAN_POINT('Ctrl Pts',(-3.33618597510699,-0.600559943098764,
-37.8205157800357));
#32000=CARTESIAN_POINT('Ctrl Pts',(-3.34333417776632,-0.559454319919173,
-37.8230244000056));
#32001=CARTESIAN_POINT('Ctrl Pts',(-3.3468345659574,-0.538117922550193,
-37.8243345255739));
#32002=CARTESIAN_POINT('Ctrl Pts',(-3.35789266484639,-0.46642741696748,
-37.8287601064496));
#32003=CARTESIAN_POINT('Ctrl Pts',(-3.36451960146333,-0.415938711200474,
-37.8319156636527));
#32004=CARTESIAN_POINT('Ctrl Pts',(-3.38306006936681,-0.244907686121074,
-37.8426953985656));
#32005=CARTESIAN_POINT('Ctrl Pts',(-3.38964942260743,-0.123887546823597,
-37.8504707980399));
#32006=CARTESIAN_POINT('Ctrl Pts',(-3.38974885739846,-0.00278321141980408,
-37.8582646956288));
#32007=CARTESIAN_POINT('Ctrl Pts',(-3.38974881917027,-0.00282938752709428,
-37.858982196792));
#32008=CARTESIAN_POINT('Ctrl Pts',(-3.38983414077145,0.099390189715147,
-37.8649908067786));
#32009=CARTESIAN_POINT('Ctrl Pts',(-3.38529153041335,0.20175593427456,-37.8709994167652));
#32010=CARTESIAN_POINT('Ctrl Pts',(-3.37610800013699,0.303808877274895,
-37.8770080267518));
#32011=CARTESIAN_POINT('Ctrl Pts',(-3.36693292370258,0.405767876070146,
-37.8830111055496));
#32012=CARTESIAN_POINT('Ctrl Pts',(-3.35312545909836,0.507414208856045,
-37.8890141843475));
#32013=CARTESIAN_POINT('Ctrl Pts',(-3.33472467480924,0.608289738297792,
-37.8950172631453));
#32014=CARTESIAN_POINT('Ctrl Pts',(-3.31633295417342,0.709115579595218,
-37.9010173850135));
#32015=CARTESIAN_POINT('Ctrl Pts',(-3.29335248592252,0.809170938964297,
-37.9070175068817));
#32016=CARTESIAN_POINT('Ctrl Pts',(-3.26587398343595,0.908004508147524,
-37.9130176287499));
#32017=CARTESIAN_POINT('Ctrl Pts',(-3.23840142551516,1.00681669615636,-37.9190164525808));
#32018=CARTESIAN_POINT('Ctrl Pts',(-3.20643288476187,1.10440719477424,-37.9250152764118));
#32019=CARTESIAN_POINT('Ctrl Pts',(-3.17010955930962,1.20033763769772,-37.9310141002427));
#32020=CARTESIAN_POINT('Ctrl Pts',(-3.13378405816074,1.2962738266684,-37.9370132833916));
#32021=CARTESIAN_POINT('Ctrl Pts',(-3.09310341155129,1.39054935081851,-37.9430124665404));
#32022=CARTESIAN_POINT('Ctrl Pts',(-3.04825740120946,1.48274471115959,-37.9490116496893));
#32023=CARTESIAN_POINT('Ctrl Pts',(-3.00336872422914,1.57502778646307,-37.9550165404802));
#32024=CARTESIAN_POINT('Ctrl Pts',(-2.95430696324229,1.66522634906806,-37.9610214312712));
#32025=CARTESIAN_POINT('Ctrl Pts',(-2.90130831939265,1.75294469345813,-37.9670263220622));
#32026=CARTESIAN_POINT('Ctrl Pts',(-2.84828370879951,1.84070601554692,-37.973034154956));
#32027=CARTESIAN_POINT('Ctrl Pts',(-2.79131862071423,1.92598433427155,-37.9790419878498));
#32028=CARTESIAN_POINT('Ctrl Pts',(-2.73069194036291,2.00841394870107,-37.9850498207436));
#32029=CARTESIAN_POINT('Ctrl Pts',(-2.66996832526969,2.09097535813164,-37.9910672594368));
#32030=CARTESIAN_POINT('Ctrl Pts',(-2.6055717034346,2.1706786247095,-37.99708469813));
#32031=CARTESIAN_POINT('Ctrl Pts',(-2.53782050305355,2.24719206050151,-38.0031021368232));
#32032=CARTESIAN_POINT('Ctrl Pts',(-2.48520910559784,2.30660766876403,-38.0077749080358));
#32033=CARTESIAN_POINT('Ctrl Pts',(-2.4305756762294,2.36410045382413,-38.0124476792483));
#32034=CARTESIAN_POINT('Ctrl Pts',(-2.37408329179727,2.41953168735379,-38.0171204504608));
#32035=CARTESIAN_POINT('Ctrl Pts',(-2.30038166078931,2.49184890959507,-38.0232166856109));
#32036=CARTESIAN_POINT('Ctrl Pts',(-2.22324734380953,2.56091852646214,-38.0293129207611));
#32037=CARTESIAN_POINT('Ctrl Pts',(-2.1429983172996,2.62639739463606,-38.0354091559112));
#32038=CARTESIAN_POINT('Ctrl Pts',(-2.06285464707167,2.69179029777838,-38.0414973875166));
#32039=CARTESIAN_POINT('Ctrl Pts',(-1.97960472572916,2.75360155518141,-38.0475856191221));
#32040=CARTESIAN_POINT('Ctrl Pts',(-1.89360335282372,2.81152474729901,-38.0536738507275));
#32041=CARTESIAN_POINT('Ctrl Pts',(-1.80769016401156,2.86938854613015,-38.0597558395816));
#32042=CARTESIAN_POINT('Ctrl Pts',(-1.71903148714816,2.92337196890895,-38.0658378284358));
#32043=CARTESIAN_POINT('Ctrl Pts',(-1.62801448641066,2.97320935935178,-38.0719198172899));
#32044=CARTESIAN_POINT('Ctrl Pts',(-1.53706143579025,3.02301173318312,-38.0779975328336));
#32045=CARTESIAN_POINT('Ctrl Pts',(-1.44375373097807,3.06867366194833,-38.0840752483773));
#32046=CARTESIAN_POINT('Ctrl Pts',(-1.34850604205042,3.10997371645702,-38.090152963921));
#32047=CARTESIAN_POINT('Ctrl Pts',(-1.25329301605569,3.15125874087905,-38.0962284676373));
#32048=CARTESIAN_POINT('Ctrl Pts',(-1.15614180181199,3.18818487542941,-38.1023039713536));
#32049=CARTESIAN_POINT('Ctrl Pts',(-1.05748936925174,3.22057778922037,-38.10837947507));
#32050=CARTESIAN_POINT('Ctrl Pts',(-0.958847159831589,3.25296734620311,
-38.1144543491949));
#32051=CARTESIAN_POINT('Ctrl Pts',(-0.85870444862362,3.28082448284244,-38.1205292233197));
#32052=CARTESIAN_POINT('Ctrl Pts',(-0.757514895782916,3.30402425008761,
-38.1266040974446));
#32053=CARTESIAN_POINT('Ctrl Pts',(-0.656309489974358,3.32722765194875,
-38.1326799232961));
#32054=CARTESIAN_POINT('Ctrl Pts',(-0.554057334471316,3.34577213901651,
-38.1387557491475));
#32055=CARTESIAN_POINT('Ctrl Pts',(-0.451222937461346,3.35958374255037,
-38.144831574999));
#32056=CARTESIAN_POINT('Ctrl Pts',(-0.348280532879214,3.37340985249268,
-38.1509137823261));
#32057=CARTESIAN_POINT('Ctrl Pts',(-0.244755091134823,3.38249309473644,
-38.1569959896531));
#32058=CARTESIAN_POINT('Ctrl Pts',(-0.141116870459519,3.3868113457014,-38.1630781969802));
#32059=CARTESIAN_POINT('Ctrl Pts',(-0.037421959047741,3.39113195877587,
-38.1691637313117));
#32060=CARTESIAN_POINT('Ctrl Pts',(0.0663854255811521,3.39068239103628,
-38.1752492656431));
#32061=CARTESIAN_POINT('Ctrl Pts',(0.169836408984024,3.385492675621,-38.1813347999746));
#32062=CARTESIAN_POINT('Ctrl Pts',(0.273456962562488,3.38029445355913,-38.1874303093211));
#32063=CARTESIAN_POINT('Ctrl Pts',(0.376719521140766,3.37034060431963,-38.1935258186677));
#32064=CARTESIAN_POINT('Ctrl Pts',(0.479161483580033,3.35571293992102,-38.1996213280143));
#32065=CARTESIAN_POINT('Ctrl Pts',(0.558010455492585,3.34445411324639,-38.2043130054658));
#32066=CARTESIAN_POINT('Ctrl Pts',(0.636373404964492,3.33042744792137,-38.2090046829173));
#32067=CARTESIAN_POINT('Ctrl Pts',(0.714045197901123,3.31369046802117,-38.2136963603687));
#32068=CARTESIAN_POINT('Ctrl Pts',(0.815268669115325,3.29187849305461,-38.2198106505055));
#32069=CARTESIAN_POINT('Ctrl Pts',(0.915658892897034,3.26538818141388,-38.2259249406422));
#32070=CARTESIAN_POINT('Ctrl Pts',(1.01475235199809,3.23429787227682,-38.232039230779));
#32071=CARTESIAN_POINT('Ctrl Pts',(1.11371593249673,3.2032483122057,-38.2381455071127));
#32072=CARTESIAN_POINT('Ctrl Pts',(1.21138572463981,3.16761086832305,-38.2442517834465));
#32073=CARTESIAN_POINT('Ctrl Pts',(1.30730876727621,3.12751480404214,-38.2503580597803));
#32074=CARTESIAN_POINT('Ctrl Pts',(1.40313321354815,3.08745995328051,-38.2564580596592));
#32075=CARTESIAN_POINT('Ctrl Pts',(1.49721409006694,3.04295575948584,-38.2625580595381));
#32076=CARTESIAN_POINT('Ctrl Pts',(1.58911477883168,2.99418090338556,-38.268658059417));
#32077=CARTESIAN_POINT('Ctrl Pts',(1.68094922156511,2.94544120633237,-38.2747536621495));
#32078=CARTESIAN_POINT('Ctrl Pts',(1.77060622723507,2.89243716882074,-38.280849264882));
#32079=CARTESIAN_POINT('Ctrl Pts',(1.85767106192568,2.83539473234044,-38.2869448676145));
#32080=CARTESIAN_POINT('Ctrl Pts',(1.94470312654783,2.77837376588941,-38.2930381760416));
#32081=CARTESIAN_POINT('Ctrl Pts',(2.0291446037669,2.71731765488788,-38.2991314844687));
#32082=CARTESIAN_POINT('Ctrl Pts',(2.11060785557143,2.65249685061079,-38.3052247928958));
#32083=CARTESIAN_POINT('Ctrl Pts',(2.19206130727747,2.5876838443316,-38.3113173682928));
#32084=CARTESIAN_POINT('Ctrl Pts',(2.2705369129707,2.51910731061273,-38.3174099436897));
#32085=CARTESIAN_POINT('Ctrl Pts',(2.34567909139088,2.44707880190067,-38.3235025190866));
#32086=CARTESIAN_POINT('Ctrl Pts',(2.42083147251851,2.3750405132512,-38.3295959217255));
#32087=CARTESIAN_POINT('Ctrl Pts',(2.49264921977449,2.29954961309818,-38.3356893243644));
#32088=CARTESIAN_POINT('Ctrl Pts',(2.56081333099779,2.22095478258429,-38.3417827270033));
#32089=CARTESIAN_POINT('Ctrl Pts',(2.62904547735814,2.14228150595014,-38.3478822115155));
#32090=CARTESIAN_POINT('Ctrl Pts',(2.69361642534844,2.06049843411023,-38.3539816960276));
#32091=CARTESIAN_POINT('Ctrl Pts',(2.75424727785984,1.9759875998856,-38.3600811805398));
#32092=CARTESIAN_POINT('Ctrl Pts',(2.81490979888174,1.89143262423578,-38.3661838509149));
#32093=CARTESIAN_POINT('Ctrl Pts',(2.87162789227152,1.80414740479087,-38.3722865212901));
#32094=CARTESIAN_POINT('Ctrl Pts',(2.92416691291382,1.71454160868731,-38.3783891916652));
#32095=CARTESIAN_POINT('Ctrl Pts',(2.97678832966248,1.62479528524586,-38.3845014327607));
#32096=CARTESIAN_POINT('Ctrl Pts',(3.02521738248743,1.53272149199777,-38.3906136738563));
#32097=CARTESIAN_POINT('Ctrl Pts',(3.06926606901717,1.43875323112751,-38.3967259149518));
#32098=CARTESIAN_POINT('Ctrl Pts',(3.10180727880631,1.36933366084283,-38.4012413667267));
#32099=CARTESIAN_POINT('Ctrl Pts',(3.13195884762922,1.2988806412099,-38.4057568185016));
#32100=CARTESIAN_POINT('Ctrl Pts',(3.15966238818469,1.2275742972183,-38.4102722702765));
#32101=CARTESIAN_POINT('Ctrl Pts',(3.1971479686723,1.13108988968846,-38.4163821149949));
#32102=CARTESIAN_POINT('Ctrl Pts',(3.23027140246842,1.03272916962564,-38.4224919597134));
#32103=CARTESIAN_POINT('Ctrl Pts',(3.25884355599605,0.932922151116077,-38.4286018044318));
#32104=CARTESIAN_POINT('Ctrl Pts',(3.28737891648419,0.833243656470446,-38.4347037813584));
#32105=CARTESIAN_POINT('Ctrl Pts',(3.31137453285367,0.732122972853293,-38.440805758285));
#32106=CARTESIAN_POINT('Ctrl Pts',(3.33068962614992,0.630009267199531,-38.4469077352115));
#32107=CARTESIAN_POINT('Ctrl Pts',(3.34998532524936,0.5279980934505,-38.453003585171));
#32108=CARTESIAN_POINT('Ctrl Pts',(3.36460976864686,0.424996297323794,-38.4590994351304));
#32109=CARTESIAN_POINT('Ctrl Pts',(3.37447245260414,0.321466528764371,-38.4651952850899));
#32110=CARTESIAN_POINT('Ctrl Pts',(3.38432840853305,0.218007385120252,-38.4712869766426));
#32111=CARTESIAN_POINT('Ctrl Pts',(3.38942902447563,0.114021408496264,-38.4773786681953));
#32112=CARTESIAN_POINT('Ctrl Pts',(3.38973531170907,0.00997893043375072,
-38.483470359748));
#32113=CARTESIAN_POINT('Ctrl Pts',(3.39004149101343,-0.0940268852787506,
-38.4895599047185));
#32114=CARTESIAN_POINT('Ctrl Pts',(3.38555669829589,-0.19808873698997,-38.4956494496891));
#32115=CARTESIAN_POINT('Ctrl Pts',(3.37629402602813,-0.301734506324266,
-38.5017389946596));
#32116=CARTESIAN_POINT('Ctrl Pts',(3.36703223868343,-0.405370373707195,
-38.5078279578565));
#32117=CARTESIAN_POINT('Ctrl Pts',(3.35299351755496,-0.508589813170739,
-38.5139169210534));
#32118=CARTESIAN_POINT('Ctrl Pts',(3.33424290886367,-0.610924943992602,
-38.5200058842503));
#32119=CARTESIAN_POINT('Ctrl Pts',(3.31548927569185,-0.713276581511107,
-38.5260958295993));
#32120=CARTESIAN_POINT('Ctrl Pts',(3.29202232159112,-0.814743207624254,
-38.5321857749483));
#32121=CARTESIAN_POINT('Ctrl Pts',(3.26395820546061,-0.914867146369542,
-38.5382757202974));
#32122=CARTESIAN_POINT('Ctrl Pts',(3.23586487097873,-1.01509532700183,-38.5443720060621));
#32123=CARTESIAN_POINT('Ctrl Pts',(3.20316493152196,-1.11397761737651,-38.5504682918269));
#32124=CARTESIAN_POINT('Ctrl Pts',(3.16602444086707,-1.21107155128522,-38.5565645775916));
#32125=CARTESIAN_POINT('Ctrl Pts',(3.12886369340613,-1.30821844122526,-38.5626641883334));
#32126=CARTESIAN_POINT('Ctrl Pts',(3.08725774069385,-1.40357464094468,-38.5687637990752));
#32127=CARTESIAN_POINT('Ctrl Pts',(3.04142001497191,-1.49671953118421,-38.574863409817));
#32128=CARTESIAN_POINT('Ctrl Pts',(2.99550844485433,-1.59001447747511,-38.5809728470076));
#32129=CARTESIAN_POINT('Ctrl Pts',(2.94535168890258,-1.68109062429625,-38.5870822841983));
#32130=CARTESIAN_POINT('Ctrl Pts',(2.89120828233017,-1.76955353993187,-38.593191721389));
#32131=CARTESIAN_POINT('Ctrl Pts',(2.85086593011768,-1.83546742171807,-38.5977438743207));
#32132=CARTESIAN_POINT('Ctrl Pts',(2.80831121941705,-1.89993105791082,-38.6022960272525));
#32133=CARTESIAN_POINT('Ctrl Pts',(2.76366569239595,-1.96279316362515,-38.6068481801843));
#32134=CARTESIAN_POINT('Ctrl Pts',(2.70438964570048,-2.04625543548805,-38.6128920920329));
#32135=CARTESIAN_POINT('Ctrl Pts',(2.64121868490761,-2.12718573413482,-38.6189360038816));
#32136=CARTESIAN_POINT('Ctrl Pts',(2.57439814735876,-2.20519369701978,-38.6249799157302));
#32137=CARTESIAN_POINT('Ctrl Pts',(2.50766623068107,-2.28309820168843,-38.6310158118286));
#32138=CARTESIAN_POINT('Ctrl Pts',(2.43729463655874,-2.35808774356995,-38.6370517079271));
#32139=CARTESIAN_POINT('Ctrl Pts',(2.36357170776567,-2.42980119449095,-38.6430876040255));
#32140=CARTESIAN_POINT('Ctrl Pts',(2.28992444284467,-2.50144104392237,-38.6491173053176));
#32141=CARTESIAN_POINT('Ctrl Pts',(2.21293299079736,-2.56981118262046,-38.6551470066097));
#32142=CARTESIAN_POINT('Ctrl Pts',(2.1329250015896,-2.63458459725513,-38.6611767079018));
#32143=CARTESIAN_POINT('Ctrl Pts',(2.05297011955903,-2.6993150170184,-38.6672024068384));
#32144=CARTESIAN_POINT('Ctrl Pts',(1.97000301736443,-2.76045318269514,-38.6732281057749));
#32145=CARTESIAN_POINT('Ctrl Pts',(1.8843864639987,-2.81771054524741,-38.6792538047115));
#32146=CARTESIAN_POINT('Ctrl Pts',(1.79879887582025,-2.87494853689343,-38.6852774650762));
#32147=CARTESIAN_POINT('Ctrl Pts',(1.71056397940562,-2.92830809062396,-38.6913011254409));
#32148=CARTESIAN_POINT('Ctrl Pts',(1.62007495157907,-2.97754298268993,-38.6973247858056));
#32149=CARTESIAN_POINT('Ctrl Pts',(1.52959198350284,-3.02677457765835,-38.7033480427858));
#32150=CARTESIAN_POINT('Ctrl Pts',(1.43685556758776,-3.07188185110027,-38.7093712997659));
#32151=CARTESIAN_POINT('Ctrl Pts',(1.34228408306178,-3.11266421299488,-38.715394556746));
#32152=CARTESIAN_POINT('Ctrl Pts',(1.24769326879543,-3.15345491051487,-38.7214190448372));
#32153=CARTESIAN_POINT('Ctrl Pts',(1.15126704190743,-3.18991876770193,-38.7274435329283));
#32154=CARTESIAN_POINT('Ctrl Pts',(1.05344341489572,-3.22190347994983,-38.7334680210194));
#32155=CARTESIAN_POINT('Ctrl Pts',(0.955504118820467,-3.25392601170848,
-38.7394996326135));
#32156=CARTESIAN_POINT('Ctrl Pts',(0.856164539250224,-3.28145868734966,
-38.7455312442075));
#32157=CARTESIAN_POINT('Ctrl Pts',(0.755877434432334,-3.304399244434,-38.7515628558016));
#32158=CARTESIAN_POINT('Ctrl Pts',(0.655529636183558,-3.32735368506916,
-38.7575981177075));
#32159=CARTESIAN_POINT('Ctrl Pts',(0.554233600829645,-3.34571039835397,
-38.7636333796133));
#32160=CARTESIAN_POINT('Ctrl Pts',(0.452449651290486,-3.35941875561043,
-38.7696686415192));
#32161=CARTESIAN_POINT('Ctrl Pts',(0.350479551375543,-3.37315218377312,
-38.7757149411798));
#32162=CARTESIAN_POINT('Ctrl Pts',(0.248020189943388,-3.38222023803654,
-38.7817612408404));
#32163=CARTESIAN_POINT('Ctrl Pts',(0.145534609622456,-3.38662438718882,
-38.787807540501));
#32164=CARTESIAN_POINT('Ctrl Pts',(0.0573004147538147,-3.390416106505,-38.7930130570314));
#32165=CARTESIAN_POINT('Ctrl Pts',(-0.0309530534813594,-3.39075170782255,
-38.7982185735618));
#32166=CARTESIAN_POINT('Ctrl Pts',(-0.118933916524157,-3.38766287962664,
-38.8034240900922));
#32167=CARTESIAN_POINT('Ctrl Pts',(-0.224849347785803,-3.38394440541362,
-38.8096907316002));
#32168=CARTESIAN_POINT('Ctrl Pts',(-0.330736464059233,-3.37524930895149,
-38.8159573731083));
#32169=CARTESIAN_POINT('Ctrl Pts',(-0.43610525559405,-3.36157957938575,
-38.8222240146163));
#32170=CARTESIAN_POINT('Ctrl Pts',(-0.541321542207547,-3.34792963462537,
-38.8284815861364));
#32171=CARTESIAN_POINT('Ctrl Pts',(-0.646020603782136,-3.32931943810331,
-38.8347391576565));
#32172=CARTESIAN_POINT('Ctrl Pts',(-0.749714638658902,-3.30580293167644,
-38.8409967291765));
#32173=CARTESIAN_POINT('Ctrl Pts',(-0.85328208895224,-3.28231513304529,
-38.8472466617607));
#32174=CARTESIAN_POINT('Ctrl Pts',(-0.955846567181931,-3.25393303523451,
-38.8534965943449));
#32175=CARTESIAN_POINT('Ctrl Pts',(-1.05692811526889,-3.22076202499566,
-38.8597465269291));
#32176=CARTESIAN_POINT('Ctrl Pts',(-1.1578921628135,-3.18762957383874,-38.8659891943845));
#32177=CARTESIAN_POINT('Ctrl Pts',(-1.2573763363218,-3.14971942491507,-38.8722318618399));
#32178=CARTESIAN_POINT('Ctrl Pts',(-1.35491429957384,-3.10718720120149,
-38.8784745292952));
#32179=CARTESIAN_POINT('Ctrl Pts',(-1.45238591808696,-3.06468390765195,
-38.8847129505256));
#32180=CARTESIAN_POINT('Ctrl Pts',(-1.54791359598286,-3.01756495602677,
-38.8909513717559));
#32181=CARTESIAN_POINT('Ctrl Pts',(-1.64104963928406,-2.96603458238532,
-38.8971897929862));
#32182=CARTESIAN_POINT('Ctrl Pts',(-1.73414143229932,-2.91452869157229,
-38.9034252502521));
#32183=CARTESIAN_POINT('Ctrl Pts',(-1.82484350394313,-2.85861574463121,
-38.9096607075179));
#32184=CARTESIAN_POINT('Ctrl Pts',(-1.91273200068808,-2.79854629335371,
-38.9158961647838));
#32185=CARTESIAN_POINT('Ctrl Pts',(-2.00059675223758,-2.73849307128611,
-38.9221299373906));
#32186=CARTESIAN_POINT('Ctrl Pts',(-2.08564911350769,-2.67428580704603,
-38.9283637099974));
#32187=CARTESIAN_POINT('Ctrl Pts',(-2.16749398185336,-2.6062185060216,-38.9345974826042));
#32188=CARTESIAN_POINT('Ctrl Pts',(-2.2493552757425,-2.53813754448999,-38.9408325062742));
#32189=CARTESIAN_POINT('Ctrl Pts',(-2.32800748004704,-2.46619525002732,
-38.9470675299442));
#32190=CARTESIAN_POINT('Ctrl Pts',(-2.40308851994954,-2.39072596250318,
-38.9533025536142));
#32191=CARTESIAN_POINT('Ctrl Pts',(-2.47817601732117,-2.31525018411803,
-38.9595381135377));
#32192=CARTESIAN_POINT('Ctrl Pts',(-2.54969146119573,-2.23624709626379,
-38.9657736734613));
#32193=CARTESIAN_POINT('Ctrl Pts',(-2.61731033495177,-2.15408720182231,
-38.9720092333848));
#32194=CARTESIAN_POINT('Ctrl Pts',(-2.68497354999018,-2.07187343077986,
-38.9782488822957));
#32195=CARTESIAN_POINT('Ctrl Pts',(-2.74873484185292,-1.98649903094724,
-38.9844885312067));
#32196=CARTESIAN_POINT('Ctrl Pts',(-2.80831063467403,-1.89836678270475,
-38.9907281801176));
#32197=CARTESIAN_POINT('Ctrl Pts',(-2.83781956101856,-1.85471334732747,
-38.9938187867451));
#32198=CARTESIAN_POINT('Ctrl Pts',(-2.86630228420872,-1.81038376008177,
-38.9969093933725));
#32199=CARTESIAN_POINT('Ctrl Pts',(-2.89372837779135,-1.76542944862293,
-39.));
#32200=CARTESIAN_POINT('Origin',(0.,0.,-25.2396150285955));
#32201=CARTESIAN_POINT('',(-4.08499846294095,-0.00354369441070796,-29.6146150285489));
#32202=CARTESIAN_POINT('Ctrl Pts',(2.48705727606859,3.24064362520075,-28.807442179994));
#32203=CARTESIAN_POINT('Ctrl Pts',(2.58164700590404,3.16804999781167,-28.8132572105571));
#32204=CARTESIAN_POINT('Ctrl Pts',(2.67316058774221,3.09123106367021,-28.8190722411201));
#32205=CARTESIAN_POINT('Ctrl Pts',(2.76120186744336,3.01047990314291,-28.8248872716832));
#32206=CARTESIAN_POINT('Ctrl Pts',(2.84917143199732,2.92979451950324,-28.8306975655389));
#32207=CARTESIAN_POINT('Ctrl Pts',(2.93367402287073,2.84518355732362,-28.8365078593947));
#32208=CARTESIAN_POINT('Ctrl Pts',(3.01434615521614,2.75698064130557,-28.8423181532505));
#32209=CARTESIAN_POINT('Ctrl Pts',(3.09498008804593,2.66881949074692,-28.8481256958413));
#32210=CARTESIAN_POINT('Ctrl Pts',(3.17178689450958,2.57707006898604,-28.853933238432));
#32211=CARTESIAN_POINT('Ctrl Pts',(3.24443994965179,2.48210282081615,-28.8597407810228));
#32212=CARTESIAN_POINT('Ctrl Pts',(3.31707661506872,2.38715699620656,-28.8655470134963));
#32213=CARTESIAN_POINT('Ctrl Pts',(3.38556114487292,2.28899511246094,-28.8713532459698));
#32214=CARTESIAN_POINT('Ctrl Pts',(3.44960762164253,2.18802016825845,-28.8771594784432));
#32215=CARTESIAN_POINT('Ctrl Pts',(3.51365472080847,2.08704424279302,-28.882965767341));
#32216=CARTESIAN_POINT('Ctrl Pts',(3.57326346288696,1.98325554704796,-28.8887720562387));
#32217=CARTESIAN_POINT('Ctrl Pts',(3.62819198975171,1.87708494360312,-28.8945783451365));
#32218=CARTESIAN_POINT('Ctrl Pts',(3.68313397534118,1.77088832597209,-28.9003860567056));
#32219=CARTESIAN_POINT('Ctrl Pts',(3.73339327778706,1.66230900215408,-28.9061937682748));
#32220=CARTESIAN_POINT('Ctrl Pts',(3.77877489615272,1.55180065865626,-28.9120014798439));
#32221=CARTESIAN_POINT('Ctrl Pts',(3.82420481518244,1.44117469867477,-28.9178153726895));
#32222=CARTESIAN_POINT('Ctrl Pts',(3.86474652885717,1.32861599717976,-28.923629265535));
#32223=CARTESIAN_POINT('Ctrl Pts',(3.90025385988548,1.21459657024397,-28.9294431583805));
#32224=CARTESIAN_POINT('Ctrl Pts',(3.93578195114944,1.10051047904186,-28.9352604504617));
#32225=CARTESIAN_POINT('Ctrl Pts',(3.96626969242796,0.984962355085262,-28.9410777425429));
#32226=CARTESIAN_POINT('Ctrl Pts',(3.99162171258813,0.868436010074988,-28.946895034624));
#32227=CARTESIAN_POINT('Ctrl Pts',(4.01701207075936,0.751733450771981,-28.9527211237717));
#32228=CARTESIAN_POINT('Ctrl Pts',(4.03725112819439,0.634050117542279,-28.9585472129194));
#32229=CARTESIAN_POINT('Ctrl Pts',(4.05229515063293,0.515876935089047,-28.9643733020672));
#32230=CARTESIAN_POINT('Ctrl Pts',(4.06112216126169,0.446539366509142,-28.967791732945));
#32231=CARTESIAN_POINT('Ctrl Pts',(4.06816166086629,0.377033218991992,-28.9712101638229));
#32232=CARTESIAN_POINT('Ctrl Pts',(4.07341316753139,0.307457585012765,-28.9746285947007));
#32233=CARTESIAN_POINT('Ctrl Pts',(4.08236103870315,0.188909928265574,-28.9804531477395));
#32234=CARTESIAN_POINT('Ctrl Pts',(4.08614387469233,0.0697810997494614,
-28.9862777007783));
#32235=CARTESIAN_POINT('Ctrl Pts',(4.0847007864651,-0.0494417339034575,
-28.9921022538172));
#32236=CARTESIAN_POINT('Ctrl Pts',(4.08325951286277,-0.168514649680232,
-28.9979194827168));
#32237=CARTESIAN_POINT('Ctrl Pts',(4.07660539043645,-0.287680930906462,
-29.0037367116165));
#32238=CARTESIAN_POINT('Ctrl Pts',(4.06472931976189,-0.406448713945576,
-29.0095539405162));
#32239=CARTESIAN_POINT('Ctrl Pts',(4.05286509059105,-0.525098074891956,
-29.0153653691189));
#32240=CARTESIAN_POINT('Ctrl Pts',(4.03578931186541,-0.64334932428627,-29.0211767977215));
#32241=CARTESIAN_POINT('Ctrl Pts',(4.01354491966947,-0.760711625910505,
-29.0269882263242));
#32242=CARTESIAN_POINT('Ctrl Pts',(3.99054423949725,-0.882064133102252,
-29.0329972379194));
#32243=CARTESIAN_POINT('Ctrl Pts',(3.96201723460135,-1.00246572457672,-29.0390062495145));
#32244=CARTESIAN_POINT('Ctrl Pts',(3.92806967614734,-1.12138022959733,-29.0450152611097));
#32245=CARTESIAN_POINT('Ctrl Pts',(3.89527504687168,-1.23625615249857,-29.050820194264));
#32246=CARTESIAN_POINT('Ctrl Pts',(3.85742219141108,-1.34974393339543,-29.0566251274183));
#32247=CARTESIAN_POINT('Ctrl Pts',(3.81465806888086,-1.46137223783749,-29.0624300605726));
#32248=CARTESIAN_POINT('Ctrl Pts',(3.77190019058608,-1.57298424278892,-29.0682341461152));
#32249=CARTESIAN_POINT('Ctrl Pts',(3.724232617372,-1.68273693020281,-29.0740382316579));
#32250=CARTESIAN_POINT('Ctrl Pts',(3.67185123912532,-1.79017694034246,-29.0798423172005));
#32251=CARTESIAN_POINT('Ctrl Pts',(3.61946516013535,-1.89762659222739,-29.085646923606));
#32252=CARTESIAN_POINT('Ctrl Pts',(3.56236461393751,-2.00276278730165,-29.0914515300115));
#32253=CARTESIAN_POINT('Ctrl Pts',(3.50079213651266,-2.10515543771265,-29.0972561364171));
#32254=CARTESIAN_POINT('Ctrl Pts',(3.43919961752166,-2.20758141647362,-29.103062632196));
#32255=CARTESIAN_POINT('Ctrl Pts',(3.37313248268168,-2.30726172496065,-29.108869127975));
#32256=CARTESIAN_POINT('Ctrl Pts',(3.30287704283458,-2.40379455027178,-29.1146756237539));
#32257=CARTESIAN_POINT('Ctrl Pts',(3.23254417097476,-2.50043376920843,-29.1204885191605));
#32258=CARTESIAN_POINT('Ctrl Pts',(3.15801402041512,-2.59391825050628,-29.1263014145671));
#32259=CARTESIAN_POINT('Ctrl Pts',(3.0796137970976,-2.68387851079853,-29.1321143099737));
#32260=CARTESIAN_POINT('Ctrl Pts',(3.0011620114909,-2.77389793618952,-29.1379310284076));
#32261=CARTESIAN_POINT('Ctrl Pts',(2.91883536487427,-2.86038822961364,-29.1437477468415));
#32262=CARTESIAN_POINT('Ctrl Pts',(2.83299741639933,-2.94301726781796,-29.1495644652754));
#32263=CARTESIAN_POINT('Ctrl Pts',(2.74703775313504,-3.02576347070479,-29.1553894315842));
#32264=CARTESIAN_POINT('Ctrl Pts',(2.65755715590551,-3.10463722190456,-29.1612143978929));
#32265=CARTESIAN_POINT('Ctrl Pts',(2.56495174898386,-3.17934702814661,-29.1670393642017));
#32266=CARTESIAN_POINT('Ctrl Pts',(2.54287925952979,-3.19715410297312,-29.1684277443373));
#32267=CARTESIAN_POINT('Ctrl Pts',(2.5206293729239,-3.21472481756346,-29.169816124473));
#32268=CARTESIAN_POINT('Ctrl Pts',(2.49820767935441,-3.23205559834831,-29.1712045046086));
#32269=CARTESIAN_POINT('Ctrl Pts',(2.40412529591361,-3.30477629440437,-29.1770302069301));
#32270=CARTESIAN_POINT('Ctrl Pts',(2.30671462318317,-3.37350184690707,-29.1828559092517));
#32271=CARTESIAN_POINT('Ctrl Pts',(2.20634918628449,-3.43791335960954,-29.1886816115732));
#32272=CARTESIAN_POINT('Ctrl Pts',(2.1061096874175,-3.50224404907865,-29.1945000038336));
#32273=CARTESIAN_POINT('Ctrl Pts',(2.00292313929499,-3.5622712473514,-29.2003183960939));
#32274=CARTESIAN_POINT('Ctrl Pts',(1.89719547046546,-3.61771673115037,-29.2061367883543));
#32275=CARTESIAN_POINT('Ctrl Pts',(1.79157297222626,-3.67310706160749,-29.2119493928795));
#32276=CARTESIAN_POINT('Ctrl Pts',(1.68341474126908,-3.72392455612287,-29.2177619974047));
#32277=CARTESIAN_POINT('Ctrl Pts',(1.57315446568604,-3.76993501629565,-29.2235746019299));
#32278=CARTESIAN_POINT('Ctrl Pts',(1.45917678316605,-3.81749671151581,-29.2295831774543));
#32279=CARTESIAN_POINT('Ctrl Pts',(1.34295318503273,-3.85992126840636,-29.2355917529787));
#32280=CARTESIAN_POINT('Ctrl Pts',(1.22498937260595,-3.89700218591195,-29.2416003285032));
#32281=CARTESIAN_POINT('Ctrl Pts',(1.11100003196341,-3.93283376213796,-29.2474064613175));
#32282=CARTESIAN_POINT('Ctrl Pts',(0.995386272004685,-3.96367584593016,
-29.2532125941318));
#32283=CARTESIAN_POINT('Ctrl Pts',(0.878622705452774,-3.98939182601344,
-29.2590187269461));
#32284=CARTESIAN_POINT('Ctrl Pts',(0.761876050015233,-4.01510408159692,
-29.2648240188459));
#32285=CARTESIAN_POINT('Ctrl Pts',(0.643980317493258,-4.0356916222519,-29.2706293107457));
#32286=CARTESIAN_POINT('Ctrl Pts',(0.525422027187254,-4.05106858660113,
-29.2764346026455));
#32287=CARTESIAN_POINT('Ctrl Pts',(0.406852989532603,-4.06644694487731,
-29.2822404207969));
#32288=CARTESIAN_POINT('Ctrl Pts',(0.287621679281552,-4.07661373524268,
-29.2880462389484));
#32289=CARTESIAN_POINT('Ctrl Pts',(0.168220844391062,-4.08153485192916,
-29.2938520570999));
#32290=CARTESIAN_POINT('Ctrl Pts',(0.0487810691944442,-4.08645757354403,
-29.2996597687082));
#32291=CARTESIAN_POINT('Ctrl Pts',(-0.0708279331831924,-4.08613120229194,
-29.3054674803166));
#32292=CARTESIAN_POINT('Ctrl Pts',(-0.190112941066558,-4.08057374270323,
-29.311275191925));
#32293=CARTESIAN_POINT('Ctrl Pts',(-0.309529390787627,-4.07501015927117,
-29.3170893031329));
#32294=CARTESIAN_POINT('Ctrl Pts',(-0.428620725640996,-4.06420400086641,
-29.3229034143409));
#32295=CARTESIAN_POINT('Ctrl Pts',(-0.546898218435627,-4.04822520849223,
-29.3287175255488));
#32296=CARTESIAN_POINT('Ctrl Pts',(-0.665253511881017,-4.03223590557698,
-29.3345354611668));
#32297=CARTESIAN_POINT('Ctrl Pts',(-0.78279349654856,-4.0110672646297,-29.3403533967849));
#32298=CARTESIAN_POINT('Ctrl Pts',(-0.899040636338648,-3.98484013910368,
-29.3461713324029));
#32299=CARTESIAN_POINT('Ctrl Pts',(-1.01545243297985,-3.95857586448382,
-29.3519975087653));
#32300=CARTESIAN_POINT('Ctrl Pts',(-1.13056733763087,-3.92723891158967,
-29.3578236851276));
#32301=CARTESIAN_POINT('Ctrl Pts',(-1.24392381923684,-3.89099968284954,
-29.36364986149));
#32302=CARTESIAN_POINT('Ctrl Pts',(-1.27071239828836,-3.88243557226568,
-29.3650267124988));
#32303=CARTESIAN_POINT('Ctrl Pts',(-1.29740286653171,-3.87359788932101,
-29.3664035635076));
#32304=CARTESIAN_POINT('Ctrl Pts',(-1.32398931486147,-3.86448926691906,
-29.3677804145163));
#32305=CARTESIAN_POINT('Ctrl Pts',(-1.43647825555107,-3.82595011071335,
-29.3736059580242));
#32306=CARTESIAN_POINT('Ctrl Pts',(-1.54746295502343,-3.78243370292111,
-29.3794315015321));
#32307=CARTESIAN_POINT('Ctrl Pts',(-1.65647161659419,-3.73407642977722,
-29.38525704504));
#32308=CARTESIAN_POINT('Ctrl Pts',(-1.76534349629072,-3.68577983436626,
-29.3910752787732));
#32309=CARTESIAN_POINT('Ctrl Pts',(-1.87224390013117,-3.63265461935452,
-29.3968935125064));
#32310=CARTESIAN_POINT('Ctrl Pts',(-1.97671716030412,-3.57488660913311,
-29.4027117462395));
#32311=CARTESIAN_POINT('Ctrl Pts',(-2.08108650355432,-3.51717605929769,
-29.408524192722));
#32312=CARTESIAN_POINT('Ctrl Pts',(-2.18303315099799,-3.45483209784832,
-29.4143366392045));
#32313=CARTESIAN_POINT('Ctrl Pts',(-2.2821229182699,-3.38808795427558,-29.420149085687));
#32314=CARTESIAN_POINT('Ctrl Pts',(-2.38455727880139,-3.31909098461538,
-29.4261577206344));
#32315=CARTESIAN_POINT('Ctrl Pts',(-2.48393808422484,-3.24539171838284,
-29.4321663555818));
#32316=CARTESIAN_POINT('Ctrl Pts',(-2.57981460119327,-3.16729878973709,
-29.4381749905292));
#32317=CARTESIAN_POINT('Ctrl Pts',(-2.67245741625451,-3.09183976207444,
-29.4439809675692));
#32318=CARTESIAN_POINT('Ctrl Pts',(-2.76182817335498,-3.01227894803338,
-29.4497869446093));
#32319=CARTESIAN_POINT('Ctrl Pts',(-2.84755165172228,-2.92893745081279,
-29.4555929216494));
#32320=CARTESIAN_POINT('Ctrl Pts',(-2.93326273082004,-2.84560800832572,
-29.4613980588977));
#32321=CARTESIAN_POINT('Ctrl Pts',(-3.01532728789925,-2.75849925454101,
-29.4672031961459));
#32322=CARTESIAN_POINT('Ctrl Pts',(-3.09340592558045,-2.66797016092455,
-29.4730083333942));
#32323=CARTESIAN_POINT('Ctrl Pts',(-3.17149165880314,-2.57743284030824,
-29.4788139981951));
#32324=CARTESIAN_POINT('Ctrl Pts',(-3.2455904859473,-2.48347487083025,-29.484619662996));
#32325=CARTESIAN_POINT('Ctrl Pts',(-3.31540279742206,-2.38648890440455,
-29.490425327797));
#32326=CARTESIAN_POINT('Ctrl Pts',(-3.38523789525339,-2.28947128228993,
-29.4962328875351));
#32327=CARTESIAN_POINT('Ctrl Pts',(-3.45078345666214,-2.18942402861275,
-29.5020404472733));
#32328=CARTESIAN_POINT('Ctrl Pts',(-3.51178312296444,-2.08676886531837,
-29.5078480070114));
#32329=CARTESIAN_POINT('Ctrl Pts',(-3.57285003860565,-1.98400052940707,
-29.5136619693183));
#32330=CARTESIAN_POINT('Ctrl Pts',(-3.62936084713854,-1.8786188959865,-29.5194759316251));
#32331=CARTESIAN_POINT('Ctrl Pts',(-3.68110502949018,-1.77107051295597,
-29.525289893932));
#32332=CARTESIAN_POINT('Ctrl Pts',(-3.7328832629757,-1.66345135589397,-29.531107682215));
#32333=CARTESIAN_POINT('Ctrl Pts',(-3.7798884630376,-1.55366298372032,-29.536925470498));
#32334=CARTESIAN_POINT('Ctrl Pts',(-3.82195878033918,-1.44217061452112,
-29.542743258781));
#32335=CARTESIAN_POINT('Ctrl Pts',(-3.8640887137464,-1.33052025409946,-29.548569291211));
#32336=CARTESIAN_POINT('Ctrl Pts',(-3.90126968056075,-1.2171614635597,-29.5543953236411));
#32337=CARTESIAN_POINT('Ctrl Pts',(-3.93339001154322,-1.10257336131979,
-29.5602213560711));
#32338=CARTESIAN_POINT('Ctrl Pts',(-3.94098903962392,-1.07546410746093,
-29.5615996788555));
#32339=CARTESIAN_POINT('Ctrl Pts',(-3.94830505004656,-1.04828608618615,
-29.5629780016398));
#32340=CARTESIAN_POINT('Ctrl Pts',(-3.95533698646056,-1.0210457010032,-29.5643563244242));
#32341=CARTESIAN_POINT('Ctrl Pts',(-3.9935929449067,-0.872849388883327,
-29.5718548363646));
#32342=CARTESIAN_POINT('Ctrl Pts',(-4.02353545220108,-0.722426523062194,
-29.579353348305));
#32343=CARTESIAN_POINT('Ctrl Pts',(-4.0449536888374,-0.570591495871375,
-29.5868518602454));
#32344=CARTESIAN_POINT('Ctrl Pts',(-4.06597312067764,-0.421583617249565,
-29.5942107508633));
#32345=CARTESIAN_POINT('Ctrl Pts',(-4.07878279064484,-0.271215465179849,
-29.6015696414811));
#32346=CARTESIAN_POINT('Ctrl Pts',(-4.08322889380424,-0.120278014625242,
-29.608928532099));
#32347=CARTESIAN_POINT('Ctrl Pts',(-4.08437411850112,-0.0813996328464814,
-29.6108240309156));
#32348=CARTESIAN_POINT('Ctrl Pts',(-4.08496468297067,-0.0424836002528471,
-29.6127195297322));
#32349=CARTESIAN_POINT('Ctrl Pts',(-4.08499846294095,-0.00354369441070524,
-29.6146150285489));
#32350=CARTESIAN_POINT('Ctrl Pts',(-4.08499846294178,-0.00354369345236866,
-29.6146150285955));
#32351=CARTESIAN_POINT('Ctrl Pts',(-4.08510089553568,0.114535647855257,
-29.620362840432));
#32352=CARTESIAN_POINT('Ctrl Pts',(-4.08007936315259,0.232738167103182,
-29.6261106522686));
#32353=CARTESIAN_POINT('Ctrl Pts',(-4.069928608205,0.350579697236656,-29.6318584641051));
#32354=CARTESIAN_POINT('Ctrl Pts',(-4.0597836237934,0.46835423641281,-29.6376030084059));
#32355=CARTESIAN_POINT('Ctrl Pts',(-4.0445152498184,0.585767779234244,-29.6433475527066));
#32356=CARTESIAN_POINT('Ctrl Pts',(-4.02417029374906,0.702337843852654,
-29.6490920970074));
#32357=CARTESIAN_POINT('Ctrl Pts',(-4.00383097033797,0.818875635148233,
-29.6548350508867));
#32358=CARTESIAN_POINT('Ctrl Pts',(-3.9784179301521,0.934570001073691,-29.660578004766));
#32359=CARTESIAN_POINT('Ctrl Pts',(-3.94802955510798,1.04894596238026,-29.6663209586452));
#32360=CARTESIAN_POINT('Ctrl Pts',(-3.9176420426122,1.16331867722185,-29.6720637495156));
#32361=CARTESIAN_POINT('Ctrl Pts',(-3.88227958379287,1.27637265809959,-29.677806540386));
#32362=CARTESIAN_POINT('Ctrl Pts',(-3.84209096551582,1.38764621308952,-29.6835493312564));
#32363=CARTESIAN_POINT('Ctrl Pts',(-3.80189350162445,1.49894425966425,-29.6892933861293));
#32364=CARTESIAN_POINT('Ctrl Pts',(-3.75686790934974,1.60846070870447,-29.6950374410022));
#32365=CARTESIAN_POINT('Ctrl Pts',(-3.70721154631942,1.71575276506726,-29.7007814958751));
#32366=CARTESIAN_POINT('Ctrl Pts',(-3.65750360539991,1.82315626531071,-29.7065315170775));
#32367=CARTESIAN_POINT('Ctrl Pts',(-3.60315546790751,1.92833038117625,-29.7122815382799));
#32368=CARTESIAN_POINT('Ctrl Pts',(-3.54441101778661,2.03085586317515,-29.7180315594823));
#32369=CARTESIAN_POINT('Ctrl Pts',(-3.48563213688581,2.1334414365069,-29.7237849508365));
#32370=CARTESIAN_POINT('Ctrl Pts',(-3.42245203699577,2.23337493319784,-29.7295383421908));
#32371=CARTESIAN_POINT('Ctrl Pts',(-3.35515760178694,2.33026660860325,-29.735291733545));
#32372=CARTESIAN_POINT('Ctrl Pts',(-3.28776329517689,2.42730208055529,-29.7410536634842));
#32373=CARTESIAN_POINT('Ctrl Pts',(-3.21624271703737,2.52128638831926,-29.7468155934235));
#32374=CARTESIAN_POINT('Ctrl Pts',(-3.14092271218498,2.6118632269092,-29.7525775233627));
#32375=CARTESIAN_POINT('Ctrl Pts',(-3.10451842418982,2.65564157403201,-29.7553624270191));
#32376=CARTESIAN_POINT('Ctrl Pts',(-3.06722711650288,2.6986244687061,-29.7581473306756));
#32377=CARTESIAN_POINT('Ctrl Pts',(-3.02908860636657,2.74077492961028,-29.760932234332));
#32378=CARTESIAN_POINT('Ctrl Pts',(-2.9493100423512,2.82894573731889,-29.7667577270908));
#32379=CARTESIAN_POINT('Ctrl Pts',(-2.86555096101358,2.91377138955036,-29.7725832198497));
#32380=CARTESIAN_POINT('Ctrl Pts',(-2.77812274705242,2.99487211785577,-29.7784087126085));
#32381=CARTESIAN_POINT('Ctrl Pts',(-2.69080426352897,3.07587105729907,-29.7842268938389));
#32382=CARTESIAN_POINT('Ctrl Pts',(-2.59982610353627,3.15315409665027,-29.7900450750693));
#32383=CARTESIAN_POINT('Ctrl Pts',(-2.50553872285622,3.22637578534616,-29.7958632562998));
#32384=CARTESIAN_POINT('Ctrl Pts',(-2.41134515554145,3.2995246204642,-29.801675648599));
#32385=CARTESIAN_POINT('Ctrl Pts',(-2.3138492382938,3.36861989519583,-29.8074880408982));
#32386=CARTESIAN_POINT('Ctrl Pts',(-2.21343651800874,3.43335459583558,-29.8133004331974));
#32387=CARTESIAN_POINT('Ctrl Pts',(-2.10963324299415,3.50027514050781,-29.8193090878242));
#32388=CARTESIAN_POINT('Ctrl Pts',(-2.00271302621213,3.56253511807048,-29.8253177424509));
#32389=CARTESIAN_POINT('Ctrl Pts',(-1.89313725188156,3.61984203322995,-29.8313263970777));
#32390=CARTESIAN_POINT('Ctrl Pts',(-1.78725863023146,3.67521537852613,-29.8371323160752));
#32391=CARTESIAN_POINT('Ctrl Pts',(-1.67890115085158,3.72596430412592,-29.8429382350727));
#32392=CARTESIAN_POINT('Ctrl Pts',(-1.56850786000158,3.77187063578714,-29.8487441540703));
#32393=CARTESIAN_POINT('Ctrl Pts',(-1.45813056223032,3.81777031683063,-29.8545492319431));
#32394=CARTESIAN_POINT('Ctrl Pts',(-1.34571841617986,3.85882864255651,-29.860354309816));
#32395=CARTESIAN_POINT('Ctrl Pts',(-1.23173513987145,3.8948752926385,-29.8661593876888));
#32396=CARTESIAN_POINT('Ctrl Pts',(-1.11774153001839,3.93092521065313,-29.8719649918409));
#32397=CARTESIAN_POINT('Ctrl Pts',(-1.00217689574656,3.96196242663428,-29.877770595993));
#32398=CARTESIAN_POINT('Ctrl Pts',(-0.885520214903857,3.98786646579303,
-29.8835762001451));
#32399=CARTESIAN_POINT('Ctrl Pts',(-0.768825481972242,4.01377895455617,
-29.8893836980196));
#32400=CARTESIAN_POINT('Ctrl Pts',(-0.651038392130681,4.03455484808431,
-29.895191195894));
#32401=CARTESIAN_POINT('Ctrl Pts',(-0.532647580448056,4.05012488141327,
-29.9009986937685));
#32402=CARTESIAN_POINT('Ctrl Pts',(-0.414126277472672,4.0657120761566,-29.9068125927132));
#32403=CARTESIAN_POINT('Ctrl Pts',(-0.295000329181403,4.07608190427893,
-29.9126264916579));
#32404=CARTESIAN_POINT('Ctrl Pts',(-0.175763106651671,4.08121701583488,
-29.9184403906027));
#32405=CARTESIAN_POINT('Ctrl Pts',(-0.0564474366678613,4.08635550583608,
-29.9242581145742));
#32406=CARTESIAN_POINT('Ctrl Pts',(0.0629792462984349,4.08625242074811,
-29.9300758385457));
#32407=CARTESIAN_POINT('Ctrl Pts',(0.182025608117366,4.08094249873598,-29.9358935625172));
#32408=CARTESIAN_POINT('Ctrl Pts',(0.301240648911888,4.07562505299788,-29.9417195297286));
#32409=CARTESIAN_POINT('Ctrl Pts',(0.420073888093814,4.06508608140495,-29.9475454969401));
#32410=CARTESIAN_POINT('Ctrl Pts',(0.538041007510124,4.04941191708592,-29.9533714641515));
#32411=CARTESIAN_POINT('Ctrl Pts',(0.565961535053325,4.04570214661131,-29.9547503575143));
#32412=CARTESIAN_POINT('Ctrl Pts',(0.593833599717153,4.04170493758397,-29.9561292508771));
#32413=CARTESIAN_POINT('Ctrl Pts',(0.621650892464621,4.0374218466613,-29.9575081442399));
#32414=CARTESIAN_POINT('Ctrl Pts',(0.739170385986166,4.01932710679901,-29.9633335439683));
#32415=CARTESIAN_POINT('Ctrl Pts',(0.856087170397083,3.99606810769409,-29.9691589436968));
#32416=CARTESIAN_POINT('Ctrl Pts',(0.971912817304395,3.96769586480106,-29.9749843434252));
#32417=CARTESIAN_POINT('Ctrl Pts',(1.08759851749451,3.93935790276343,-29.9808027045953));
#32418=CARTESIAN_POINT('Ctrl Pts',(1.20219530906337,3.90591907906435,-29.9866210657655));
#32419=CARTESIAN_POINT('Ctrl Pts',(1.31522185004862,3.86748193081166,-29.9924394269356));
#32420=CARTESIAN_POINT('Ctrl Pts',(1.42812074180017,3.82908819247382,-29.9982512170001));
#32421=CARTESIAN_POINT('Ctrl Pts',(1.53945252905253,3.78570749722147,-30.0040630070645));
#32422=CARTESIAN_POINT('Ctrl Pts',(1.64874884363787,3.73749277599339,-30.009874797129));
#32423=CARTESIAN_POINT('Ctrl Pts',(1.75797285251911,3.68930995153494,-30.0156827423651));
#32424=CARTESIAN_POINT('Ctrl Pts',(1.86516369482128,3.63629962515944,-30.0214906876011));
#32425=CARTESIAN_POINT('Ctrl Pts',(1.96987115601415,3.57866352549433,-30.0272986328372));
#32426=CARTESIAN_POINT('Ctrl Pts',(2.07454021434151,3.52104856464166,-30.0331044479315));
#32427=CARTESIAN_POINT('Ctrl Pts',(2.17672734503127,3.45881139899725,-30.0389102630258));
#32428=CARTESIAN_POINT('Ctrl Pts',(2.27600570578405,3.3922003223923,-30.04471607812));
#32429=CARTESIAN_POINT('Ctrl Pts',(2.34793368652654,3.34394005500928,-30.0489224384299));
#32430=CARTESIAN_POINT('Ctrl Pts',(2.41833528000595,3.29338485814733,-30.0531287987397));
#32431=CARTESIAN_POINT('Ctrl Pts',(2.48705727606859,3.24064362520075,-30.0573351590495));
#32432=CARTESIAN_POINT('',(-4.08499876708699,0.00317378287634478,-29.5103849714406));
#32433=CARTESIAN_POINT('Ctrl Pts',(-4.08499876708699,0.00317378287634033,
-29.5103849714406));
#32434=CARTESIAN_POINT('Ctrl Pts',(-4.08488929600371,0.144074801529089,
-29.5172304279821));
#32435=CARTESIAN_POINT('Ctrl Pts',(-4.07748594560271,0.284674789363894,
-29.5240758845235));
#32436=CARTESIAN_POINT('Ctrl Pts',(-4.06290522156446,0.424294898136044,
-29.530921341065));
#32437=CARTESIAN_POINT('Ctrl Pts',(-4.04810681336837,0.565999477179698,
-29.5378689974313));
#32438=CARTESIAN_POINT('Ctrl Pts',(-4.025915162707,0.706694609343906,-29.5448166537975));
#32439=CARTESIAN_POINT('Ctrl Pts',(-3.99650239142486,0.845691217487437,
-29.5517643101638));
#32440=CARTESIAN_POINT('Ctrl Pts',(-3.96708962014271,0.984687825630963,
-29.5587119665301));
#32441=CARTESIAN_POINT('Ctrl Pts',(-3.93045585216911,1.12198587687786,-29.5656596228963));
#32442=CARTESIAN_POINT('Ctrl Pts',(-3.88682172051456,1.25691762376707,-29.5726072792626));
#32443=CARTESIAN_POINT('Ctrl Pts',(-3.85023392742419,1.37005966760532,-29.5784329804729));
#32444=CARTESIAN_POINT('Ctrl Pts',(-3.80864334589806,1.48178369611155,-29.5842586816833));
#32445=CARTESIAN_POINT('Ctrl Pts',(-3.76217819466759,1.59161560421092,-29.5900843828936));
#32446=CARTESIAN_POINT('Ctrl Pts',(-3.71577134776499,1.70130969557213,-29.5959027740321));
#32447=CARTESIAN_POINT('Ctrl Pts',(-3.66450225477699,1.80911601644211,-29.6017211651706));
#32448=CARTESIAN_POINT('Ctrl Pts',(-3.60854884390259,1.91457573398632,-29.6075395563091));
#32449=CARTESIAN_POINT('Ctrl Pts',(-3.55265109172022,2.01993054729239,-29.6133521597032));
#32450=CARTESIAN_POINT('Ctrl Pts',(-3.49207848178133,2.12294304271336,-29.6191647630973));
#32451=CARTESIAN_POINT('Ctrl Pts',(-3.42705671164646,2.22317504824945,-29.6249773664914));
#32452=CARTESIAN_POINT('Ctrl Pts',(-3.35984272551286,2.32678638667152,-29.6309859424364));
#32453=CARTESIAN_POINT('Ctrl Pts',(-3.28787444324839,2.42742602431081,-29.6369945183813));
#32454=CARTESIAN_POINT('Ctrl Pts',(-3.21145263674161,2.5246379863191,-29.6430030943263));
#32455=CARTESIAN_POINT('Ctrl Pts',(-3.13760567617815,2.61857462891975,-29.6488092259938));
#32456=CARTESIAN_POINT('Ctrl Pts',(-3.05960073089692,2.70931050351429,-29.6546153576614));
#32457=CARTESIAN_POINT('Ctrl Pts',(-2.97775237715265,2.79646487200568,-29.6604214893289));
#32458=CARTESIAN_POINT('Ctrl Pts',(-2.8959158777345,2.88360661768599,-29.6662267800782));
#32459=CARTESIAN_POINT('Ctrl Pts',(-2.81023735611584,2.967167591559,-29.6720320708274));
#32460=CARTESIAN_POINT('Ctrl Pts',(-2.721069871197,3.04680221807454,-29.6778373615767));
#32461=CARTESIAN_POINT('Ctrl Pts',(-2.63189430325336,3.12644406346209,-29.683643178575));
#32462=CARTESIAN_POINT('Ctrl Pts',(-2.53922944748117,3.20215858206116,-29.6894489955734));
#32463=CARTESIAN_POINT('Ctrl Pts',(-2.44346272712173,3.27363939693529,-29.6952548125717));
#32464=CARTESIAN_POINT('Ctrl Pts',(-2.34766477428718,3.34514352390325,-29.7010625230257));
#32465=CARTESIAN_POINT('Ctrl Pts',(-2.24876327173674,3.41241095722145,-29.7068702334797));
#32466=CARTESIAN_POINT('Ctrl Pts',(-2.14717545758527,3.4751780608112,-29.7126779439337));
#32467=CARTESIAN_POINT('Ctrl Pts',(-2.04547570229445,3.53801432841583,-29.7184920539911));
#32468=CARTESIAN_POINT('Ctrl Pts',(-1.94108407419197,3.59634015337465,-29.7243061640485));
#32469=CARTESIAN_POINT('Ctrl Pts',(-1.83444342769416,3.64993730228201,-29.7301202741059));
#32470=CARTESIAN_POINT('Ctrl Pts',(-1.72773263500741,3.7035697063745,-29.7359382085743));
#32471=CARTESIAN_POINT('Ctrl Pts',(-1.61877024903109,3.75246707315416,-29.7417561430428));
#32472=CARTESIAN_POINT('Ctrl Pts',(-1.50801863533895,3.79645950794559,-29.7475740775112));
#32473=CARTESIAN_POINT('Ctrl Pts',(-1.39711014864572,3.84051425537555,-29.7534002527339));
#32474=CARTESIAN_POINT('Ctrl Pts',(-1.28440776002582,3.87965007109166,-29.7592264279567));
#32475=CARTESIAN_POINT('Ctrl Pts',(-1.17038860321449,3.91374699200979,-29.7650526031795));
#32476=CARTESIAN_POINT('Ctrl Pts',(-1.14344319942173,3.9218048949791,-29.7664294651765));
#32477=CARTESIAN_POINT('Ctrl Pts',(-1.11642429684647,3.92958160727636,-29.7678063271735));
#32478=CARTESIAN_POINT('Ctrl Pts',(-1.08933825928154,3.93707596534096,-29.7691831891705));
#32479=CARTESIAN_POINT('Ctrl Pts',(-0.974731543651779,3.96878616885371,
-29.7750089815543));
#32480=CARTESIAN_POINT('Ctrl Pts',(-0.858555805965655,3.99553869464658,
-29.7808347739381));
#32481=CARTESIAN_POINT('Ctrl Pts',(-0.741277505723837,4.01717968972112,
-29.7866605663218));
#32482=CARTESIAN_POINT('Ctrl Pts',(-0.624147580059496,4.03879330570256,
-29.7924789882076));
#32483=CARTESIAN_POINT('Ctrl Pts',(-0.505918264273633,4.05530818077743,
-29.7982974100933));
#32484=CARTESIAN_POINT('Ctrl Pts',(-0.387070608536924,4.0666203835626,-29.804115831979));
#32485=CARTESIAN_POINT('Ctrl Pts',(-0.268342398844149,4.07792121718898,
-29.8099284061476));
#32486=CARTESIAN_POINT('Ctrl Pts',(-0.148997489524003,4.08402974303888,
-29.8157409803162));
#32487=CARTESIAN_POINT('Ctrl Pts',(-0.0295259523632294,4.08489329335994,
-29.8215535544847));
#32488=CARTESIAN_POINT('Ctrl Pts',(0.0898546208102128,4.08575618618565,
-29.8273617030392));
#32489=CARTESIAN_POINT('Ctrl Pts',(0.209361223302048,4.08138204855642,-29.8331698515936));
#32490=CARTESIAN_POINT('Ctrl Pts',(0.328500470335767,4.0717701851884,-29.838978000148));
#32491=CARTESIAN_POINT('Ctrl Pts',(0.447591693800847,4.06216219624456,-29.8447838075091));
#32492=CARTESIAN_POINT('Ctrl Pts',(0.566315450295777,4.04732071319067,-29.8505896148701));
#32493=CARTESIAN_POINT('Ctrl Pts',(0.684180624496516,4.02729709272405,-29.8563954222311));
#32494=CARTESIAN_POINT('Ctrl Pts',(0.802026048285521,4.0072768275721,-29.8622002567256));
#32495=CARTESIAN_POINT('Ctrl Pts',(0.919012774035862,3.9820762212117,-29.8680050912201));
#32496=CARTESIAN_POINT('Ctrl Pts',(1.03465769411707,3.9517981294601,-29.8738099257145));
#32497=CARTESIAN_POINT('Ctrl Pts',(1.15031047185885,3.92151798041998,-29.8796151546268));
#32498=CARTESIAN_POINT('Ctrl Pts',(1.26462086834682,3.8861597644006,-29.8854203835391));
#32499=CARTESIAN_POINT('Ctrl Pts',(1.37711942230712,3.84587663565857,-29.8912256124514));
#32500=CARTESIAN_POINT('Ctrl Pts',(1.48970655940519,3.80556178734489,-29.8970354124926));
#32501=CARTESIAN_POINT('Ctrl Pts',(1.60047862020886,3.7603144193227,-29.9028452125339));
#32502=CARTESIAN_POINT('Ctrl Pts',(1.7089846065242,3.71033645572249,-29.9086550125751));
#32503=CARTESIAN_POINT('Ctrl Pts',(1.81753764560202,3.66033681957378,-29.9144673319901));
#32504=CARTESIAN_POINT('Ctrl Pts',(1.92382228891063,3.60560268585826,-29.9202796514051));
#32505=CARTESIAN_POINT('Ctrl Pts',(2.0274120530472,3.54638201088926,-29.9260919708202));
#32506=CARTESIAN_POINT('Ctrl Pts',(2.13113213206795,3.48708683690518,-29.9319116020747));
#32507=CARTESIAN_POINT('Ctrl Pts',(2.23215021574526,3.42329406624566,-29.9377312333293));
#32508=CARTESIAN_POINT('Ctrl Pts',(2.33006853975684,3.35529515840789,-29.9435508645839));
#32509=CARTESIAN_POINT('Ctrl Pts',(2.38333476514479,3.31830468509675,-29.9467166641746));
#32510=CARTESIAN_POINT('Ctrl Pts',(2.43568426306117,3.2800702455178,-29.9498824637653));
#32511=CARTESIAN_POINT('Ctrl Pts',(2.4870572760686,3.24064362520074,-29.953048263356));
#32512=CARTESIAN_POINT('Ctrl Pts',(2.48705727606861,3.24064362520074,-28.7030585997167));
#32513=CARTESIAN_POINT('Ctrl Pts',(2.5820429500745,3.16774612736371,-28.7088749448307));
#32514=CARTESIAN_POINT('Ctrl Pts',(2.67379681749158,3.09068757207375,-28.7146912899448));
#32515=CARTESIAN_POINT('Ctrl Pts',(2.76194772936773,3.0097956309757,-28.7205076350588));
#32516=CARTESIAN_POINT('Ctrl Pts',(2.85019138505813,2.92881858324633,-28.7263300995654));
#32517=CARTESIAN_POINT('Ctrl Pts',(2.93482421452443,2.84400037004034,-28.7321525640719));
#32518=CARTESIAN_POINT('Ctrl Pts',(3.01551131907359,2.75570616803372,-28.7379750285785));
#32519=CARTESIAN_POINT('Ctrl Pts',(3.09624297403552,2.6673632154471,-28.7438007078887));
#32520=CARTESIAN_POINT('Ctrl Pts',(3.17302430283473,2.57554076189417,-28.7496263871989));
#32521=CARTESIAN_POINT('Ctrl Pts',(3.24556126143353,2.48063643008845,-28.7554520665091));
#32522=CARTESIAN_POINT('Ctrl Pts',(3.31821166631927,2.38558366989167,-28.7612868570599));
#32523=CARTESIAN_POINT('Ctrl Pts',(3.38660420697483,2.28743973558254,-28.7671216476108));
#32524=CARTESIAN_POINT('Ctrl Pts',(3.45048838246255,2.1866309525137,-28.7729564381616));
#32525=CARTESIAN_POINT('Ctrl Pts',(3.49920049723502,2.10976357536697,-28.7774055053182));
#32526=CARTESIAN_POINT('Ctrl Pts',(3.54529227459696,2.03134740200414,-28.7818545724747));
#32527=CARTESIAN_POINT('Ctrl Pts',(3.58867117582947,1.95157992195316,-28.7863036396313));
#32528=CARTESIAN_POINT('Ctrl Pts',(3.64540504598989,1.84725459955786,-28.7921224315145));
#32529=CARTESIAN_POINT('Ctrl Pts',(3.69767873305401,1.7402825949867,-28.7979412233978));
#32530=CARTESIAN_POINT('Ctrl Pts',(3.74523652803682,1.63108195657322,-28.803760015281));
#32531=CARTESIAN_POINT('Ctrl Pts',(3.79273386794356,1.52202013310909,-28.8095714103641));
#32532=CARTESIAN_POINT('Ctrl Pts',(3.8355270769139,1.41073568209517,-28.8153828054471));
#32533=CARTESIAN_POINT('Ctrl Pts',(3.87340569200842,1.29767227955165,-28.8211942005302));
#32534=CARTESIAN_POINT('Ctrl Pts',(3.91124607595361,1.18472299268568,-28.8269997301318));
#32535=CARTESIAN_POINT('Ctrl Pts',(3.94418160439638,1.06999871173745,-28.8328052597335));
#32536=CARTESIAN_POINT('Ctrl Pts',(3.97204964984305,0.953963615229478,-28.8386107893351));
#32537=CARTESIAN_POINT('Ctrl Pts',(4.00090495850115,0.833817818448801,-28.844621987677));
#32538=CARTESIAN_POINT('Ctrl Pts',(4.02432690494964,0.712267018809643,-28.8506331860188));
#32539=CARTESIAN_POINT('Ctrl Pts',(4.04219101456488,0.589844726831512,-28.8566443843606));
#32540=CARTESIAN_POINT('Ctrl Pts',(4.0594242412896,0.471745859367154,-28.8624432932424));
#32541=CARTESIAN_POINT('Ctrl Pts',(4.07148548363172,0.352836451920664,-28.8682422021241));
#32542=CARTESIAN_POINT('Ctrl Pts',(4.07831501460774,0.233605739709209,-28.8740411110058));
#32543=CARTESIAN_POINT('Ctrl Pts',(4.08514350486473,0.114393196486407,-28.87983913622));
#32544=CARTESIAN_POINT('Ctrl Pts',(4.08674184577814,-0.00514014580494544,
-28.8856371614342));
#32545=CARTESIAN_POINT('Ctrl Pts',(4.0831023036904,-0.124501315648307,-28.8914351866484));
#32546=CARTESIAN_POINT('Ctrl Pts',(4.07946245324251,-0.243872598364953,
-28.8972337031002));
#32547=CARTESIAN_POINT('Ctrl Pts',(4.07058385001204,-0.363071270689855,
-28.903032219552));
#32548=CARTESIAN_POINT('Ctrl Pts',(4.05651084924008,-0.481606405685688,
-28.9088307360038));
#32549=CARTESIAN_POINT('Ctrl Pts',(4.04243331929281,-0.600179689361881,
-28.9146311186175));
#32550=CARTESIAN_POINT('Ctrl Pts',(4.02315811549969,-0.718088604982401,
-28.9204315012311));
#32551=CARTESIAN_POINT('Ctrl Pts',(3.99878111898172,-0.834850023941597,
-28.9262318838448));
#32552=CARTESIAN_POINT('Ctrl Pts',(3.97437724410051,-0.951740185415469,
-28.9320386620286));
#32553=CARTESIAN_POINT('Ctrl Pts',(3.94486043195975,-1.06747992407829,-28.9378454402124));
#32554=CARTESIAN_POINT('Ctrl Pts',(3.91037712731112,-1.18159879917086,-28.9436522183963));
#32555=CARTESIAN_POINT('Ctrl Pts',(3.87587117640201,-1.29579261968403,-28.9494628100722));
#32556=CARTESIAN_POINT('Ctrl Pts',(3.83639237272657,-1.40836307167021,-28.9552734017482));
#32557=CARTESIAN_POINT('Ctrl Pts',(3.79213564343457,-1.51885886829325,-28.9610839934241));
#32558=CARTESIAN_POINT('Ctrl Pts',(3.74781584900742,-1.62951211966858,-28.9669028651008));
#32559=CARTESIAN_POINT('Ctrl Pts',(3.69870470839285,-1.7380844439387,-28.9727217367774));
#32560=CARTESIAN_POINT('Ctrl Pts',(3.64504351654909,-1.84414824850483,-28.9785406084541));
#32561=CARTESIAN_POINT('Ctrl Pts',(3.63170572170372,-1.87051101118706,-28.9799869221491));
#32562=CARTESIAN_POINT('Ctrl Pts',(3.61808703583387,-1.89671893567489,-28.9814332358441));
#32563=CARTESIAN_POINT('Ctrl Pts',(3.60419157521962,-1.92276573953145,-28.9828795495391));
#32564=CARTESIAN_POINT('Ctrl Pts',(3.54821053207587,-2.02770124983436,-28.988706355257));
#32565=CARTESIAN_POINT('Ctrl Pts',(3.48755364954155,-2.13035724183415,-28.9945331609749));
#32566=CARTESIAN_POINT('Ctrl Pts',(3.42243093206937,-2.23028955860327,-29.0003599666929));
#32567=CARTESIAN_POINT('Ctrl Pts',(3.35738987472761,-2.33009656601281,-29.0061794659326));
#32568=CARTESIAN_POINT('Ctrl Pts',(3.28789434159158,-2.42718635272648,-29.0119989651723));
#32569=CARTESIAN_POINT('Ctrl Pts',(3.21420056746468,-2.5211385745551,-29.0178184644121));
#32570=CARTESIAN_POINT('Ctrl Pts',(3.14058005737015,-2.61499739203983,-29.0236321780887));
#32571=CARTESIAN_POINT('Ctrl Pts',(3.06276985998779,-2.70572453117917,-29.0294458917653));
#32572=CARTESIAN_POINT('Ctrl Pts',(2.98106958028543,-2.79292841968727,-29.0352596054419));
#32573=CARTESIAN_POINT('Ctrl Pts',(2.89663673280179,-2.88304895103929,-29.0412677660255));
#32574=CARTESIAN_POINT('Ctrl Pts',(2.80804926529348,-2.96940604873364,-29.047275926609));
#32575=CARTESIAN_POINT('Ctrl Pts',(2.71568353120819,-3.05160416147387,-29.0532840871926));
#32576=CARTESIAN_POINT('Ctrl Pts',(2.62640662530868,-3.13105346427971,-29.0590913272081));
#32577=CARTESIAN_POINT('Ctrl Pts',(2.53360044283256,-3.20661720742733,-29.0648985672237));
#32578=CARTESIAN_POINT('Ctrl Pts',(2.43764192380558,-3.27797602970269,-29.0707058072392));
#32579=CARTESIAN_POINT('Ctrl Pts',(2.34169734481314,-3.34932448557748,-29.0765122036285));
#32580=CARTESIAN_POINT('Ctrl Pts',(2.24260166717051,-3.41646899216351,-29.0823186000178));
#32581=CARTESIAN_POINT('Ctrl Pts',(2.14076350622285,-3.47913158854684,-29.0881249964071));
#32582=CARTESIAN_POINT('Ctrl Pts',(2.03891618486954,-3.54179982146952,-29.0939319150854));
#32583=CARTESIAN_POINT('Ctrl Pts',(1.93432623706127,-3.59998512891101,-29.0997388337636));
#32584=CARTESIAN_POINT('Ctrl Pts',(1.82742918978747,-3.6534541951847,-29.1055457524419));
#32585=CARTESIAN_POINT('Ctrl Pts',(1.72049738272784,-3.70694064803118,-29.1113545593598));
#32586=CARTESIAN_POINT('Ctrl Pts',(1.61125734871256,-3.7557076273608,-29.1171633662778));
#32587=CARTESIAN_POINT('Ctrl Pts',(1.50016642568618,-3.79956914600115,-29.1229721731957));
#32588=CARTESIAN_POINT('Ctrl Pts',(1.38895336717806,-3.84347888683252,-29.1287873664269));
#32589=CARTESIAN_POINT('Ctrl Pts',(1.27588573739614,-3.88247225210961,-29.1346025596581));
#32590=CARTESIAN_POINT('Ctrl Pts',(1.16143808384948,-3.9164124626224,-29.1404177528893));
#32591=CARTESIAN_POINT('Ctrl Pts',(1.04691529150172,-3.95037495604486,-29.1462367639938));
#32592=CARTESIAN_POINT('Ctrl Pts',(0.931011065705889,-3.97927758902914,
-29.1520557750984));
#32593=CARTESIAN_POINT('Ctrl Pts',(0.814210640603455,-4.0030346029891,-29.1578747862029));
#32594=CARTESIAN_POINT('Ctrl Pts',(0.69724516002812,-4.02682518896021,-29.1637020203908));
#32595=CARTESIAN_POINT('Ctrl Pts',(0.579381353782573,-4.0454555794725,-29.1695292545787));
#32596=CARTESIAN_POINT('Ctrl Pts',(0.461110193239268,-4.05889176865938,
-29.1753564887666));
#32597=CARTESIAN_POINT('Ctrl Pts',(0.433378911481162,-4.06204217951512,
-29.1767228123267));
#32598=CARTESIAN_POINT('Ctrl Pts',(0.405625235287611,-4.06490725385444,
-29.1780891358869));
#32599=CARTESIAN_POINT('Ctrl Pts',(0.377855485250725,-4.06748696768237,
-29.179455459447));
#32600=CARTESIAN_POINT('Ctrl Pts',(0.259436741077086,-4.07848765985374,
-29.1852818828001));
#32601=CARTESIAN_POINT('Ctrl Pts',(0.140348538711738,-4.08433021474692,
-29.1911083061533));
#32602=CARTESIAN_POINT('Ctrl Pts',(0.0210772652008093,-4.08494562373744,
-29.1969347295064));
#32603=CARTESIAN_POINT('Ctrl Pts',(-0.0980447236284092,-4.08556026245753,
-29.2027538602758));
#32604=CARTESIAN_POINT('Ctrl Pts',(-0.217348923508945,-4.08096076647072,
-29.2085729910451));
#32605=CARTESIAN_POINT('Ctrl Pts',(-0.33634339722807,-4.07112983324544,
-29.2143921218145));
#32606=CARTESIAN_POINT('Ctrl Pts',(-0.455219855369642,-4.0613086500802,
-29.2202054813236));
#32607=CARTESIAN_POINT('Ctrl Pts',(-0.57378679427682,-4.04626638506521,
-29.2260188408327));
#32608=CARTESIAN_POINT('Ctrl Pts',(-0.691552442077824,-4.0260377817224,
-29.2318322003417));
#32609=CARTESIAN_POINT('Ctrl Pts',(-0.813267121606498,-4.00513085326611,
-29.2378404990506));
#32610=CARTESIAN_POINT('Ctrl Pts',(-0.934125382280565,-3.97868364374994,
-29.2438487977595));
#32611=CARTESIAN_POINT('Ctrl Pts',(-1.0535897799802,-3.94679282145912,-29.2498570964684));
#32612=CARTESIAN_POINT('Ctrl Pts',(-1.16905020009331,-3.91597085432622,
-29.2556640205935));
#32613=CARTESIAN_POINT('Ctrl Pts',(-1.28320826895366,-3.88006443957004,
-29.2614709447186));
#32614=CARTESIAN_POINT('Ctrl Pts',(-1.39558996935444,-3.83921263248563,
-29.2672778688437));
#32615=CARTESIAN_POINT('Ctrl Pts',(-1.5079556297809,-3.79836665608304,-29.2730839641602));
#32616=CARTESIAN_POINT('Ctrl Pts',(-1.61854504275882,-3.75257683041765,
-29.2788900594768));
#32617=CARTESIAN_POINT('Ctrl Pts',(-1.7269013388541,-3.70203143771956,-29.2846961547933));
#32618=CARTESIAN_POINT('Ctrl Pts',(-1.83526766642404,-3.65148136559956,
-29.2905027876301));
#32619=CARTESIAN_POINT('Ctrl Pts',(-1.94140009642179,-3.59617502350045,
-29.2963094204668));
#32620=CARTESIAN_POINT('Ctrl Pts',(-2.04486423824582,-3.53634772712517,
-29.3021160533036));
#32621=CARTESIAN_POINT('Ctrl Pts',(-2.14836230419483,-3.47650081440124,
-29.3079245900361));
#32622=CARTESIAN_POINT('Ctrl Pts',(-2.24918998908878,-3.41213020333553,
-29.3137331267685));
#32623=CARTESIAN_POINT('Ctrl Pts',(-2.34694042848864,-3.34351545908278,
-29.319541663501));
#32624=CARTESIAN_POINT('Ctrl Pts',(-2.44479875690645,-3.27482498343262,
-29.3253566112259));
#32625=CARTESIAN_POINT('Ctrl Pts',(-2.53957272641626,-3.20188125889247,
-29.3311715589508));
#32626=CARTESIAN_POINT('Ctrl Pts',(-2.6308870983957,-3.12500529207473,-29.3369865066757));
#32627=CARTESIAN_POINT('Ctrl Pts',(-2.72226164629221,-3.04807866420874,
-29.3428052864349));
#32628=CARTESIAN_POINT('Ctrl Pts',(-2.81017175667237,-2.96721490870144,
-29.3486240661942));
#32629=CARTESIAN_POINT('Ctrl Pts',(-2.8942789213397,-2.88277202107428,-29.3544428459534));
#32630=CARTESIAN_POINT('Ctrl Pts',(-2.97850527091434,-2.7982094728002,-29.3602698712733));
#32631=CARTESIAN_POINT('Ctrl Pts',(-3.05891764516055,-2.71005796986689,
-29.3660968965932));
#32632=CARTESIAN_POINT('Ctrl Pts',(-3.13521759930363,-2.61870876674303,
-29.3719239219131));
#32633=CARTESIAN_POINT('Ctrl Pts',(-3.15314544608915,-2.59724486763618,
-29.3732930710603));
#32634=CARTESIAN_POINT('Ctrl Pts',(-3.1708464403585,-2.57560455290277,-29.3746622202076));
#32635=CARTESIAN_POINT('Ctrl Pts',(-3.18831706365248,-2.55379312036477,
-29.3760313693548));
#32636=CARTESIAN_POINT('Ctrl Pts',(-3.26237872775687,-2.46132984855801,
-29.381835481924));
#32637=CARTESIAN_POINT('Ctrl Pts',(-3.33254054271542,-2.36548514299076,
-29.3876395944932));
#32638=CARTESIAN_POINT('Ctrl Pts',(-3.39847713634306,-2.26662263152769,
-29.3934437070624));
#32639=CARTESIAN_POINT('Ctrl Pts',(-3.46433414477886,-2.16787944670112,
-29.3992408140921));
#32640=CARTESIAN_POINT('Ctrl Pts',(-3.52597584417932,-2.06612603520603,
-29.4050379211218));
#32641=CARTESIAN_POINT('Ctrl Pts',(-3.58311662522096,-1.96175947813823,
-29.4108350281515));
#32642=CARTESIAN_POINT('Ctrl Pts',(-3.64020214125889,-1.85749386155564,
-29.4166265283775));
#32643=CARTESIAN_POINT('Ctrl Pts',(-3.69279519861236,-1.75062048281814,
-29.4224180286035));
#32644=CARTESIAN_POINT('Ctrl Pts',(-3.74065347945115,-1.64156527335042,
-29.4282095288295));
#32645=CARTESIAN_POINT('Ctrl Pts',(-3.78847694820317,-1.53258939058119,
-29.4339968163215));
#32646=CARTESIAN_POINT('Ctrl Pts',(-3.83157232612829,-1.4214352085985,-29.4397841038135));
#32647=CARTESIAN_POINT('Ctrl Pts',(-3.86974356700218,-1.30855253071677,
-29.4455713913055));
#32648=CARTESIAN_POINT('Ctrl Pts',(-3.90790030706425,-1.19571273565552,
-29.4513564802741));
#32649=CARTESIAN_POINT('Ctrl Pts',(-3.94113649529612,-1.08114613798668,
-29.4571415692426));
#32650=CARTESIAN_POINT('Ctrl Pts',(-3.9693047037138,-0.965321277645671,
-29.4629266582112));
#32651=CARTESIAN_POINT('Ctrl Pts',(-3.99746607423578,-0.84952453404903,
-29.4687103428364));
#32652=CARTESIAN_POINT('Ctrl Pts',(-4.02056181862068,-0.732470535382498,
-29.4744940274617));
#32653=CARTESIAN_POINT('Ctrl Pts',(-4.03849496394938,-0.61464089203007,
-29.4802777120869));
#32654=CARTESIAN_POINT('Ctrl Pts',(-4.05643362708318,-0.496774993966302,
-29.4860631762798));
#32655=CARTESIAN_POINT('Ctrl Pts',(-4.06920645404034,-0.378133380728452,
-29.4918486404727));
#32656=CARTESIAN_POINT('Ctrl Pts',(-4.07676802272873,-0.259205495421065,
-29.4976341046655));
#32657=CARTESIAN_POINT('Ctrl Pts',(-4.08232312608598,-0.171835172916947,
-29.5018843935785));
#32658=CARTESIAN_POINT('Ctrl Pts',(-4.08506673678685,-0.08431052717293,
-29.5061346824915));
#32659=CARTESIAN_POINT('Ctrl Pts',(-4.08499876708757,0.00317378213280428,
-29.5103849714045));
#32660=CARTESIAN_POINT('Ctrl Pts',(2.56728386697198,2.20447077508736,-28.0032546584631));
#32661=CARTESIAN_POINT('Ctrl Pts',(3.29391280982238,1.35834294948386,-28.0688249167149));
#32662=CARTESIAN_POINT('Ctrl Pts',(3.8330717178654,-1.09327735402418,-28.1999204782692));
#32663=CARTESIAN_POINT('Ctrl Pts',(1.19130828931765,-3.80720619125929,-28.3965413431262));
#32664=CARTESIAN_POINT('Ctrl Pts',(-2.52138985036123,-3.08713556078082,
-28.593117253034));
#32665=CARTESIAN_POINT('Ctrl Pts',(-3.96617369173339,0.405202913805355,
-28.7896931629418));
#32666=CARTESIAN_POINT('Ctrl Pts',(-1.84365258781347,3.53532882910493,-28.9862690728496));
#32667=CARTESIAN_POINT('Ctrl Pts',(1.93714903006732,3.48448758973885,-29.1828449827575));
#32668=CARTESIAN_POINT('Ctrl Pts',(3.97558571389243,0.300131850383572,-29.3794208926653));
#32669=CARTESIAN_POINT('Ctrl Pts',(2.43821705627172,-3.15447164483265,-29.5759968025731));
#32670=CARTESIAN_POINT('Ctrl Pts',(-1.29219047376943,-3.77165820795234,
-29.772572712481));
#32671=CARTESIAN_POINT('Ctrl Pts',(-3.86034553203149,-0.996531969245317,
-29.9691486223888));
#32672=CARTESIAN_POINT('Ctrl Pts',(-2.95634241771665,2.67495669448989,-30.1657245322966));
#32673=CARTESIAN_POINT('Ctrl Pts',(0.606721126975111,3.94045560524475,-30.3623004422045));
#32674=CARTESIAN_POINT('Ctrl Pts',(3.62407370691447,1.66175139044748,-30.5588763521123));
#32675=CARTESIAN_POINT('Ctrl Pts',(3.3817804106626,-2.11160786060308,-30.7554522620201));
#32676=CARTESIAN_POINT('Ctrl Pts',(0.0977699855536051,-3.98569458351054,
-30.9520281719279));
#32677=CARTESIAN_POINT('Ctrl Pts',(-3.27417889645636,-2.27487948951289,
-31.1486040818358));
#32678=CARTESIAN_POINT('Ctrl Pts',(-3.70119208770647,1.48205962121795,-31.3451799917436));
#32679=CARTESIAN_POINT('Ctrl Pts',(-0.799195750105958,3.90597094842635,
-31.5417559016514));
#32680=CARTESIAN_POINT('Ctrl Pts',(2.82163122020526,2.81668611762427,-31.7383318115593));
#32681=CARTESIAN_POINT('Ctrl Pts',(3.90456310915817,-0.806046051412663,
-31.9349077214671));
#32682=CARTESIAN_POINT('Ctrl Pts',(1.47556493170961,-3.70378608599469,-32.1314836313749));
#32683=CARTESIAN_POINT('Ctrl Pts',(-2.28061907953618,-3.27018346938094,
-32.3280595412828));
#32684=CARTESIAN_POINT('Ctrl Pts',(-3.9855173287882,0.104761205677251,-32.5246354511906));
#32685=CARTESIAN_POINT('Ctrl Pts',(-2.10567184542122,3.38547919224393,-32.7212113610984));
#32686=CARTESIAN_POINT('Ctrl Pts',(1.66810441974091,3.62115326045451,-32.9177872710062));
#32687=CARTESIAN_POINT('Ctrl Pts',(3.9415166492128,0.599808128823799,-33.1143631809141));
#32688=CARTESIAN_POINT('Ctrl Pts',(2.66976122810008,-2.96102993432676,-33.3109390908219));
#32689=CARTESIAN_POINT('Ctrl Pts',(-1.00329094829934,-3.85859178472063,
-33.5075150007297));
#32690=CARTESIAN_POINT('Ctrl Pts',(-3.77394059016891,-1.28557213310189,
-33.7040909106375));
#32691=CARTESIAN_POINT('Ctrl Pts',(-3.15014761363694,2.44374575198617,-33.9006668205454));
#32692=CARTESIAN_POINT('Ctrl Pts',(0.30702205740443,3.97505481010171,-34.0972427304532));
#32693=CARTESIAN_POINT('Ctrl Pts',(3.48804303651859,1.93103057014098,-34.2938186403611));
#32694=CARTESIAN_POINT('Ctrl Pts',(3.53176981253407,-1.84984466432527,-34.4903945502688));
#32695=CARTESIAN_POINT('Ctrl Pts',(0.398872662601994,-3.96689095901879,
-34.6869704601767));
#32696=CARTESIAN_POINT('Ctrl Pts',(-3.09278751656281,-2.51594687258676,
-34.8835463700845));
#32697=CARTESIAN_POINT('Ctrl Pts',(-3.80266311499646,1.19794680316039,-35.0801222799923));
#32698=CARTESIAN_POINT('Ctrl Pts',(-1.092261827831,3.83435618298071,-35.2766981899002));
#32699=CARTESIAN_POINT('Ctrl Pts',(2.6005661715146,3.02198261046796,-35.473274099808));
#32700=CARTESIAN_POINT('Ctrl Pts',(3.95433441888669,-0.508490640683108,
-35.6698500097158));
#32701=CARTESIAN_POINT('Ctrl Pts',(1.75140611463455,-3.58160571790905,-35.8664259196237));
#32702=CARTESIAN_POINT('Ctrl Pts',(-2.02681120527418,-3.43327248104789,
-36.0630018295315));
#32703=CARTESIAN_POINT('Ctrl Pts',(-3.98202856408726,-0.196907726104969,
-36.2595777394393));
#32704=CARTESIAN_POINT('Ctrl Pts',(-2.35563972507278,3.21656365843416,-36.4561536493472));
#32705=CARTESIAN_POINT('Ctrl Pts',(1.38951083230835,3.73692201548276,-36.6527295592549));
#32706=CARTESIAN_POINT('Ctrl Pts',(3.88487784518938,0.896131711725264,-36.8493054691628));
#32707=CARTESIAN_POINT('Ctrl Pts',(2.88601746641837,-2.75067338779994,-37.0458813790706));
#32708=CARTESIAN_POINT('Ctrl Pts',(-0.708643658991017,-3.92341407103033,
-37.2424572889785));
#32709=CARTESIAN_POINT('Ctrl Pts',(-3.66593245019103,-1.56725328617931,
-37.4390331988863));
#32710=CARTESIAN_POINT('Ctrl Pts',(-3.32590237765776,2.19853024368671,-37.6356091087942));
#32711=CARTESIAN_POINT('Ctrl Pts',(0.00553985079000487,3.98692401251902,
-37.832185018702));
#32712=CARTESIAN_POINT('Ctrl Pts',(3.33208928316455,2.18918749885435,-38.0287609286098));
#32713=CARTESIAN_POINT('Ctrl Pts',(3.66143934028185,-1.57735921247231,-38.2253368385177));
#32714=CARTESIAN_POINT('Ctrl Pts',(0.697881833191951,-3.9256293433477,-38.4219127484254));
#32715=CARTESIAN_POINT('Ctrl Pts',(-2.89406083608174,-2.74210412483044,
-38.6184886583333));
#32716=CARTESIAN_POINT('Ctrl Pts',(-3.88162410493238,0.90598402643207,-38.8150645682411));
#32717=CARTESIAN_POINT('Ctrl Pts',(-1.38054113569662,3.74274506153031,-39.0116404781489));
#32718=CARTESIAN_POINT('Ctrl Pts',(2.36774286239059,3.20596553681761,-39.2082163880568));
#32719=CARTESIAN_POINT('Ctrl Pts',(3.43742279325449,0.936456751147026,-39.339266994662));
#32720=CARTESIAN_POINT('Ctrl Pts',(3.37926985666995,-0.176560176875435,
-39.4047922979646));
#32721=CARTESIAN_POINT('Ctrl Pts',(2.74548793878474,2.35749073262566,-27.8676427113695));
#32722=CARTESIAN_POINT('Ctrl Pts',(3.52255471516762,1.45263024183603,-27.9332129696212));
#32723=CARTESIAN_POINT('Ctrl Pts',(4.09913851182676,-1.1691655246368,-28.0643085311756));
#32724=CARTESIAN_POINT('Ctrl Pts',(1.27400112693951,-4.07147756936497,-28.2609293960326));
#32725=CARTESIAN_POINT('Ctrl Pts',(-2.69640825940523,-3.30142434054789,
-28.4575053059404));
#32726=CARTESIAN_POINT('Ctrl Pts',(-4.24147955505312,0.433329452549069,
-28.6540812158482));
#32727=CARTESIAN_POINT('Ctrl Pts',(-1.97162690432098,3.78072825713415,-28.8506571257561));
#32728=CARTESIAN_POINT('Ctrl Pts',(2.07161325870492,3.72635795112,-29.0472330356639));
#32729=CARTESIAN_POINT('Ctrl Pts',(4.25154489829376,0.320965042422498,-29.2438089455717));
#32730=CARTESIAN_POINT('Ctrl Pts',(2.60746215338809,-3.37343445559113,-29.4403848554795));
#32731=CARTESIAN_POINT('Ctrl Pts',(-1.38188589348746,-4.03346207732183,
-29.6369607653874));
#32732=CARTESIAN_POINT('Ctrl Pts',(-4.12830549596942,-1.06570470736585,
-29.8335366752952));
#32733=CARTESIAN_POINT('Ctrl Pts',(-3.16155239207421,2.86063471047149,-30.0301125852031));
#32734=CARTESIAN_POINT('Ctrl Pts',(0.648835743388491,4.21397628703841,-30.2266884951108));
#32735=CARTESIAN_POINT('Ctrl Pts',(3.87563322451603,1.7770993143479,-30.4232644050187));
#32736=CARTESIAN_POINT('Ctrl Pts',(3.61652151074496,-2.25818188136967,-30.6198403149265));
#32737=CARTESIAN_POINT('Ctrl Pts',(0.104556539136899,-4.26235545959098,
-30.8164162248343));
#32738=CARTESIAN_POINT('Ctrl Pts',(-3.50145100247405,-2.43278675996705,
-31.0129921347422));
#32739=CARTESIAN_POINT('Ctrl Pts',(-3.95810465942314,1.58493451657646,-31.20956804465));
#32740=CARTESIAN_POINT('Ctrl Pts',(-0.854670697257917,4.17709793066106,
-31.4061439545578));
#32741=CARTESIAN_POINT('Ctrl Pts',(3.01749042341354,3.0122020641219,-31.6027198644657));
#32742=CARTESIAN_POINT('Ctrl Pts',(4.17559236838947,-0.861996501722528,
-31.7992957743735));
#32743=CARTESIAN_POINT('Ctrl Pts',(1.57798900815773,-3.96087871612375,-31.9958716842813));
#32744=CARTESIAN_POINT('Ctrl Pts',(-2.43892475482816,-3.49717823895654,
-32.1924475941892));
#32745=CARTESIAN_POINT('Ctrl Pts',(-4.26216590100397,0.112033044081982,
-32.3890235040969));
#32746=CARTESIAN_POINT('Ctrl Pts',(-2.2518338267989,3.62047703757641,-32.5855994140048));
#32747=CARTESIAN_POINT('Ctrl Pts',(1.78389332942519,3.87251005974457,-32.7821753239126));
#32748=CARTESIAN_POINT('Ctrl Pts',(4.21511098174603,0.64144289007397,-32.9787512338205));
#32749=CARTESIAN_POINT('Ctrl Pts',(2.85507860875126,-3.1665652854599,-33.1753271437283));
#32750=CARTESIAN_POINT('Ctrl Pts',(-1.07293285058369,-4.12643001497894,
-33.3719030536361));
#32751=CARTESIAN_POINT('Ctrl Pts',(-4.03590288759914,-1.37480815085398,
-33.5684789635439));
#32752=CARTESIAN_POINT('Ctrl Pts',(-3.36881027840236,2.6133746150354,-33.7650548734518));
#32753=CARTESIAN_POINT('Ctrl Pts',(0.328333522595203,4.25097714263074,-33.9616307833595));
#32754=CARTESIAN_POINT('Ctrl Pts',(3.73016019378445,2.06507009526757,-34.1582066932675));
#32755=CARTESIAN_POINT('Ctrl Pts',(3.77692219688698,-1.97824879432617,-34.3547826031752));
#32756=CARTESIAN_POINT('Ctrl Pts',(0.426559796668051,-4.24224661034696,
-34.5513585130831));
#32757=CARTESIAN_POINT('Ctrl Pts',(-3.30746861817128,-2.69058746567722,
-34.7479344229909));
#32758=CARTESIAN_POINT('Ctrl Pts',(-4.06661914243173,1.28110044303818,-34.9445103328988));
#32759=CARTESIAN_POINT('Ctrl Pts',(-1.16807950725057,4.10051213611788,-35.1410862428066));
#32760=CARTESIAN_POINT('Ctrl Pts',(2.78108048344732,3.23174889812353,-35.3376621527144));
#32761=CARTESIAN_POINT('Ctrl Pts',(4.22881847724137,-0.54378673856078,-35.5342380626223));
#32762=CARTESIAN_POINT('Ctrl Pts',(1.87297728369805,-3.83021738519307,-35.7308139725301));
#32763=CARTESIAN_POINT('Ctrl Pts',(-2.16749919627598,-3.67158782421524,
-35.9273898824379));
#32764=CARTESIAN_POINT('Ctrl Pts',(-4.25843496905253,-0.210575773886802,
-36.1239657923457));
#32765=CARTESIAN_POINT('Ctrl Pts',(-2.51915284340472,3.43983649107734,-36.3205417022536));
#32766=CARTESIAN_POINT('Ctrl Pts',(1.48596159544011,3.99631472533188,-36.5171176121614));
#32767=CARTESIAN_POINT('Ctrl Pts',(4.15454068201641,0.958335319968377,-36.7136935220692));
#32768=CARTESIAN_POINT('Ctrl Pts',(3.08634594214907,-2.94160716191005,-36.910269431977));
#32769=CARTESIAN_POINT('Ctrl Pts',(-0.757833071631014,-4.19575184086556,
-37.1068453418849));
#32770=CARTESIAN_POINT('Ctrl Pts',(-3.92039752825235,-1.67604176911731,
-37.3034212517927));
#32771=CARTESIAN_POINT('Ctrl Pts',(-3.55676478978729,2.35113784834968,-37.4999971617006));
#32772=CARTESIAN_POINT('Ctrl Pts',(0.00592439103532244,4.26367022752833,
-37.6965730716083));
#32773=CARTESIAN_POINT('Ctrl Pts',(3.56338114985008,2.34114659121509,-37.8931489815162));
#32774=CARTESIAN_POINT('Ctrl Pts',(3.91559253601055,-1.68684918278303,-38.089724891424));
#32775=CARTESIAN_POINT('Ctrl Pts',(0.746324230201072,-4.19812088291295,
-38.2863008013318));
#32776=CARTESIAN_POINT('Ctrl Pts',(-3.09494762998035,-2.93244307669544,
-38.4828767112397));
#32777=CARTESIAN_POINT('Ctrl Pts',(-4.15106108837021,0.968871517988643,
-38.6794526211475));
#32778=CARTESIAN_POINT('Ctrl Pts',(-1.47636928109619,4.00254196918918,-38.8760285310553));
#32779=CARTESIAN_POINT('Ctrl Pts',(2.53209610143512,3.42850271710462,-39.0726044409632));
#32780=CARTESIAN_POINT('Ctrl Pts',(3.67602622397774,1.00145946014927,-39.2036550475684));
#32781=CARTESIAN_POINT('Ctrl Pts',(3.61383669049771,-0.188815830737465,
-39.269180350871));
#32782=CARTESIAN_POINT('Ctrl Pts',(2.92369201059751,2.51051069016395,-27.7320307642759));
#32783=CARTESIAN_POINT('Ctrl Pts',(3.75119662051287,1.54691753418819,-27.7976010225276));
#32784=CARTESIAN_POINT('Ctrl Pts',(4.36520530578812,-1.24505369524941,-27.9286965840819));
#32785=CARTESIAN_POINT('Ctrl Pts',(1.35669396456135,-4.33574894747066,-28.125317448939));
#32786=CARTESIAN_POINT('Ctrl Pts',(-2.87142666844923,-3.51571312031497,
-28.3218933588468));
#32787=CARTESIAN_POINT('Ctrl Pts',(-4.51678541837286,0.461455991292788,
-28.5184692687547));
#32788=CARTESIAN_POINT('Ctrl Pts',(-2.0996012208285,4.02612768516337,-28.7150451786624));
#32789=CARTESIAN_POINT('Ctrl Pts',(2.20607748734252,3.96822831250115,-28.9116210885703));
#32790=CARTESIAN_POINT('Ctrl Pts',(4.52750408269509,0.341798234461419,-29.1081969984781));
#32791=CARTESIAN_POINT('Ctrl Pts',(2.77670725050445,-3.59239726634962,-29.304772908386));
#32792=CARTESIAN_POINT('Ctrl Pts',(-1.47158131320549,-4.29526594669133,
-29.5013488182938));
#32793=CARTESIAN_POINT('Ctrl Pts',(-4.39626545990734,-1.13487744548638,
-29.6979247282016));
#32794=CARTESIAN_POINT('Ctrl Pts',(-3.36676236643178,3.04631272645307,-29.8945006381094));
#32795=CARTESIAN_POINT('Ctrl Pts',(0.690950359801877,4.48749696883208,-30.0910765480173));
#32796=CARTESIAN_POINT('Ctrl Pts',(4.12719274211759,1.89244723824832,-30.287652457925));
#32797=CARTESIAN_POINT('Ctrl Pts',(3.85126261082733,-2.40475590213628,-30.484228367833));
#32798=CARTESIAN_POINT('Ctrl Pts',(0.111343092720193,-4.53901633567143,
-30.6808042777407));
#32799=CARTESIAN_POINT('Ctrl Pts',(-3.72872310849174,-2.59069403042121,
-30.8773801876486));
#32800=CARTESIAN_POINT('Ctrl Pts',(-4.2150172311398,1.68780941193497,-31.0739560975564));
#32801=CARTESIAN_POINT('Ctrl Pts',(-0.910145644409873,4.44822491289575,
-31.2705320074642));
#32802=CARTESIAN_POINT('Ctrl Pts',(3.21334962662181,3.20771801061954,-31.4671079173721));
#32803=CARTESIAN_POINT('Ctrl Pts',(4.44662162762077,-0.917946952032398,
-31.6636838272799));
#32804=CARTESIAN_POINT('Ctrl Pts',(1.68041308460585,-4.2179713462528,-31.8602597371878));
#32805=CARTESIAN_POINT('Ctrl Pts',(-2.59723043012015,-3.72417300853216,
-32.0568356470955));
#32806=CARTESIAN_POINT('Ctrl Pts',(-4.53881447321974,0.119304882486721,
-32.2534115570034));
#32807=CARTESIAN_POINT('Ctrl Pts',(-2.39799580817657,3.85547488290889,-32.4499874669112));
#32808=CARTESIAN_POINT('Ctrl Pts',(1.89968223910945,4.12386685903462,-32.6465633768191));
#32809=CARTESIAN_POINT('Ctrl Pts',(4.48870531427926,0.683077651324139,-32.8431392867268));
#32810=CARTESIAN_POINT('Ctrl Pts',(3.04039598940244,-3.37210063659303,-33.0397151966347));
#32811=CARTESIAN_POINT('Ctrl Pts',(-1.14257475286803,-4.39426824523726,
-33.2362911065425));
#32812=CARTESIAN_POINT('Ctrl Pts',(-4.29786518502939,-1.46404416860608,
-33.4328670164504));
#32813=CARTESIAN_POINT('Ctrl Pts',(-3.58747294316779,2.78300347808462,-33.6294429263582));
#32814=CARTESIAN_POINT('Ctrl Pts',(0.349644987785975,4.52689947515976,-33.826018836266));
#32815=CARTESIAN_POINT('Ctrl Pts',(3.97227735105031,2.19910962039414,-34.0225947461739));
#32816=CARTESIAN_POINT('Ctrl Pts',(4.02207458123991,-2.10665292432707,-34.2191706560816));
#32817=CARTESIAN_POINT('Ctrl Pts',(0.454246930734107,-4.51760226167515,
-34.4157465659895));
#32818=CARTESIAN_POINT('Ctrl Pts',(-3.52214971977974,-2.86522805876768,
-34.6123224758973));
#32819=CARTESIAN_POINT('Ctrl Pts',(-4.330575169867,1.36425408291597,-34.8088983858051));
#32820=CARTESIAN_POINT('Ctrl Pts',(-1.24389718667016,4.36666808925506,-35.005474295713));
#32821=CARTESIAN_POINT('Ctrl Pts',(2.96159479538005,3.4415151857791,-35.2020502056208));
#32822=CARTESIAN_POINT('Ctrl Pts',(4.50330253559606,-0.579082836438446,
-35.3986261155287));
#32823=CARTESIAN_POINT('Ctrl Pts',(1.99454845276156,-4.0788290524771,-35.5952020254364));
#32824=CARTESIAN_POINT('Ctrl Pts',(-2.30818718727777,-3.9099031673826,-35.7917779353443));
#32825=CARTESIAN_POINT('Ctrl Pts',(-4.53484137401781,-0.224243821668637,
-35.9883538452521));
#32826=CARTESIAN_POINT('Ctrl Pts',(-2.68266596173667,3.6631093237205,-36.18492975516));
#32827=CARTESIAN_POINT('Ctrl Pts',(1.58241235857187,4.25570743518099,-36.3815056650678));
#32828=CARTESIAN_POINT('Ctrl Pts',(4.42420351884345,1.02053892821149,-36.5780815749756));
#32829=CARTESIAN_POINT('Ctrl Pts',(3.28667441787977,-3.13254093602017,-36.7746574848834));
#32830=CARTESIAN_POINT('Ctrl Pts',(-0.807022484271015,-4.46808961070079,
-36.9712333947913));
#32831=CARTESIAN_POINT('Ctrl Pts',(-4.17486260631367,-1.78483025205532,
-37.1678093046991));
#32832=CARTESIAN_POINT('Ctrl Pts',(-3.78762720191682,2.50374545301266,-37.364385214607));
#32833=CARTESIAN_POINT('Ctrl Pts',(0.00630893128064401,4.54041644253765,
-37.5609611245147));
#32834=CARTESIAN_POINT('Ctrl Pts',(3.79467301653562,2.49310568357585,-37.7575370344226));
#32835=CARTESIAN_POINT('Ctrl Pts',(4.16974573173925,-1.79633915309375,-37.9541129443304));
#32836=CARTESIAN_POINT('Ctrl Pts',(0.794766627210192,-4.4706124224782,-38.1506888542383));
#32837=CARTESIAN_POINT('Ctrl Pts',(-3.29583442387897,-3.12278202856045,
-38.3472647641461));
#32838=CARTESIAN_POINT('Ctrl Pts',(-4.42049807180803,1.03175900954522,-38.5438406740539));
#32839=CARTESIAN_POINT('Ctrl Pts',(-1.57219742649575,4.26233887684804,-38.7404165839617));
#32840=CARTESIAN_POINT('Ctrl Pts',(2.69644934047965,3.65103989739164,-38.9369924938696));
#32841=CARTESIAN_POINT('Ctrl Pts',(3.91462965470099,1.06646216915153,-39.0680431004748));
#32842=CARTESIAN_POINT('Ctrl Pts',(3.84840352432548,-0.201071484599496,
-39.1335684037774));
#32843=CARTESIAN_POINT('Ctrl Pts',(3.10189608241027,2.66353064770225,-27.5964188171822));
#32844=CARTESIAN_POINT('Ctrl Pts',(3.97983852585811,1.64120482654036,-27.661989075434));
#32845=CARTESIAN_POINT('Ctrl Pts',(4.63127209974949,-1.32094186586204,-27.7930846369884));
#32846=CARTESIAN_POINT('Ctrl Pts',(1.4393868021832,-4.60002032557634,-27.9897055018454));
#32847=CARTESIAN_POINT('Ctrl Pts',(-3.04644507749322,-3.73000190008205,
-28.1862814117532));
#32848=CARTESIAN_POINT('Ctrl Pts',(-4.7920912816926,0.489582530036508,-28.3828573216609));
#32849=CARTESIAN_POINT('Ctrl Pts',(-2.22757553733602,4.27152711319258,-28.5794332315689));
#32850=CARTESIAN_POINT('Ctrl Pts',(2.34054171598012,4.2100986738823,-28.7760091414767));
#32851=CARTESIAN_POINT('Ctrl Pts',(4.80346326709643,0.362631426500339,-28.9725850513845));
#32852=CARTESIAN_POINT('Ctrl Pts',(2.94595234762082,-3.81136007710809,-29.1691609612924));
#32853=CARTESIAN_POINT('Ctrl Pts',(-1.56127673292352,-4.55706981606083,
-29.3657368712001));
#32854=CARTESIAN_POINT('Ctrl Pts',(-4.66422542384527,-1.2040501836069,-29.562312781108));
#32855=CARTESIAN_POINT('Ctrl Pts',(-3.57197234078933,3.23199074243467,-29.7588886910158));
#32856=CARTESIAN_POINT('Ctrl Pts',(0.73306497621526,4.76101765062574,-29.9554646009237));
#32857=CARTESIAN_POINT('Ctrl Pts',(4.37875225971916,2.00779516214874,-30.1520405108315));
#32858=CARTESIAN_POINT('Ctrl Pts',(4.0860037109097,-2.55132992290288,-30.3486164207393));
#32859=CARTESIAN_POINT('Ctrl Pts',(0.118129646303484,-4.81567721175188,
-30.5451923306472));
#32860=CARTESIAN_POINT('Ctrl Pts',(-3.95599521450942,-2.74860130087537,
-30.7417682405549));
#32861=CARTESIAN_POINT('Ctrl Pts',(-4.47192980285647,1.79068430729347,-30.9383441504629));
#32862=CARTESIAN_POINT('Ctrl Pts',(-0.965620591561828,4.71935189513045,
-31.1349200603706));
#32863=CARTESIAN_POINT('Ctrl Pts',(3.40920882983009,3.40323395711717,-31.3314959702785));
#32864=CARTESIAN_POINT('Ctrl Pts',(4.71765088685207,-0.973897402342265,
-31.5280718801863));
#32865=CARTESIAN_POINT('Ctrl Pts',(1.78283716105399,-4.47506397638186,-31.7246477900941));
#32866=CARTESIAN_POINT('Ctrl Pts',(-2.75553610541214,-3.95116777810775,
-31.921223700002));
#32867=CARTESIAN_POINT('Ctrl Pts',(-4.81546304543552,0.126576720891454,
-32.1177996099098));
#32868=CARTESIAN_POINT('Ctrl Pts',(-2.54415778955425,4.09047272824138,-32.3143755198176));
#32869=CARTESIAN_POINT('Ctrl Pts',(2.01547114879372,4.37522365832467,-32.5109514297255));
#32870=CARTESIAN_POINT('Ctrl Pts',(4.7622996468125,0.724712412574313,-32.7075273396332));
#32871=CARTESIAN_POINT('Ctrl Pts',(3.22571337005362,-3.57763598772617,-32.9041032495411));
#32872=CARTESIAN_POINT('Ctrl Pts',(-1.21221665515238,-4.66210647549557,
-33.1006791594489));
#32873=CARTESIAN_POINT('Ctrl Pts',(-4.55982748245962,-1.55328018635817,
-33.2972550693568));
#32874=CARTESIAN_POINT('Ctrl Pts',(-3.80613560793321,2.95263234113385,-33.4938309792646));
#32875=CARTESIAN_POINT('Ctrl Pts',(0.370956452976748,4.80282180768878,-33.6904068891724));
#32876=CARTESIAN_POINT('Ctrl Pts',(4.21439450831618,2.33314914552072,-33.8869827990801));
#32877=CARTESIAN_POINT('Ctrl Pts',(4.26722696559284,-2.23505705432797,-34.0835587089881));
#32878=CARTESIAN_POINT('Ctrl Pts',(0.48193406480016,-4.79295791300333,-34.2801346188959));
#32879=CARTESIAN_POINT('Ctrl Pts',(-3.73683082138821,-3.03986865185813,
-34.4767105288038));
#32880=CARTESIAN_POINT('Ctrl Pts',(-4.59453119730227,1.44740772279378,-34.6732864387115));
#32881=CARTESIAN_POINT('Ctrl Pts',(-1.31971486608973,4.63282404239223,-34.8698623486193));
#32882=CARTESIAN_POINT('Ctrl Pts',(3.14210910731277,3.65128147343468,-35.0664382585272));
#32883=CARTESIAN_POINT('Ctrl Pts',(4.77778659395074,-0.614378934316126,
-35.263014168435));
#32884=CARTESIAN_POINT('Ctrl Pts',(2.11611962182505,-4.32744071976112,-35.4595900783428));
#32885=CARTESIAN_POINT('Ctrl Pts',(-2.44887517827956,-4.14821851054996,
-35.6561659882507));
#32886=CARTESIAN_POINT('Ctrl Pts',(-4.81124777898309,-0.237911869450464,
-35.8527418981585));
#32887=CARTESIAN_POINT('Ctrl Pts',(-2.84617908006861,3.88638215636366,-36.0493178080664));
#32888=CARTESIAN_POINT('Ctrl Pts',(1.67886312170362,4.51510014503012,-36.2458937179742));
#32889=CARTESIAN_POINT('Ctrl Pts',(4.69386635567049,1.0827425364546,-36.442469627882));
#32890=CARTESIAN_POINT('Ctrl Pts',(3.48700289361047,-3.32347471013028,-36.6390455377899));
#32891=CARTESIAN_POINT('Ctrl Pts',(-0.856211896911012,-4.74042738053602,
-36.8356214476976));
#32892=CARTESIAN_POINT('Ctrl Pts',(-4.42932768437499,-1.89361873499331,
-37.0321973576056));
#32893=CARTESIAN_POINT('Ctrl Pts',(-4.01848961404635,2.65635305767562,-37.2287732675133));
#32894=CARTESIAN_POINT('Ctrl Pts',(0.00669347152596622,4.81716265754697,
-37.4253491774212));
#32895=CARTESIAN_POINT('Ctrl Pts',(4.02596488322114,2.64506477593659,-37.621925087329));
#32896=CARTESIAN_POINT('Ctrl Pts',(4.42389892746796,-1.90582912340446,-37.8185009972368));
#32897=CARTESIAN_POINT('Ctrl Pts',(0.843209024219307,-4.74310396204345,
-38.0150769071447));
#32898=CARTESIAN_POINT('Ctrl Pts',(-3.49672121777756,-3.31312098042544,
-38.2116528170525));
#32899=CARTESIAN_POINT('Ctrl Pts',(-4.68993505524586,1.09464650110178,-38.4082287269604));
#32900=CARTESIAN_POINT('Ctrl Pts',(-1.66802557189533,4.52213578450691,-38.6048046368681));
#32901=CARTESIAN_POINT('Ctrl Pts',(2.86080257952418,3.87357707767866,-38.801380546776));
#32902=CARTESIAN_POINT('Ctrl Pts',(4.15323308542423,1.13146487815378,-38.9324311533812));
#32903=CARTESIAN_POINT('Ctrl Pts',(4.08297035815325,-0.213327138461527,
-38.9979564566838));
#32904=CARTESIAN_POINT('Ctrl Pts',(4.07943565862452,-0.213142457391218,
-39.));
#32905=CARTESIAN_POINT('Ctrl Pts',(4.07547862263307,-0.0893448369054089,
-39.));
#32906=CARTESIAN_POINT('Ctrl Pts',(4.06544764788375,0.0339030770314181,
-39.));
#32907=CARTESIAN_POINT('Ctrl Pts',(4.04961725587858,0.156269764503743,-39.));
#32908=CARTESIAN_POINT('Ctrl Pts',(4.03355455981531,0.280432129434245,-39.));
#32909=CARTESIAN_POINT('Ctrl Pts',(4.01152059276709,0.403687980955931,-39.));
#32910=CARTESIAN_POINT('Ctrl Pts',(3.98374860021197,0.525679242089098,-39.));
#32911=CARTESIAN_POINT('Ctrl Pts',(3.9558662643795,0.648155197128751,-39.));
#32912=CARTESIAN_POINT('Ctrl Pts',(3.9221997260414,0.769357256097345,-39.));
#32913=CARTESIAN_POINT('Ctrl Pts',(3.88293829909243,0.888899762117013,-39.));
#32914=CARTESIAN_POINT('Ctrl Pts',(3.84594470302387,1.00153721634053,-39.));
#32915=CARTESIAN_POINT('Ctrl Pts',(3.80398315981906,1.11270162038201,-39.));
#32916=CARTESIAN_POINT('Ctrl Pts',(3.75718016985247,1.22204245191786,-39.));
#32917=CARTESIAN_POINT('Ctrl Pts',(3.74832861001601,1.24272140669402,-39.));
#32918=CARTESIAN_POINT('Ctrl Pts',(3.73930380307158,1.26333504411753,-39.));
#32919=CARTESIAN_POINT('Ctrl Pts',(3.73010649791783,1.28388085829669,-39.));
#32920=CARTESIAN_POINT('Ctrl Pts',(3.72331964578407,1.29904197347889,-39.));
#32921=CARTESIAN_POINT('Ctrl Pts',(3.71643932891027,1.31416499535076,-39.));
#32922=CARTESIAN_POINT('Ctrl Pts',(3.70947119635962,1.32923777417663,-39.));
#32923=CARTESIAN_POINT('Ctrl Pts',(3.65772911496908,1.44116115438239,-39.));
#32924=CARTESIAN_POINT('Ctrl Pts',(3.60107392087828,1.55048480765739,-39.));
#32925=CARTESIAN_POINT('Ctrl Pts',(3.53972500093587,1.65686661310373,-39.));
#32926=CARTESIAN_POINT('Ctrl Pts',(3.47866871745544,1.76274097367257,-39.));
#32927=CARTESIAN_POINT('Ctrl Pts',(3.41296282504321,1.86570215783094,-39.));
#32928=CARTESIAN_POINT('Ctrl Pts',(3.34278310915447,1.96538145265714,-39.));
#32929=CARTESIAN_POINT('Ctrl Pts',(3.27420369022065,2.06278777629846,-39.));
#32930=CARTESIAN_POINT('Ctrl Pts',(3.20135157516031,2.15706065609363,-39.));
#32931=CARTESIAN_POINT('Ctrl Pts',(3.12436054260474,2.2478176249695,-39.));
#32932=CARTESIAN_POINT('Ctrl Pts',(3.05951101564277,2.32426219656105,-39.));
#32933=CARTESIAN_POINT('Ctrl Pts',(2.99172440946438,2.39821187176379,-39.));
#32934=CARTESIAN_POINT('Ctrl Pts',(2.92106768956024,2.46941240302989,-39.));
#32935=CARTESIAN_POINT('Ctrl Pts',(2.90675811120593,2.48383211544229,-39.));
#32936=CARTESIAN_POINT('Ctrl Pts',(2.89233078089546,2.4981389856815,-39.));
#32937=CARTESIAN_POINT('Ctrl Pts',(2.87778620684771,2.51233076884828,-39.));
#32938=CARTESIAN_POINT('Ctrl Pts',(2.86578714363673,2.52403878468538,-39.));
#32939=CARTESIAN_POINT('Ctrl Pts',(2.85370820051999,2.5356684616658,-39.));
#32940=CARTESIAN_POINT('Ctrl Pts',(2.84156035651544,2.54720861596515,-39.));
#32941=CARTESIAN_POINT('Ctrl Pts',(2.75684747169488,2.62768378189632,-39.));
#32942=CARTESIAN_POINT('Ctrl Pts',(2.66865995789381,2.7039333039484,-39.));
#32943=CARTESIAN_POINT('Ctrl Pts',(2.5771544005093,2.77562846691384,-39.));
#32944=CARTESIAN_POINT('Ctrl Pts',(2.48616555011133,2.84691878680019,-39.));
#32945=CARTESIAN_POINT('Ctrl Pts',(2.39189554495299,2.91370656208833,-39.));
#32946=CARTESIAN_POINT('Ctrl Pts',(2.29447234532102,2.97562460420606,-39.));
#32947=CARTESIAN_POINT('Ctrl Pts',(2.27139641425051,2.99029068453731,-39.));
#32948=CARTESIAN_POINT('Ctrl Pts',(2.24814347894285,3.0046833385606,-39.));
#32949=CARTESIAN_POINT('Ctrl Pts',(2.22471506914856,3.01879727283302,-39.));
#32950=CARTESIAN_POINT('Ctrl Pts',(2.12317225035552,3.07996952834948,-39.));
#32951=CARTESIAN_POINT('Ctrl Pts',(2.01833364786956,3.13591009017389,-39.));
#32952=CARTESIAN_POINT('Ctrl Pts',(1.91064248930382,3.18656524692859,-39.));
#32953=CARTESIAN_POINT('Ctrl Pts',(1.85027201234174,3.21496196969207,-39.));
#32954=CARTESIAN_POINT('Ctrl Pts',(1.78900493758425,3.24169676584405,-39.));
#32955=CARTESIAN_POINT('Ctrl Pts',(1.72691930409674,3.26675302213736,-39.));
#32956=CARTESIAN_POINT('Ctrl Pts',(1.7081799729301,3.2743157618261,-39.));
#32957=CARTESIAN_POINT('Ctrl Pts',(1.68936607397445,3.28172554844747,-39.));
#32958=CARTESIAN_POINT('Ctrl Pts',(1.67047976756002,3.28898183330933,-39.));
#32959=CARTESIAN_POINT('Ctrl Pts',(1.65401551208684,3.29530754491912,-39.));
#32960=CARTESIAN_POINT('Ctrl Pts',(1.63749558785105,3.30151676005302,-39.));
#32961=CARTESIAN_POINT('Ctrl Pts',(1.62093733317381,3.30760347428902,-39.));
#32962=CARTESIAN_POINT('Ctrl Pts',(1.51232751810485,3.34752778518023,-39.));
#32963=CARTESIAN_POINT('Ctrl Pts',(1.40192140847811,3.3822442337368,-39.));
#32964=CARTESIAN_POINT('Ctrl Pts',(1.29014212257712,3.41176730634751,-39.));
#32965=CARTESIAN_POINT('Ctrl Pts',(1.1774449041267,3.44153282270878,-39.));
#32966=CARTESIAN_POINT('Ctrl Pts',(1.06335174640429,3.46601902640531,-39.));
#32967=CARTESIAN_POINT('Ctrl Pts',(0.948291874745636,3.48518748998652,-39.));
#32968=CARTESIAN_POINT('Ctrl Pts',(0.834769919331161,3.50409974355208,-39.));
#32969=CARTESIAN_POINT('Ctrl Pts',(0.720306022442315,3.51783531415529,-39.));
#32970=CARTESIAN_POINT('Ctrl Pts',(0.605319480240082,3.52630781742824,-39.));
#32971=CARTESIAN_POINT('Ctrl Pts',(0.521444284469331,3.53248795692175,-39.));
#32972=CARTESIAN_POINT('Ctrl Pts',(0.437291099039107,3.53586672787097,-39.));
#32973=CARTESIAN_POINT('Ctrl Pts',(0.353029136599959,3.53639426684562,-39.));
#32974=CARTESIAN_POINT('Ctrl Pts',(0.327898163577327,3.53655160436016,-39.));
#32975=CARTESIAN_POINT('Ctrl Pts',(0.302757563702177,3.53645522658894,-39.));
#32976=CARTESIAN_POINT('Ctrl Pts',(0.277611962535154,3.53610357479034,-39.));
#32977=CARTESIAN_POINT('Ctrl Pts',(0.258741040287152,3.53583967202238,-39.));
#32978=CARTESIAN_POINT('Ctrl Pts',(0.239875829455418,3.53543209444648,-39.));
#32979=CARTESIAN_POINT('Ctrl Pts',(0.221022502202154,3.53488072125031,-39.));
#32980=CARTESIAN_POINT('Ctrl Pts',(0.107579683538356,3.53156304004373,-39.));
#32981=CARTESIAN_POINT('Ctrl Pts',(-0.00548437432396109,3.52304246054611,
-39.));
#32982=CARTESIAN_POINT('Ctrl Pts',(-0.117759280560823,3.50925106599073,
-39.));
#32983=CARTESIAN_POINT('Ctrl Pts',(-0.227468089891742,3.49577488038169,
-39.));
#32984=CARTESIAN_POINT('Ctrl Pts',(-0.336424125111459,3.47726582969332,
-39.));
#32985=CARTESIAN_POINT('Ctrl Pts',(-0.444223733781713,3.45361539240257,
-39.));
#32986=CARTESIAN_POINT('Ctrl Pts',(-0.469784016719349,3.44800765526691,
-39.));
#32987=CARTESIAN_POINT('Ctrl Pts',(-0.495279164302631,3.44211066994351,
-39.));
#32988=CARTESIAN_POINT('Ctrl Pts',(-0.520703552750254,3.43592262669056,
-39.));
#32989=CARTESIAN_POINT('Ctrl Pts',(-0.544842672211385,3.43004740512441,
-39.));
#32990=CARTESIAN_POINT('Ctrl Pts',(-0.568920339517025,3.42390906587648,
-39.));
#32991=CARTESIAN_POINT('Ctrl Pts',(-0.592909343325201,3.41751225292074,
-39.));
#32992=CARTESIAN_POINT('Ctrl Pts',(-0.696930171154229,3.38977447004135,
-39.));
#32993=CARTESIAN_POINT('Ctrl Pts',(-0.79937645949779,3.35715927661756,-39.));
#32994=CARTESIAN_POINT('Ctrl Pts',(-0.899875244423881,3.31958176012196,
-39.));
#32995=CARTESIAN_POINT('Ctrl Pts',(-0.994995238784878,3.28401542805347,
-39.));
#32996=CARTESIAN_POINT('Ctrl Pts',(-1.0883709659824,3.24400334859258,-39.));
#32997=CARTESIAN_POINT('Ctrl Pts',(-1.17966135005092,3.19943835339881,-39.));
#32998=CARTESIAN_POINT('Ctrl Pts',(-1.22188181501936,3.17882769612537,-39.));
#32999=CARTESIAN_POINT('Ctrl Pts',(-1.26365583302969,3.15724268359402,-39.));
#33000=CARTESIAN_POINT('Ctrl Pts',(-1.30496166320995,3.13470830288176,-39.));
#33001=CARTESIAN_POINT('Ctrl Pts',(2.57323442701465,2.20655152809233,-28.));
#33002=CARTESIAN_POINT('Ctrl Pts',(2.65146086060648,2.13210309013611,-28.));
#33003=CARTESIAN_POINT('Ctrl Pts',(2.72559006808564,2.05386847221022,-28.));
#33004=CARTESIAN_POINT('Ctrl Pts',(2.79562474081432,1.97228873410646,-28.));
#33005=CARTESIAN_POINT('Ctrl Pts',(2.8662200815952,1.89005590302633,-28.));
#33006=CARTESIAN_POINT('Ctrl Pts',(2.93265540757401,1.8044236111313,-28.));
#33007=CARTESIAN_POINT('Ctrl Pts',(2.99490662467184,1.71579430777158,-28.));
#33008=CARTESIAN_POINT('Ctrl Pts',(3.05871119030977,1.62495344606167,-28.));
#33009=CARTESIAN_POINT('Ctrl Pts',(3.11812071413516,1.5309636073814,-28.));
#33010=CARTESIAN_POINT('Ctrl Pts',(3.17307474355074,1.43421476081748,-28.));
#33011=CARTESIAN_POINT('Ctrl Pts',(3.22407555773482,1.34442571352461,-28.));
#33012=CARTESIAN_POINT('Ctrl Pts',(3.27123873365936,1.25225942026066,-28.));
#33013=CARTESIAN_POINT('Ctrl Pts',(3.31448495636522,1.15800209474407,-28.));
#33014=CARTESIAN_POINT('Ctrl Pts',(3.32156241408425,1.1425764183656,-28.));
#33015=CARTESIAN_POINT('Ctrl Pts',(3.32853559102356,1.12709311608126,-28.));
#33016=CARTESIAN_POINT('Ctrl Pts',(3.33540186900274,1.11155835104982,-28.));
#33017=CARTESIAN_POINT('Ctrl Pts',(3.38154819417809,1.00715355986056,-28.));
#33018=CARTESIAN_POINT('Ctrl Pts',(3.42271638561207,0.900775643276435,-28.));
#33019=CARTESIAN_POINT('Ctrl Pts',(3.45888174339864,0.79286061108879,-28.));
#33020=CARTESIAN_POINT('Ctrl Pts',(3.49551139265451,0.683560163909538,-28.));
#33021=CARTESIAN_POINT('Ctrl Pts',(3.52700936086568,0.572682160975876,-28.));
#33022=CARTESIAN_POINT('Ctrl Pts',(3.55331100085337,0.460641756070989,-28.));
#33023=CARTESIAN_POINT('Ctrl Pts',(3.57965805345284,0.348407901350266,-28.));
#33024=CARTESIAN_POINT('Ctrl Pts',(3.60079119852265,0.235006803316379,-28.));
#33025=CARTESIAN_POINT('Ctrl Pts',(3.61660057879941,0.12082976881976,-28.));
#33026=CARTESIAN_POINT('Ctrl Pts',(3.62981203276487,0.0254152358805882,
-28.));
#33027=CARTESIAN_POINT('Ctrl Pts',(3.63930497467244,-0.0705418771992364,
-28.));
#33028=CARTESIAN_POINT('Ctrl Pts',(3.64498836398506,-0.166820713555591,
-28.));
#33029=CARTESIAN_POINT('Ctrl Pts',(3.6461235777139,-0.186051677830032,-28.));
#33030=CARTESIAN_POINT('Ctrl Pts',(3.6471067185271,-0.20529548900737,-28.));
#33031=CARTESIAN_POINT('Ctrl Pts',(3.64793693432402,-0.224550399084413,
-28.));
#33032=CARTESIAN_POINT('Ctrl Pts',(3.64860254404802,-0.23998765699922,-28.));
#33033=CARTESIAN_POINT('Ctrl Pts',(3.64916964547777,-0.255427938226552,
-28.));
#33034=CARTESIAN_POINT('Ctrl Pts',(3.64963779664493,-0.270862333203369,
-28.));
#33035=CARTESIAN_POINT('Ctrl Pts',(3.65323277593957,-0.38938458468805,-28.));
#33036=CARTESIAN_POINT('Ctrl Pts',(3.65100280640831,-0.507698311102713,
-28.));
#33037=CARTESIAN_POINT('Ctrl Pts',(3.64288169923472,-0.625376302714804,
-28.));
#33038=CARTESIAN_POINT('Ctrl Pts',(3.63479002186308,-0.742627845086358,
-28.));
#33039=CARTESIAN_POINT('Ctrl Pts',(3.62085014760366,-0.859249136162332,
-28.));
#33040=CARTESIAN_POINT('Ctrl Pts',(3.60094836490086,-0.974834987561213,
-28.));
#33041=CARTESIAN_POINT('Ctrl Pts',(3.59783401431466,-0.992922556370264,
-28.));
#33042=CARTESIAN_POINT('Ctrl Pts',(3.59457356725438,-1.01098478869548,-28.));
#33043=CARTESIAN_POINT('Ctrl Pts',(3.59116647252837,-1.02902014863058,-28.));
#33044=CARTESIAN_POINT('Ctrl Pts',(3.5698067929562,-1.14208701062335,-28.));
#33045=CARTESIAN_POINT('Ctrl Pts',(3.54268787530998,-1.25409799710567,-28.));
#33046=CARTESIAN_POINT('Ctrl Pts',(3.51011097433732,-1.36479007515236,-28.));
#33047=CARTESIAN_POINT('Ctrl Pts',(3.48961584669467,-1.43442985674183,-28.));
#33048=CARTESIAN_POINT('Ctrl Pts',(3.46695931768047,-1.50354758632599,-28.));
#33049=CARTESIAN_POINT('Ctrl Pts',(3.44220601927238,-1.57207614745179,-28.));
#33050=CARTESIAN_POINT('Ctrl Pts',(3.43518503142662,-1.59151348411776,-28.));
#33051=CARTESIAN_POINT('Ctrl Pts',(3.42799530994855,-1.61090340968787,-28.));
#33052=CARTESIAN_POINT('Ctrl Pts',(3.42063822020598,-1.63024436076578,-28.));
#33053=CARTESIAN_POINT('Ctrl Pts',(3.41481803847106,-1.64554495572091,-28.));
#33054=CARTESIAN_POINT('Ctrl Pts',(3.40889428943117,-1.6608116772918,-28.));
#33055=CARTESIAN_POINT('Ctrl Pts',(3.40287157324905,-1.67603450368239,-28.));
#33056=CARTESIAN_POINT('Ctrl Pts',(3.35899814626558,-1.7869275861277,-28.));
#33057=CARTESIAN_POINT('Ctrl Pts',(3.30982303933651,-1.89563557342822,-28.));
#33058=CARTESIAN_POINT('Ctrl Pts',(3.25572869869663,-2.0018849375163,-28.));
#33059=CARTESIAN_POINT('Ctrl Pts',(3.20129011712566,-2.10881044220593,-28.));
#33060=CARTESIAN_POINT('Ctrl Pts',(3.1418691079394,-2.21324660722471,-28.));
#33061=CARTESIAN_POINT('Ctrl Pts',(3.07779972161007,-2.31491110313074,-28.));
#33062=CARTESIAN_POINT('Ctrl Pts',(3.01270127986138,-2.41820849122544,-28.));
#33063=CARTESIAN_POINT('Ctrl Pts',(2.94280360348117,-2.51864522862981,-28.));
#33064=CARTESIAN_POINT('Ctrl Pts',(2.86840510375314,-2.61591053169999,-28.));
#33065=CARTESIAN_POINT('Ctrl Pts',(2.79774779990573,-2.70828476099175,-28.));
#33066=CARTESIAN_POINT('Ctrl Pts',(2.72303020373738,-2.79779894671307,-28.));
#33067=CARTESIAN_POINT('Ctrl Pts',(2.64447016582119,-2.88416524587393,-28.));
#33068=CARTESIAN_POINT('Ctrl Pts',(2.63081639884696,-2.89917574427043,-28.));
#33069=CARTESIAN_POINT('Ctrl Pts',(2.6170454616123,-2.91409207965698,-28.));
#33070=CARTESIAN_POINT('Ctrl Pts',(2.60317113657109,-2.92889936528399,-28.));
#33071=CARTESIAN_POINT('Ctrl Pts',(2.51751513814057,-3.02031518772295,-28.));
#33072=CARTESIAN_POINT('Ctrl Pts',(2.42781771358721,-3.10769309042211,-28.));
#33073=CARTESIAN_POINT('Ctrl Pts',(2.33441120260619,-3.19071846015963,-28.));
#33074=CARTESIAN_POINT('Ctrl Pts',(2.24083730371898,-3.27389261441609,-28.));
#33075=CARTESIAN_POINT('Ctrl Pts',(2.14354049917036,-3.35269940049145,-28.));
#33076=CARTESIAN_POINT('Ctrl Pts',(2.04281067096056,-3.42679563159201,-28.));
#33077=CARTESIAN_POINT('Ctrl Pts',(2.01620424429062,-3.44636715250426,-28.));
#33078=CARTESIAN_POINT('Ctrl Pts',(1.98935808664189,-3.46560984606407,-28.));
#33079=CARTESIAN_POINT('Ctrl Pts',(1.96227709625951,-3.4845169684059,-28.));
#33080=CARTESIAN_POINT('Ctrl Pts',(1.94383437408304,-3.49739311508973,-28.));
#33081=CARTESIAN_POINT('Ctrl Pts',(1.92528081035815,-3.51011491576498,-28.));
#33082=CARTESIAN_POINT('Ctrl Pts',(1.90662413024797,-3.52267600831012,-28.));
#33083=CARTESIAN_POINT('Ctrl Pts',(1.79806977795192,-3.59576303436816,-28.));
#33084=CARTESIAN_POINT('Ctrl Pts',(1.68620253668162,-3.66329638779482,-28.));
#33085=CARTESIAN_POINT('Ctrl Pts',(1.57136880162434,-3.72490971212853,-28.));
#33086=CARTESIAN_POINT('Ctrl Pts',(1.45653506656706,-3.78652303646223,-28.));
#33087=CARTESIAN_POINT('Ctrl Pts',(1.33873418968137,-3.84221725159107,-28.));
#33088=CARTESIAN_POINT('Ctrl Pts',(1.21827111413391,-3.89158314773214,-28.));
#33089=CARTESIAN_POINT('Ctrl Pts',(1.166391910295,-3.91284330049641,-28.));
#33090=CARTESIAN_POINT('Ctrl Pts',(1.11401847832268,-3.93292910513849,-28.));
#33091=CARTESIAN_POINT('Ctrl Pts',(1.06118740155668,-3.95185074745288,-28.));
#33092=CARTESIAN_POINT('Ctrl Pts',(-1.05882113085931,-3.94905752896967,
-28.0020436944626));
#33093=CARTESIAN_POINT('Ctrl Pts',(-2.35950680140507,-3.60031774422942,
-28.0675689977652));
#33094=CARTESIAN_POINT('Ctrl Pts',(-4.5680262281043,-1.52377528117773,-28.1986196043704));
#33095=CARTESIAN_POINT('Ctrl Pts',(-3.78535991995299,2.98379941052452,-28.3951955142783));
#33096=CARTESIAN_POINT('Ctrl Pts',(0.408199144658901,4.79866122549394,-28.5917714241861));
#33097=CARTESIAN_POINT('Ctrl Pts',(4.23151248292971,2.30176772412023,-28.7883473340939));
#33098=CARTESIAN_POINT('Ctrl Pts',(4.25039471757788,-2.26763872001778,-28.9849232440017));
#33099=CARTESIAN_POINT('Ctrl Pts',(0.445491442266795,-4.79631292568449,
-29.1814991539096));
#33100=CARTESIAN_POINT('Ctrl Pts',(-3.75969845785261,-3.01155046772413,
-29.3780750638174));
#33101=CARTESIAN_POINT('Ctrl Pts',(-4.58346317448722,1.48221938381933,-29.5746509737252));
#33102=CARTESIAN_POINT('Ctrl Pts',(-1.28456058010556,4.64266995936712,-29.7712268836331));
#33103=CARTESIAN_POINT('Ctrl Pts',(3.16967659691989,3.62738124137317,-29.9678027935409));
#33104=CARTESIAN_POINT('Ctrl Pts',(4.7729992922858,-0.650566816687759,-30.1643787034487));
#33105=CARTESIAN_POINT('Ctrl Pts',(2.08326953584618,-4.34334784652524,-30.3609546133566));
#33106=CARTESIAN_POINT('Ctrl Pts',(-2.48023430202747,-4.12954713239435,
-30.5575305232643));
#33107=CARTESIAN_POINT('Ctrl Pts',(-4.81291358150149,-0.201451079063452,
-30.7541064331722));
#33108=CARTESIAN_POINT('Ctrl Pts',(-2.81665191682384,3.90783605333626,-30.9506823430801));
#33109=CARTESIAN_POINT('Ctrl Pts',(1.71302529420149,4.50225061230501,-31.1472582529878));
#33110=CARTESIAN_POINT('Ctrl Pts',(4.70193520370772,1.04714888338313,-31.3438341628957));
#33111=CARTESIAN_POINT('Ctrl Pts',(3.46172444128033,-3.34980272978597,-31.5404100728035));
#33112=CARTESIAN_POINT('Ctrl Pts',(-0.892108337079269,-4.73379952267849,
-31.7369859827114));
#33113=CARTESIAN_POINT('Ctrl Pts',(-4.44354101170039,-1.86001567550251,
-31.9335618926191));
#33114=CARTESIAN_POINT('Ctrl Pts',(-3.99826394800999,2.68674530490854,-32.1301378025271));
#33115=CARTESIAN_POINT('Ctrl Pts',(0.043221683045428,4.81693335226694,-32.3267137124348));
#33116=CARTESIAN_POINT('Ctrl Pts',(4.04583190312332,2.6145667356681,-32.5232896223427));
#33117=CARTESIAN_POINT('Ctrl Pts',(4.4094488939688,-1.93945235711869,-32.7198655322504));
#33118=CARTESIAN_POINT('Ctrl Pts',(0.807020081006245,-4.74904554580652,
-32.9164414421584));
#33119=CARTESIAN_POINT('Ctrl Pts',(-3.52127690491969,-3.28714526013178,
-33.1130173520661));
#33120=CARTESIAN_POINT('Ctrl Pts',(-4.68238773251868,1.13135322695175,-33.309593261974));
#33121=CARTESIAN_POINT('Ctrl Pts',(-1.63195995882842,4.53226452184925,-33.5061691718818));
#33122=CARTESIAN_POINT('Ctrl Pts',(2.8863219858102,3.85666441328645,-33.7027450817896));
#33123=CARTESIAN_POINT('Ctrl Pts',(4.80852322250443,-0.287783637249186,
-33.8993209916975));
#33124=CARTESIAN_POINT('Ctrl Pts',(2.40573423502515,-4.17338684909552,-34.0958969016053));
#33125=CARTESIAN_POINT('Ctrl Pts',(-2.16087440442547,-4.30526849460362,
-34.2924728115131));
#33126=CARTESIAN_POINT('Ctrl Pts',(-4.78390073438757,-0.564808614327262,
-34.4890487214209));
#33127=CARTESIAN_POINT('Ctrl Pts',(-3.10408335123885,3.68366414628393,-34.6856246313288));
#33128=CARTESIAN_POINT('Ctrl Pts',(1.36767856671707,4.61889276144569,-34.8822005412366));
#33129=CARTESIAN_POINT('Ctrl Pts',(4.60929224090002,1.39969284918004,-35.0787764511445));
#33130=CARTESIAN_POINT('Ctrl Pts',(3.70511249281298,-3.07845031582542,-35.2753523610522));
#33131=CARTESIAN_POINT('Ctrl Pts',(-0.531602930013868,-4.78770439360861,
-35.4719282709601));
#33132=CARTESIAN_POINT('Ctrl Pts',(-4.29017212852273,-2.19069356908814,
-35.6685041808679));
#33133=CARTESIAN_POINT('Ctrl Pts',(-4.1899780121579,2.3767201546401,-35.8650800907758));
#33134=CARTESIAN_POINT('Ctrl Pts',(-0.32113973386512,4.8064107934268,-36.0616560006836));
#33135=CARTESIAN_POINT('Ctrl Pts',(3.83654567111785,2.91301107927893,-36.2582319105914));
#33136=CARTESIAN_POINT('Ctrl Pts',(4.54347800750842,-1.60047437829833,-36.4548078204993));
#33137=CARTESIAN_POINT('Ctrl Pts',(1.16381458360049,-4.67442566474814,-36.6513837304071));
#33138=CARTESIAN_POINT('Ctrl Pts',(-3.2626361586303,-3.54399873137932,-36.8479596403149));
#33139=CARTESIAN_POINT('Ctrl Pts',(-4.75452733360971,0.774049293558451,
-37.0445355502227));
#33140=CARTESIAN_POINT('Ctrl Pts',(-1.97000605283459,4.39588848572516,-37.2411114601306));
#33141=CARTESIAN_POINT('Ctrl Pts',(2.58644514433784,4.0638708043759,-37.4376873700384));
#33142=CARTESIAN_POINT('Ctrl Pts',(4.81649301369077,0.0766504053415182,
-37.6342632799463));
#33143=CARTESIAN_POINT('Ctrl Pts',(2.71446985731166,-3.9795429847404,-37.830839189854));
#33144=CARTESIAN_POINT('Ctrl Pts',(-1.82923482333114,-4.45630661812464,
-38.0274150997619));
#33145=CARTESIAN_POINT('Ctrl Pts',(-4.72731037414528,-0.924995639297582,
-38.2239910096697));
#33146=CARTESIAN_POINT('Ctrl Pts',(-3.37410476784824,3.43852550307855,-38.4205669195776));
#33147=CARTESIAN_POINT('Ctrl Pts',(1.01521569000634,4.70883952282901,-38.6171428294853));
#33148=CARTESIAN_POINT('Ctrl Pts',(4.48884927255114,1.74470865965533,-38.8137187393932));
#33149=CARTESIAN_POINT('Ctrl Pts',(3.93008090951081,-2.7904251809593,-39.010294649301));
#33150=CARTESIAN_POINT('Ctrl Pts',(-0.174843701399625,-4.81279159986601,
-39.2069155208212));
#33151=CARTESIAN_POINT('Ctrl Pts',(-2.79071673421448,-3.27789123761485,
-39.3380110890387));
#33152=CARTESIAN_POINT('Ctrl Pts',(-3.49170722037164,-2.12700203220468,
-39.4035813539536));
#33153=CARTESIAN_POINT('Ctrl Pts',(-0.997991714641228,-3.72218364338343,
-27.8664315295235));
#33154=CARTESIAN_POINT('Ctrl Pts',(-2.22395281866996,-3.3934790061289,-27.9319568328261));
#33155=CARTESIAN_POINT('Ctrl Pts',(-4.30559250759574,-1.43623418655831,
-28.0630074394313));
#33156=CARTESIAN_POINT('Ctrl Pts',(-3.56789048399717,2.81237973352319,-28.2595833493392));
#33157=CARTESIAN_POINT('Ctrl Pts',(0.384748048957611,4.52297749340006,-28.456159259247));
#33158=CARTESIAN_POINT('Ctrl Pts',(3.98841152229129,2.16953085913224,-28.6527351691548));
#33159=CARTESIAN_POINT('Ctrl Pts',(4.00620897002213,-2.13736257090065,-28.8493110790626));
#33160=CARTESIAN_POINT('Ctrl Pts',(0.419897899057805,-4.52076410373015,
-29.0458869889705));
#33161=CARTESIAN_POINT('Ctrl Pts',(-3.54370327634202,-2.8385364887584,-29.2424628988783));
#33162=CARTESIAN_POINT('Ctrl Pts',(-4.32014259933502,1.39706568108611,-29.4390388087861));
#33163=CARTESIAN_POINT('Ctrl Pts',(-1.21076240220069,4.37594794646929,-29.635614718694));
#33164=CARTESIAN_POINT('Ctrl Pts',(2.98757825058798,3.41898770172583,-29.8321906286018));
#33165=CARTESIAN_POINT('Ctrl Pts',(4.49878984170234,-0.613191665666869,
-30.0287665385096));
#33166=CARTESIAN_POINT('Ctrl Pts',(1.96358542112927,-4.09382192922343,-30.2253424484175));
#33167=CARTESIAN_POINT('Ctrl Pts',(-2.33774450816214,-3.892304094843,-30.4219183583252));
#33168=CARTESIAN_POINT('Ctrl Pts',(-4.53641104964019,-0.189877687506765,
-30.6184942682331));
#33169=CARTESIAN_POINT('Ctrl Pts',(-2.6548348857915,3.68333034706318,-30.8150701781409));
#33170=CARTESIAN_POINT('Ctrl Pts',(1.61461176090855,4.24359570976092,-31.0116460880488));
#33171=CARTESIAN_POINT('Ctrl Pts',(4.43180839456038,0.986990039350689,-31.2082219979566));
#33172=CARTESIAN_POINT('Ctrl Pts',(3.26284790705395,-3.15735611292137,-31.4047979078644));
#33173=CARTESIAN_POINT('Ctrl Pts',(-0.840856593261335,-4.46184210412537,
-31.6013738177723));
#33174=CARTESIAN_POINT('Ctrl Pts',(-4.18825898359853,-1.753157525056,-31.7979497276801));
#33175=CARTESIAN_POINT('Ctrl Pts',(-3.76856314703911,2.53239142618341,-31.9945256375879));
#33176=CARTESIAN_POINT('Ctrl Pts',(0.0407385915477348,4.54019988403512,
-32.1911015474957));
#33177=CARTESIAN_POINT('Ctrl Pts',(3.81339831674055,2.46435952544285,-32.3876774574036));
#33178=CARTESIAN_POINT('Ctrl Pts',(4.15612546261083,-1.82803055864119,-32.5842533673114));
#33179=CARTESIAN_POINT('Ctrl Pts',(0.760656668931118,-4.47621224117645,
-32.7808292772193));
#33180=CARTESIAN_POINT('Ctrl Pts',(-3.31897907365649,-3.0982983233167,-32.977405187127));
#33181=CARTESIAN_POINT('Ctrl Pts',(-4.41338392821731,1.06635683206863,-33.1739810970349));
#33182=CARTESIAN_POINT('Ctrl Pts',(-1.53820363994361,4.27188531616954,-33.3705570069427));
#33183=CARTESIAN_POINT('Ctrl Pts',(2.72050239995459,3.63509852460902,-33.5671329168505));
#33184=CARTESIAN_POINT('Ctrl Pts',(4.53227291735735,-0.27125042862614,-33.7637088267584));
#33185=CARTESIAN_POINT('Ctrl Pts',(2.26752448001801,-3.93362521392992,-33.9602847366662));
#33186=CARTESIAN_POINT('Ctrl Pts',(-2.03673187958264,-4.05793024118558,
-34.156860646574));
#33187=CARTESIAN_POINT('Ctrl Pts',(-4.50906499449078,-0.532360283553406,
-34.3534365564819));
#33188=CARTESIAN_POINT('Ctrl Pts',(-2.92575334568362,3.472037146188,-34.5500124663897));
#33189=CARTESIAN_POINT('Ctrl Pts',(1.28910524931466,4.35353675176285,-34.7465883762975));
#33190=CARTESIAN_POINT('Ctrl Pts',(4.34448778241235,1.31928030694909,-34.9431642862054));
#33191=CARTESIAN_POINT('Ctrl Pts',(3.49225328232741,-2.90159293159843,-35.1397401961131));
#33192=CARTESIAN_POINT('Ctrl Pts',(-0.501062270264922,-4.51265013297856,
-35.336316106021));
#33193=CARTESIAN_POINT('Ctrl Pts',(-4.0437011633642,-2.0648379292293,-35.5328920159288));
#33194=CARTESIAN_POINT('Ctrl Pts',(-3.94926321244538,2.24017726244907,-35.7294679258367));
#33195=CARTESIAN_POINT('Ctrl Pts',(-0.302690213010174,4.53028184761403,
-35.9260438357445));
#33196=CARTESIAN_POINT('Ctrl Pts',(3.61613560688092,2.74565820141793,-36.1226197456523));
#33197=CARTESIAN_POINT('Ctrl Pts',(4.28245458557109,-1.50852691024499,-36.3191956555602));
#33198=CARTESIAN_POINT('Ctrl Pts',(1.09695327941679,-4.40587928230987,-36.515771565468));
#33199=CARTESIAN_POINT('Ctrl Pts',(-3.07519727298922,-3.34039552813339,
-36.7123474753758));
#33200=CARTESIAN_POINT('Ctrl Pts',(-4.48137909953387,0.729580057651749,
-36.9089233852837));
#33201=CARTESIAN_POINT('Ctrl Pts',(-1.8568289404334,4.1433441016426,-37.1054992951915));
#33202=CARTESIAN_POINT('Ctrl Pts',(2.4378535233126,3.83040088069267,-37.3020752050993));
#33203=CARTESIAN_POINT('Ctrl Pts',(4.53978484296931,0.0722468292568363,
-37.4986511150071));
#33204=CARTESIAN_POINT('Ctrl Pts',(2.55852319932624,-3.75091770562448,-37.695227024915));
#33205=CARTESIAN_POINT('Ctrl Pts',(-1.72414503697722,-4.20029120421869,
-37.8918029348228));
#33206=CARTESIAN_POINT('Ctrl Pts',(-4.4557257580472,-0.871854515548868,
-38.0883788447306));
#33207=CARTESIAN_POINT('Ctrl Pts',(-3.18026199563204,3.24098175096857,-38.2849547546384));
#33208=CARTESIAN_POINT('Ctrl Pts',(0.956891412223545,4.43831605962057,-38.4815306645463));
#33209=CARTESIAN_POINT('Ctrl Pts',(4.23096427877636,1.64447491276048,-38.6781065744541));
#33210=CARTESIAN_POINT('Ctrl Pts',(3.70429723326195,-2.63011487942588,-38.8746824843619));
#33211=CARTESIAN_POINT('Ctrl Pts',(-0.164798907264359,-4.53629607586606,
-39.0713033558821));
#33212=CARTESIAN_POINT('Ctrl Pts',(-2.63038968290739,-3.08957594563662,
-39.2023989240996));
#33213=CARTESIAN_POINT('Ctrl Pts',(-3.29110817145834,-2.00480547969662,
-39.2679691890145));
#33214=CARTESIAN_POINT('Ctrl Pts',(-0.937162298423141,-3.49530975779719,
-27.7308193645844));
#33215=CARTESIAN_POINT('Ctrl Pts',(-2.08839883593485,-3.18664026802839,
-27.796344667887));
#33216=CARTESIAN_POINT('Ctrl Pts',(-4.04315878708718,-1.34869309193889,
-27.9273952744922));
#33217=CARTESIAN_POINT('Ctrl Pts',(-3.35042104804134,2.64096005652187,-28.1239711844001));
#33218=CARTESIAN_POINT('Ctrl Pts',(0.361296953256328,4.24729376130616,-28.3205470943079));
#33219=CARTESIAN_POINT('Ctrl Pts',(3.74531056165287,2.03729399414426,-28.5171230042157));
#33220=CARTESIAN_POINT('Ctrl Pts',(3.76202322246639,-2.0070864217835,-28.7136989141235));
#33221=CARTESIAN_POINT('Ctrl Pts',(0.39430435584881,-4.2452152817758,-28.9102748240314));
#33222=CARTESIAN_POINT('Ctrl Pts',(-3.32770809483142,-2.66552250979267,
-29.1068507339392));
#33223=CARTESIAN_POINT('Ctrl Pts',(-4.05682202418285,1.31191197835287,-29.303426643847));
#33224=CARTESIAN_POINT('Ctrl Pts',(-1.13696422429583,4.10922593357146,-29.5000025537548));
#33225=CARTESIAN_POINT('Ctrl Pts',(2.80547990425606,3.2105941620785,-29.6965784636627));
#33226=CARTESIAN_POINT('Ctrl Pts',(4.22458039111889,-0.575816514645981,
-29.8931543735705));
#33227=CARTESIAN_POINT('Ctrl Pts',(1.84390130641238,-3.84429601192161,-30.0897302834784));
#33228=CARTESIAN_POINT('Ctrl Pts',(-2.1952547142968,-3.65506105729165,-30.2863061933862));
#33229=CARTESIAN_POINT('Ctrl Pts',(-4.2599085177789,-0.178304295950073,
-30.482882103294));
#33230=CARTESIAN_POINT('Ctrl Pts',(-2.49301785475917,3.4588246407901,-30.6794580132018));
#33231=CARTESIAN_POINT('Ctrl Pts',(1.51619822761561,3.98494080721683,-30.8760339231097));
#33232=CARTESIAN_POINT('Ctrl Pts',(4.16168158541303,0.926831195318249,-31.0726098330175));
#33233=CARTESIAN_POINT('Ctrl Pts',(3.06397137282756,-2.96490949605675,-31.2691857429253));
#33234=CARTESIAN_POINT('Ctrl Pts',(-0.789604849443395,-4.18988468557226,
-31.4657616528332));
#33235=CARTESIAN_POINT('Ctrl Pts',(-3.93297695549669,-1.6462993746095,-31.662337562741));
#33236=CARTESIAN_POINT('Ctrl Pts',(-3.53886234606824,2.37803754745827,-31.8589134726488));
#33237=CARTESIAN_POINT('Ctrl Pts',(0.0382555000500392,4.26346641580331,
-32.0554893825566));
#33238=CARTESIAN_POINT('Ctrl Pts',(3.58096473035777,2.3141523152176,-32.2520652924645));
#33239=CARTESIAN_POINT('Ctrl Pts',(3.90280203125285,-1.71660876016369,-32.4486412023723));
#33240=CARTESIAN_POINT('Ctrl Pts',(0.714293256855994,-4.20337893654636,
-32.6452171122801));
#33241=CARTESIAN_POINT('Ctrl Pts',(-3.11668124239328,-2.90945138650161,
-32.8417930221879));
#33242=CARTESIAN_POINT('Ctrl Pts',(-4.14438012391592,1.00136043718551,-33.0383689320958));
#33243=CARTESIAN_POINT('Ctrl Pts',(-1.44444732105879,4.01150611048984,-33.2349448420036));
#33244=CARTESIAN_POINT('Ctrl Pts',(2.55468281409898,3.4135326359316,-33.4315207519115));
#33245=CARTESIAN_POINT('Ctrl Pts',(4.25602261221028,-0.254717220003096,
-33.6280966618193));
#33246=CARTESIAN_POINT('Ctrl Pts',(2.12931472501088,-3.69386357876432,-33.8246725717271));
#33247=CARTESIAN_POINT('Ctrl Pts',(-1.91258935473982,-3.81059198776754,
-34.0212484816349));
#33248=CARTESIAN_POINT('Ctrl Pts',(-4.23422925459399,-0.499911952779544,
-34.2178243915428));
#33249=CARTESIAN_POINT('Ctrl Pts',(-2.74742334012838,3.26041014609205,-34.4144003014506));
#33250=CARTESIAN_POINT('Ctrl Pts',(1.21053193191224,4.08818074208003,-34.6109762113584));
#33251=CARTESIAN_POINT('Ctrl Pts',(4.07968332392467,1.23886776471814,-34.8075521212663));
#33252=CARTESIAN_POINT('Ctrl Pts',(3.27939407184185,-2.72473554737144,-35.0041280311741));
#33253=CARTESIAN_POINT('Ctrl Pts',(-0.470521610515976,-4.23759587234851,
-35.2007039410819));
#33254=CARTESIAN_POINT('Ctrl Pts',(-3.79723019820567,-1.93898228937048,
-35.3972798509897));
#33255=CARTESIAN_POINT('Ctrl Pts',(-3.70854841273286,2.10363437025803,-35.5938557608975));
#33256=CARTESIAN_POINT('Ctrl Pts',(-0.284240692155229,4.25415290180127,
-35.7904316708054));
#33257=CARTESIAN_POINT('Ctrl Pts',(3.39572554264398,2.57830532355692,-35.9870075807132));
#33258=CARTESIAN_POINT('Ctrl Pts',(4.02143116363375,-1.41657944219165,-36.1835834906211));
#33259=CARTESIAN_POINT('Ctrl Pts',(1.03009197523309,-4.13733289987159,-36.3801594005289));
#33260=CARTESIAN_POINT('Ctrl Pts',(-2.88775838734814,-3.13679232488744,
-36.5767353104367));
#33261=CARTESIAN_POINT('Ctrl Pts',(-4.20823086545802,0.685110821745049,
-36.7733112203445));
#33262=CARTESIAN_POINT('Ctrl Pts',(-1.74365182803221,3.89079971756003,-36.9698871302524));
#33263=CARTESIAN_POINT('Ctrl Pts',(2.28926190228734,3.59693095700945,-37.1664630401602));
#33264=CARTESIAN_POINT('Ctrl Pts',(4.26307667224786,0.0678432531721597,
-37.363038950068));
#33265=CARTESIAN_POINT('Ctrl Pts',(2.40257654134081,-3.52229242650857,-37.5596148599759));
#33266=CARTESIAN_POINT('Ctrl Pts',(-1.61905525062328,-3.94427579031274,
-37.7561907698837));
#33267=CARTESIAN_POINT('Ctrl Pts',(-4.18414114194912,-0.818713391800153,
-37.9527666797915));
#33268=CARTESIAN_POINT('Ctrl Pts',(-2.98641922341583,3.0434379988586,-38.1493425896994));
#33269=CARTESIAN_POINT('Ctrl Pts',(0.898567134440758,4.16779259641213,-38.3459184996071));
#33270=CARTESIAN_POINT('Ctrl Pts',(3.97307928500157,1.54424116586562,-38.542494409515));
#33271=CARTESIAN_POINT('Ctrl Pts',(3.47851355701309,-2.46980457789247,-38.7390703194228));
#33272=CARTESIAN_POINT('Ctrl Pts',(-0.154754113129096,-4.25980055186612,
-38.935691190943));
#33273=CARTESIAN_POINT('Ctrl Pts',(-2.47006263160031,-2.90126065365839,
-39.0667867591605));
#33274=CARTESIAN_POINT('Ctrl Pts',(-3.09050912254503,-1.88260892718855,
-39.1323570240753));
#33275=CARTESIAN_POINT('Ctrl Pts',(-0.876332882205054,-3.26843587221096,
-27.5952071996452));
#33276=CARTESIAN_POINT('Ctrl Pts',(-1.95284485319974,-2.97980152992788,
-27.6607325029478));
#33277=CARTESIAN_POINT('Ctrl Pts',(-3.78072506657861,-1.26115199731948,
-27.791783109553));
#33278=CARTESIAN_POINT('Ctrl Pts',(-3.13295161208552,2.46954037952055,-27.9883590194609));
#33279=CARTESIAN_POINT('Ctrl Pts',(0.337845857555048,3.97161002921227,-28.1849349293687));
#33280=CARTESIAN_POINT('Ctrl Pts',(3.50220960101444,1.90505712915628,-28.3815108392765));
#33281=CARTESIAN_POINT('Ctrl Pts',(3.51783747491063,-1.87681027266635,-28.5780867491843));
#33282=CARTESIAN_POINT('Ctrl Pts',(0.368710812639818,-3.96966645982145,
-28.7746626590923));
#33283=CARTESIAN_POINT('Ctrl Pts',(-3.11171291332083,-2.49250853082694,
-28.971238569));
#33284=CARTESIAN_POINT('Ctrl Pts',(-3.79350144903066,1.22675827561963,-29.1678144789079));
#33285=CARTESIAN_POINT('Ctrl Pts',(-1.06316604639096,3.84250392067363,-29.3643903888156));
#33286=CARTESIAN_POINT('Ctrl Pts',(2.62338155792415,3.00220062243116,-29.5609662987235));
#33287=CARTESIAN_POINT('Ctrl Pts',(3.95037094053543,-0.538441363625094,
-29.7575422086313));
#33288=CARTESIAN_POINT('Ctrl Pts',(1.72421719169547,-3.5947700946198,-29.9541181185392));
#33289=CARTESIAN_POINT('Ctrl Pts',(-2.05276492043147,-3.4178180197403,-30.1506940284469));
#33290=CARTESIAN_POINT('Ctrl Pts',(-3.98340598591762,-0.166730904393382,
-30.3472699383548));
#33291=CARTESIAN_POINT('Ctrl Pts',(-2.33120082372684,3.23431893451701,-30.5438458482627));
#33292=CARTESIAN_POINT('Ctrl Pts',(1.41778469432266,3.72628590467274,-30.7404217581705));
#33293=CARTESIAN_POINT('Ctrl Pts',(3.89155477626569,0.866672351285809,-30.9369976680783));
#33294=CARTESIAN_POINT('Ctrl Pts',(2.86509483860116,-2.77246287919215,-31.1335735779861));
#33295=CARTESIAN_POINT('Ctrl Pts',(-0.738353105625458,-3.91792726701915,
-31.3301494878941));
#33296=CARTESIAN_POINT('Ctrl Pts',(-3.67769492739484,-1.53944122416299,
-31.5267253978018));
#33297=CARTESIAN_POINT('Ctrl Pts',(-3.30916154509737,2.22368366873312,-31.7233013077096));
#33298=CARTESIAN_POINT('Ctrl Pts',(0.0357724085523446,3.9867329475715,-31.9198772176174));
#33299=CARTESIAN_POINT('Ctrl Pts',(3.34853114397498,2.16394510499236,-32.1164531275253));
#33300=CARTESIAN_POINT('Ctrl Pts',(3.64947859989488,-1.60518696168619,-32.3130290374331));
#33301=CARTESIAN_POINT('Ctrl Pts',(0.667929844780863,-3.93054563191626,
-32.5096049473409));
#33302=CARTESIAN_POINT('Ctrl Pts',(-2.91438341113007,-2.72060444968652,
-32.7061808572487));
#33303=CARTESIAN_POINT('Ctrl Pts',(-3.87537631961455,0.936364042302392,
-32.9027567671566));
#33304=CARTESIAN_POINT('Ctrl Pts',(-1.35069100217398,3.75112690481014,-33.0993326770644));
#33305=CARTESIAN_POINT('Ctrl Pts',(2.38886322824336,3.19196674725417,-33.2959085869722));
#33306=CARTESIAN_POINT('Ctrl Pts',(3.97977230706319,-0.238184011380052,
-33.4924844968801));
#33307=CARTESIAN_POINT('Ctrl Pts',(1.99110497000374,-3.45410194359872,-33.6890604067879));
#33308=CARTESIAN_POINT('Ctrl Pts',(-1.788446829897,-3.56325373434949,-33.8856363166957));
#33309=CARTESIAN_POINT('Ctrl Pts',(-3.9593935146972,-0.467463622005686,
-34.0822122266036));
#33310=CARTESIAN_POINT('Ctrl Pts',(-2.56909333457314,3.04878314599611,-34.2787881365114));
#33311=CARTESIAN_POINT('Ctrl Pts',(1.13195861450983,3.8228247323972,-34.4753640464193));
#33312=CARTESIAN_POINT('Ctrl Pts',(3.814878865437,1.15845522248718,-34.671939956327));
#33313=CARTESIAN_POINT('Ctrl Pts',(3.06653486135627,-2.54787816314444,-34.8685158662349));
#33314=CARTESIAN_POINT('Ctrl Pts',(-0.439980950767031,-3.96254161171846,
-35.0650917761427));
#33315=CARTESIAN_POINT('Ctrl Pts',(-3.55075923304713,-1.81312664951164,
-35.2616676860505));
#33316=CARTESIAN_POINT('Ctrl Pts',(-3.46783361302034,1.96709147806698,-35.4582435959584));
#33317=CARTESIAN_POINT('Ctrl Pts',(-0.265791171300281,3.9780239559885,-35.6548195058662));
#33318=CARTESIAN_POINT('Ctrl Pts',(3.17531547840704,2.4109524456959,-35.851395415774));
#33319=CARTESIAN_POINT('Ctrl Pts',(3.76040774169642,-1.3246319741383,-36.0479713256819));
#33320=CARTESIAN_POINT('Ctrl Pts',(0.96323067104939,-3.86878651743331,-36.2445472355897));
#33321=CARTESIAN_POINT('Ctrl Pts',(-2.70031950170705,-2.93318912164151,
-36.4411231454975));
#33322=CARTESIAN_POINT('Ctrl Pts',(-3.93508263138217,0.640641585838348,
-36.6376990554053));
#33323=CARTESIAN_POINT('Ctrl Pts',(-1.63047471563101,3.63825533347747,-36.8342749653132));
#33324=CARTESIAN_POINT('Ctrl Pts',(2.14067028126209,3.36346103332622,-37.030850875221));
#33325=CARTESIAN_POINT('Ctrl Pts',(3.98636850152641,0.0634396770874798,
-37.2274267851288));
#33326=CARTESIAN_POINT('Ctrl Pts',(2.24662988335538,-3.29366714739265,-37.4240026950367));
#33327=CARTESIAN_POINT('Ctrl Pts',(-1.51396546426936,-3.68826037640678,
-37.6205786049445));
#33328=CARTESIAN_POINT('Ctrl Pts',(-3.91255652585104,-0.765572268051441,
-37.8171545148523));
#33329=CARTESIAN_POINT('Ctrl Pts',(-2.79257645119962,2.84589424674863,-38.0137304247602));
#33330=CARTESIAN_POINT('Ctrl Pts',(0.840242856657966,3.89726913320368,-38.210306334668));
#33331=CARTESIAN_POINT('Ctrl Pts',(3.71519429122678,1.44400741897077,-38.4068822445758));
#33332=CARTESIAN_POINT('Ctrl Pts',(3.25272988076424,-2.30949427635907,-38.6034581544836));
#33333=CARTESIAN_POINT('Ctrl Pts',(-0.144709318993833,-3.98330502786617,
-38.8000790260038));
#33334=CARTESIAN_POINT('Ctrl Pts',(-2.30973558029321,-2.71294536168015,
-38.9311745942213));
#33335=CARTESIAN_POINT('Ctrl Pts',(-2.88991007363174,-1.7604123746805,-38.9967448591362));
#33336=CARTESIAN_POINT('Ctrl Pts',(-2.89372837779135,-1.76542944862293,
-39.));
#33337=CARTESIAN_POINT('Ctrl Pts',(-2.84709705329411,-1.86283293579633,
-39.));
#33338=CARTESIAN_POINT('Ctrl Pts',(-2.79559872548623,-1.95750971474293,
-39.));
#33339=CARTESIAN_POINT('Ctrl Pts',(-2.73965370343092,-2.04932605347633,
-39.));
#33340=CARTESIAN_POINT('Ctrl Pts',(-2.68326084165469,-2.14187738170485,
-39.));
#33341=CARTESIAN_POINT('Ctrl Pts',(-2.62234937512617,-2.23152278993156,
-39.));
#33342=CARTESIAN_POINT('Ctrl Pts',(-2.55729461435447,-2.31811500318715,
-39.));
#33343=CARTESIAN_POINT('Ctrl Pts',(-2.49061650072561,-2.40686800706172,
-39.));
#33344=CARTESIAN_POINT('Ctrl Pts',(-2.41958537665938,-2.49241416222915,
-39.));
#33345=CARTESIAN_POINT('Ctrl Pts',(-2.34455344889113,-2.57457547121683,
-39.));
#33346=CARTESIAN_POINT('Ctrl Pts',(-2.27491905341145,-2.6508263853723,-39.));
#33347=CARTESIAN_POINT('Ctrl Pts',(-2.20183785832801,-2.72416209662977,
-39.));
#33348=CARTESIAN_POINT('Ctrl Pts',(-2.1255575635722,-2.79441872971172,-39.));
#33349=CARTESIAN_POINT('Ctrl Pts',(-2.1130737496862,-2.80591672843419,-39.));
#33350=CARTESIAN_POINT('Ctrl Pts',(-2.10050290352848,-2.81733335528404,
-39.));
#33351=CARTESIAN_POINT('Ctrl Pts',(-2.08785007700729,-2.82866421622847,
-39.));
#33352=CARTESIAN_POINT('Ctrl Pts',(-2.00281517469671,-2.90481468362719,
-39.));
#33353=CARTESIAN_POINT('Ctrl Pts',(-1.91436539047486,-2.97684040078833,
-39.));
#33354=CARTESIAN_POINT('Ctrl Pts',(-1.82290776635402,-3.04458314589731,
-39.));
#33355=CARTESIAN_POINT('Ctrl Pts',(-1.73027595536054,-3.11319561228746,
-39.));
#33356=CARTESIAN_POINT('Ctrl Pts',(-1.63455802419001,-3.17741505746554,
-39.));
#33357=CARTESIAN_POINT('Ctrl Pts',(-1.53612883601075,-3.23705171222188,
-39.));
#33358=CARTESIAN_POINT('Ctrl Pts',(-1.43752959901041,-3.29679139681137,
-39.));
#33359=CARTESIAN_POINT('Ctrl Pts',(-1.33620906279526,-3.35193305880578,
-39.));
#33360=CARTESIAN_POINT('Ctrl Pts',(-1.23250544109713,-3.40225130016081,
-39.));
#33361=CARTESIAN_POINT('Ctrl Pts',(-1.14584321588747,-3.44430085149816,
-39.));
#33362=CARTESIAN_POINT('Ctrl Pts',(-1.0575158871866,-3.48298155408148,-39.));
#33363=CARTESIAN_POINT('Ctrl Pts',(-0.967705373285046,-3.51813857622562,
-39.));
#33364=CARTESIAN_POINT('Ctrl Pts',(-0.949769817206312,-3.52515958874225,
-39.));
#33365=CARTESIAN_POINT('Ctrl Pts',(-0.931775072721506,-3.53203999475971,
-39.));
#33366=CARTESIAN_POINT('Ctrl Pts',(-0.913722538202823,-3.53877844450556,
-39.));
#33367=CARTESIAN_POINT('Ctrl Pts',(-0.899250411794731,-3.54418043924572,
-39.));
#33368=CARTESIAN_POINT('Ctrl Pts',(-0.884744979028471,-3.54948973453049,
-39.));
#33369=CARTESIAN_POINT('Ctrl Pts',(-0.870214583172694,-3.55470315445478,
-39.));
#33370=CARTESIAN_POINT('Ctrl Pts',(-0.7586042886915,-3.59474826669951,-39.));
#33371=CARTESIAN_POINT('Ctrl Pts',(-0.645392298328396,-3.62918911380257,
-39.));
#33372=CARTESIAN_POINT('Ctrl Pts',(-0.530964467386553,-3.65783073729646,
-39.));
#33373=CARTESIAN_POINT('Ctrl Pts',(-0.416951129848167,-3.68636861186927,
-39.));
#33374=CARTESIAN_POINT('Ctrl Pts',(-0.301730002251125,-3.70914977822842,
-39.));
#33375=CARTESIAN_POINT('Ctrl Pts',(-0.185651311893365,-3.72594088561003,
-39.));
#33376=CARTESIAN_POINT('Ctrl Pts',(-0.16747868702798,-3.72856960664901,
-39.));
#33377=CARTESIAN_POINT('Ctrl Pts',(-0.149284994067021,-3.73105142456686,
-39.));
#33378=CARTESIAN_POINT('Ctrl Pts',(-0.131071525139037,-3.73338533923414,
-39.));
#33379=CARTESIAN_POINT('Ctrl Pts',(-0.0169379366033663,-3.74801067268194,
-39.));
#33380=CARTESIAN_POINT('Ctrl Pts',(0.0979711271621422,-3.75683236794301,
-39.));
#33381=CARTESIAN_POINT('Ctrl Pts',(0.213312418309857,-3.76005565158897,
-39.));
#33382=CARTESIAN_POINT('Ctrl Pts',(0.285877101729696,-3.762083516502,-39.));
#33383=CARTESIAN_POINT('Ctrl Pts',(0.358613183455896,-3.76189444895298,
-39.));
#33384=CARTESIAN_POINT('Ctrl Pts',(0.431436860770681,-3.75952917685634,
-39.));
#33385=CARTESIAN_POINT('Ctrl Pts',(0.452092660752138,-3.75885828808594,
-39.));
#33386=CARTESIAN_POINT('Ctrl Pts',(0.472755511053182,-3.7580122701961,-39.));
#33387=CARTESIAN_POINT('Ctrl Pts',(0.49342350284441,-3.75699193862249,-39.));
#33388=CARTESIAN_POINT('Ctrl Pts',(0.509773936527692,-3.75618475503649,
-39.));
#33389=CARTESIAN_POINT('Ctrl Pts',(0.526124157697629,-3.75526860350868,
-39.));
#33390=CARTESIAN_POINT('Ctrl Pts',(0.542463214077932,-3.75424476214021,
-39.));
#33391=CARTESIAN_POINT('Ctrl Pts',(0.659891007300508,-3.74688647719952,
-39.));
#33392=CARTESIAN_POINT('Ctrl Pts',(0.776890688476788,-3.73396289933532,
-39.));
#33393=CARTESIAN_POINT('Ctrl Pts',(0.893098832740734,-3.71574250047003,
-39.));
#33394=CARTESIAN_POINT('Ctrl Pts',(1.01145043029335,-3.6971860272778,-39.));
#33395=CARTESIAN_POINT('Ctrl Pts',(1.1289817363392,-3.67313548364135,-39.));
#33396=CARTESIAN_POINT('Ctrl Pts',(1.24532264134319,-3.64382098539602,-39.));
#33397=CARTESIAN_POINT('Ctrl Pts',(1.36364893407646,-3.6140062276323,-39.));
#33398=CARTESIAN_POINT('Ctrl Pts',(1.48074468032365,-3.57874624629638,-39.));
#33399=CARTESIAN_POINT('Ctrl Pts',(1.59622282744335,-3.53822926970182,-39.));
#33400=CARTESIAN_POINT('Ctrl Pts',(1.67894642587911,-3.50920464309289,-39.));
#33401=CARTESIAN_POINT('Ctrl Pts',(1.76084001244962,-3.47748115701661,-39.));
#33402=CARTESIAN_POINT('Ctrl Pts',(1.84175830671377,-3.44311185638279,-39.));
#33403=CARTESIAN_POINT('Ctrl Pts',(1.86974700891392,-3.43122391275997,-39.));
#33404=CARTESIAN_POINT('Ctrl Pts',(1.8976189921892,-3.41901931236763,-39.));
#33405=CARTESIAN_POINT('Ctrl Pts',(1.9253681103356,-3.40649989145697,-39.));
#33406=CARTESIAN_POINT('Ctrl Pts',(1.94401447908019,-3.39808730920707,-39.));
#33407=CARTESIAN_POINT('Ctrl Pts',(1.96260673881699,-3.38953185050619,-39.));
#33408=CARTESIAN_POINT('Ctrl Pts',(1.98112608404139,-3.38084219828656,-39.));
#33409=CARTESIAN_POINT('Ctrl Pts',(2.09453669000687,-3.3276276428087,-39.));
#33410=CARTESIAN_POINT('Ctrl Pts',(2.20535587450821,-3.26932167429468,-39.));
#33411=CARTESIAN_POINT('Ctrl Pts',(2.31318172936241,-3.20614314300893,-39.));
#33412=CARTESIAN_POINT('Ctrl Pts',(2.42120078697442,-3.14285140820167,-39.));
#33413=CARTESIAN_POINT('Ctrl Pts',(2.52621667759038,-3.07466938567556,-39.));
#33414=CARTESIAN_POINT('Ctrl Pts',(2.6278134383443,-3.00176671616721,-39.));
#33415=CARTESIAN_POINT('Ctrl Pts',(2.65464889975007,-2.98251042532239,-39.));
#33416=CARTESIAN_POINT('Ctrl Pts',(2.68124570868624,-2.96292452198041,-39.));
#33417=CARTESIAN_POINT('Ctrl Pts',(2.70759593777791,-2.94301158064002,-39.));
#33418=CARTESIAN_POINT('Ctrl Pts',(2.72554097494419,-2.92945046619201,-39.));
#33419=CARTESIAN_POINT('Ctrl Pts',(2.74337347257275,-2.91573623922872,-39.));
#33420=CARTESIAN_POINT('Ctrl Pts',(2.76108499265317,-2.90187428087526,-39.));
#33421=CARTESIAN_POINT('Ctrl Pts',(2.86413983193027,-2.82121819468424,-39.));
#33422=CARTESIAN_POINT('Ctrl Pts',(2.96293657097843,-2.73569517853608,-39.));
#33423=CARTESIAN_POINT('Ctrl Pts',(3.05701974862933,-2.64552146010616,-39.));
#33424=CARTESIAN_POINT('Ctrl Pts',(3.15110292628022,-2.55534774167624,-39.));
#33425=CARTESIAN_POINT('Ctrl Pts',(3.24047361764325,-2.46052298890747,-39.));
#33426=CARTESIAN_POINT('Ctrl Pts',(3.3246484150941,-2.36121076386274,-39.));
#33427=CARTESIAN_POINT('Ctrl Pts',(3.36089955029359,-2.31844046911791,-39.));
#33428=CARTESIAN_POINT('Ctrl Pts',(3.39618654382643,-2.27483723891631,-39.));
#33429=CARTESIAN_POINT('Ctrl Pts',(3.43050777773768,-2.23043901384844,-39.));
#33430=CARTESIAN_POINT('Ctrl Pts',(-1.05790442297294,-3.94563850749841,
-28.));
#33431=CARTESIAN_POINT('Ctrl Pts',(-1.17552092509457,-3.90322260833457,
-28.));
#33432=CARTESIAN_POINT('Ctrl Pts',(-1.29069214983657,-3.85509352261539,
-28.));
#33433=CARTESIAN_POINT('Ctrl Pts',(-1.40318092946675,-3.80162495038346,
-28.));
#33434=CARTESIAN_POINT('Ctrl Pts',(-1.51645569700177,-3.74778277954729,
-28.));
#33435=CARTESIAN_POINT('Ctrl Pts',(-1.62701098511845,-3.68852555691594,
-28.));
#33436=CARTESIAN_POINT('Ctrl Pts',(-1.73457653866827,-3.62418713824119,
-28.));
#33437=CARTESIAN_POINT('Ctrl Pts',(-1.84251278075503,-3.55962699882501,
-28.));
#33438=CARTESIAN_POINT('Ctrl Pts',(-1.94743922183795,-3.4899498717791,-28.));
#33439=CARTESIAN_POINT('Ctrl Pts',(-2.04904592292942,-3.41545575870663,
-28.));
#33440=CARTESIAN_POINT('Ctrl Pts',(-2.11167361902161,-3.36953954822009,
-28.));
#33441=CARTESIAN_POINT('Ctrl Pts',(-2.17303933245443,-3.32179259632812,
-28.));
#33442=CARTESIAN_POINT('Ctrl Pts',(-2.2330620984525,-3.27227990388831,-28.));
#33443=CARTESIAN_POINT('Ctrl Pts',(-2.26769437499633,-3.24371178929892,
-28.));
#33444=CARTESIAN_POINT('Ctrl Pts',(-2.30187944275612,-3.21455577193222,
-28.));
#33445=CARTESIAN_POINT('Ctrl Pts',(-2.33560066189846,-3.18482388432906,
-28.));
#33446=CARTESIAN_POINT('Ctrl Pts',(-2.35176548728777,-3.17057141114382,
-28.));
#33447=CARTESIAN_POINT('Ctrl Pts',(-2.36782485329837,-3.15618556031416,
-28.));
#33448=CARTESIAN_POINT('Ctrl Pts',(-2.38377304232987,-3.14167111942472,
-28.));
#33449=CARTESIAN_POINT('Ctrl Pts',(-2.39929945678807,-3.12754053541714,
-28.));
#33450=CARTESIAN_POINT('Ctrl Pts',(-2.4147144303058,-3.11329357780667,-28.));
#33451=CARTESIAN_POINT('Ctrl Pts',(-2.43001123186977,-3.09893695799548,
-28.));
#33452=CARTESIAN_POINT('Ctrl Pts',(-2.51988581706192,-3.01458630175559,
-28.));
#33453=CARTESIAN_POINT('Ctrl Pts',(-2.60575268760725,-2.9263905122201,-28.));
#33454=CARTESIAN_POINT('Ctrl Pts',(-2.68735143209645,-2.83466145344241,
-28.));
#33455=CARTESIAN_POINT('Ctrl Pts',(-2.76850886109889,-2.74342849855061,
-28.));
#33456=CARTESIAN_POINT('Ctrl Pts',(-2.84544466814443,-2.64869965528777,
-28.));
#33457=CARTESIAN_POINT('Ctrl Pts',(-2.91785977185231,-2.55075381811677,
-28.));
#33458=CARTESIAN_POINT('Ctrl Pts',(-2.98860807815616,-2.45506242592718,
-28.));
#33459=CARTESIAN_POINT('Ctrl Pts',(-3.05504166648732,-2.35629973630334,
-28.));
#33460=CARTESIAN_POINT('Ctrl Pts',(-3.1168354308863,-2.25470965775042,-28.));
#33461=CARTESIAN_POINT('Ctrl Pts',(-3.16443730013298,-2.17645131432253,
-28.));
#33462=CARTESIAN_POINT('Ctrl Pts',(-3.20928496516993,-2.0965147583857,-28.));
#33463=CARTESIAN_POINT('Ctrl Pts',(-3.25120884148141,-2.01500844711875,
-28.));
#33464=CARTESIAN_POINT('Ctrl Pts',(-3.26049991453858,-1.9969452058532,-28.));
#33465=CARTESIAN_POINT('Ctrl Pts',(-3.26964731182438,-1.97880486295949,
-28.));
#33466=CARTESIAN_POINT('Ctrl Pts',(-3.27864905600516,-1.96058859515145,
-28.));
#33467=CARTESIAN_POINT('Ctrl Pts',(-3.28607688065843,-1.94555737004687,
-28.));
#33468=CARTESIAN_POINT('Ctrl Pts',(-3.29340549865561,-1.93047437020423,
-28.));
#33469=CARTESIAN_POINT('Ctrl Pts',(-3.30062766338968,-1.91535349873123,
-28.));
#33470=CARTESIAN_POINT('Ctrl Pts',(-3.35136195689617,-1.80913233656823,
-28.));
#33471=CARTESIAN_POINT('Ctrl Pts',(-3.39692754659769,-1.7008825211242,-28.));
#33472=CARTESIAN_POINT('Ctrl Pts',(-3.43705405523292,-1.59086014700212,
-28.));
#33473=CARTESIAN_POINT('Ctrl Pts',(-3.47636174188234,-1.48308289068189,
-28.));
#33474=CARTESIAN_POINT('Ctrl Pts',(-3.51045028631878,-1.37360404476521,
-28.));
#33475=CARTESIAN_POINT('Ctrl Pts',(-3.53901673706831,-1.26265350321925,
-28.));
#33476=CARTESIAN_POINT('Ctrl Pts',(-3.54583445116938,-1.23617387233156,
-28.));
#33477=CARTESIAN_POINT('Ctrl Pts',(-3.55233739955794,-1.20961038884467,
-28.));
#33478=CARTESIAN_POINT('Ctrl Pts',(-3.55852102006359,-1.18296614385692,
-28.));
#33479=CARTESIAN_POINT('Ctrl Pts',(-3.58533465285514,-1.06743043133119,
-28.));
#33480=CARTESIAN_POINT('Ctrl Pts',(-3.60614802893092,-0.950375395504629,
-28.));
#33481=CARTESIAN_POINT('Ctrl Pts',(-3.62104714913887,-0.832239843135369,
-28.));
#33482=CARTESIAN_POINT('Ctrl Pts',(-3.63268207221584,-0.739986203639362,
-28.));
#33483=CARTESIAN_POINT('Ctrl Pts',(-3.64070921633916,-0.647073564177628,
-28.));
#33484=CARTESIAN_POINT('Ctrl Pts',(-3.64514860307971,-0.553717990972986,
-28.));
#33485=CARTESIAN_POINT('Ctrl Pts',(-3.64592450960589,-0.537401503417666,
-28.));
#33486=CARTESIAN_POINT('Ctrl Pts',(-3.64659030245521,-0.521081374381654,
-28.));
#33487=CARTESIAN_POINT('Ctrl Pts',(-3.64714640790116,-0.504759992890122,
-28.));
#33488=CARTESIAN_POINT('Ctrl Pts',(-3.65110332464657,-0.3886267160034,-28.));
#33489=CARTESIAN_POINT('Ctrl Pts',(-3.64951230537173,-0.272408796396214,
-28.));
#33490=CARTESIAN_POINT('Ctrl Pts',(-3.64251723929508,-0.156512198468872,
-28.));
#33491=CARTESIAN_POINT('Ctrl Pts',(-3.63549581042975,-0.0401788130280003,
-28.));
#33492=CARTESIAN_POINT('Ctrl Pts',(-3.62302921007484,0.0758317450340023,
-28.));
#33493=CARTESIAN_POINT('Ctrl Pts',(-3.60521119974026,0.19109879958983,-28.));
#33494=CARTESIAN_POINT('Ctrl Pts',(-3.58767840055076,0.304520785700679,
-28.));
#33495=CARTESIAN_POINT('Ctrl Pts',(-3.56496370537445,0.417223667382557,
-28.));
#33496=CARTESIAN_POINT('Ctrl Pts',(-3.53711222719414,0.528784290151367,
-28.));
#33497=CARTESIAN_POINT('Ctrl Pts',(-3.51189251588176,0.629803226447788,
-28.));
#33498=CARTESIAN_POINT('Ctrl Pts',(-3.48246023862158,0.729885733889866,
-28.));
#33499=CARTESIAN_POINT('Ctrl Pts',(-3.44882098814669,0.828693432313728,
-28.));
#33500=CARTESIAN_POINT('Ctrl Pts',(-3.4427386179877,0.846559020514666,-28.));
#33501=CARTESIAN_POINT('Ctrl Pts',(-3.43652137213233,0.864374779285486,
-28.));
#33502=CARTESIAN_POINT('Ctrl Pts',(-3.43017104275558,0.882134801923077,
-28.));
#33503=CARTESIAN_POINT('Ctrl Pts',(-3.3919499839386,0.989027976993363,-28.));
#33504=CARTESIAN_POINT('Ctrl Pts',(-3.34889518138372,1.09395211482332,-28.));
#33505=CARTESIAN_POINT('Ctrl Pts',(-3.30106890262405,1.19649560051157,-28.));
#33506=CARTESIAN_POINT('Ctrl Pts',(-3.26179920216696,1.28069307669486,-28.));
#33507=CARTESIAN_POINT('Ctrl Pts',(-3.21931172738894,1.36328529314877,-28.));
#33508=CARTESIAN_POINT('Ctrl Pts',(-3.17362084982711,1.44402623804176,-28.));
#33509=CARTESIAN_POINT('Ctrl Pts',(-3.15207647343335,1.48209758619672,-28.));
#33510=CARTESIAN_POINT('Ctrl Pts',(-3.12981961866877,1.51975706275399,-28.));
#33511=CARTESIAN_POINT('Ctrl Pts',(-3.1068505199988,1.55697730019376,-28.));
#33512=CARTESIAN_POINT('Ctrl Pts',(-3.09148427832198,1.58187750076261,-28.));
#33513=CARTESIAN_POINT('Ctrl Pts',(-3.07579848046801,1.60658184767048,-28.));
#33514=CARTESIAN_POINT('Ctrl Pts',(-3.05981013081646,1.63105693002514,-28.));
#33515=CARTESIAN_POINT('Ctrl Pts',(-3.0009759331342,1.72112074930146,-28.));
#33516=CARTESIAN_POINT('Ctrl Pts',(-2.93799599951988,1.80816816462597,-28.));
#33517=CARTESIAN_POINT('Ctrl Pts',(-2.870903420132,1.8918173136697,-28.));
#33518=CARTESIAN_POINT('Ctrl Pts',(-2.81008529796309,1.96764364516987,-28.));
#33519=CARTESIAN_POINT('Ctrl Pts',(-2.74588720662993,2.04067754747659,-28.));
#33520=CARTESIAN_POINT('Ctrl Pts',(-2.67831174925371,2.11060476373359,-28.));
#33521=CARTESIAN_POINT('Ctrl Pts',(-2.64566301465728,2.14438973853489,-28.));
#33522=CARTESIAN_POINT('Ctrl Pts',(-2.6122255718507,2.17744902968664,-28.));
#33523=CARTESIAN_POINT('Ctrl Pts',(-2.57802990330401,2.20976968150249,-28.));
#33524=CARTESIAN_POINT('Origin',(0.,0.,-28.));
#33525=CARTESIAN_POINT('',(1.38777878078145E-16,-5.,-28.));
#33526=CARTESIAN_POINT('',(1.38777878078145E-16,5.,-28.));
#33527=CARTESIAN_POINT('Origin',(0.,0.,-28.));
#33528=CARTESIAN_POINT('Origin',(0.,0.,-28.));
#33529=CARTESIAN_POINT('Origin',(0.,0.,0.));
#33530=CARTESIAN_POINT('',(-5.,-6.12323399573677E-16,-39.));
#33531=CARTESIAN_POINT('Origin',(0.,0.,-39.));
#33532=CARTESIAN_POINT('',(-5.,3.06161699786838E-16,-31.3571312154738));
#33533=CARTESIAN_POINT('',(-5.,6.12323399573677E-16,0.));
#33534=CARTESIAN_POINT('',(-2.7252308025327,4.19203018511639,-30.8799792272101));
#33535=CARTESIAN_POINT('Ctrl Pts',(-2.7252308025327,4.19203018511639,-30.8799792272101));
#33536=CARTESIAN_POINT('Ctrl Pts',(-2.8912176764087,4.08412243600022,-30.8653304951571));
#33537=CARTESIAN_POINT('Ctrl Pts',(-3.04862894705818,3.96746986254389,-30.8620029267808));
#33538=CARTESIAN_POINT('Ctrl Pts',(-3.74387664835538,3.39066664475822,-30.8821120697405));
#33539=CARTESIAN_POINT('Ctrl Pts',(-4.21066500973337,2.79554609173792,-31.0137757194408));
#33540=CARTESIAN_POINT('Ctrl Pts',(-4.83880724780192,1.45969207554558,-31.2576781989471));
#33541=CARTESIAN_POINT('Ctrl Pts',(-5.,0.716580051177333,-31.3571312154738));
#33542=CARTESIAN_POINT('Ctrl Pts',(-5.,6.93889390390723E-17,-31.3571312154738));
#33543=CARTESIAN_POINT('',(2.72523080253269,4.1920301851164,-30.8799792272101));
#33544=CARTESIAN_POINT('Ctrl Pts',(2.72523080253269,4.1920301851164,-30.8799792272101));
#33545=CARTESIAN_POINT('Ctrl Pts',(2.47095718963917,4.35733297434463,-30.9024194716491));
#33546=CARTESIAN_POINT('Ctrl Pts',(2.1983745065567,4.50125462875715,-30.923256490722));
#33547=CARTESIAN_POINT('Ctrl Pts',(1.29915176153723,4.87407242020745,-30.9789098121903));
#33548=CARTESIAN_POINT('Ctrl Pts',(0.62898575038369,5.,-31.));
#33549=CARTESIAN_POINT('Ctrl Pts',(-0.62898575038369,5.,-31.));
#33550=CARTESIAN_POINT('Ctrl Pts',(-1.29915176153723,4.87407242020745,-30.9789098121903));
#33551=CARTESIAN_POINT('Ctrl Pts',(-2.1983745065567,4.50125462875714,-30.923256490722));
#33552=CARTESIAN_POINT('Ctrl Pts',(-2.47095718963918,4.35733297434463,-30.9024194716491));
#33553=CARTESIAN_POINT('Ctrl Pts',(-2.7252308025327,4.19203018511639,-30.8799792272101));
#33554=CARTESIAN_POINT('',(2.72523080253269,-4.1920301851164,-30.8799792272101));
#33555=CARTESIAN_POINT('Ctrl Pts',(2.72523080253269,-4.1920301851164,-30.8799792272101));
#33556=CARTESIAN_POINT('Ctrl Pts',(2.89121767640869,-4.08412243600022,-30.8653304951571));
#33557=CARTESIAN_POINT('Ctrl Pts',(3.04862894705818,-3.9674698625439,-30.8620029267808));
#33558=CARTESIAN_POINT('Ctrl Pts',(3.74387664835538,-3.39066664475823,-30.8821120697405));
#33559=CARTESIAN_POINT('Ctrl Pts',(4.21066500973337,-2.79554609173792,-31.0137757194408));
#33560=CARTESIAN_POINT('Ctrl Pts',(4.83880724780192,-1.45969207554558,-31.2576781989471));
#33561=CARTESIAN_POINT('Ctrl Pts',(5.,-0.716580051177333,-31.3571312154738));
#33562=CARTESIAN_POINT('Ctrl Pts',(5.,0.716580051177333,-31.3571312154738));
#33563=CARTESIAN_POINT('Ctrl Pts',(4.83880724780192,1.45969207554558,-31.2576781989471));
#33564=CARTESIAN_POINT('Ctrl Pts',(4.21066500973337,2.79554609173792,-31.0137757194408));
#33565=CARTESIAN_POINT('Ctrl Pts',(3.74387664835538,3.39066664475823,-30.8821120697405));
#33566=CARTESIAN_POINT('Ctrl Pts',(3.04862894705818,3.9674698625439,-30.8620029267808));
#33567=CARTESIAN_POINT('Ctrl Pts',(2.89121767640869,4.08412243600022,-30.8653304951571));
#33568=CARTESIAN_POINT('Ctrl Pts',(2.72523080253269,4.1920301851164,-30.8799792272101));
#33569=CARTESIAN_POINT('',(-2.7252308025327,-4.19203018511639,-30.8799792272101));
#33570=CARTESIAN_POINT('Ctrl Pts',(-2.7252308025327,-4.19203018511639,-30.8799792272101));
#33571=CARTESIAN_POINT('Ctrl Pts',(-2.47095718963918,-4.35733297434463,
-30.9024194716491));
#33572=CARTESIAN_POINT('Ctrl Pts',(-2.1983745065567,-4.50125462875714,-30.923256490722));
#33573=CARTESIAN_POINT('Ctrl Pts',(-1.29915176153723,-4.87407242020745,
-30.9789098121903));
#33574=CARTESIAN_POINT('Ctrl Pts',(-0.628985750383691,-5.,-31.));
#33575=CARTESIAN_POINT('Ctrl Pts',(0.628985750383688,-5.,-31.));
#33576=CARTESIAN_POINT('Ctrl Pts',(1.29915176153722,-4.87407242020745,-30.9789098121903));
#33577=CARTESIAN_POINT('Ctrl Pts',(2.1983745065567,-4.50125462875715,-30.923256490722));
#33578=CARTESIAN_POINT('Ctrl Pts',(2.47095718963917,-4.35733297434463,-30.9024194716491));
#33579=CARTESIAN_POINT('Ctrl Pts',(2.72523080253269,-4.1920301851164,-30.8799792272101));
#33580=CARTESIAN_POINT('Ctrl Pts',(-5.,6.93889390390723E-17,-31.3571312154738));
#33581=CARTESIAN_POINT('Ctrl Pts',(-5.,-0.716580051177333,-31.3571312154738));
#33582=CARTESIAN_POINT('Ctrl Pts',(-4.83880724780192,-1.45969207554558,
-31.2576781989471));
#33583=CARTESIAN_POINT('Ctrl Pts',(-4.21066500973337,-2.79554609173792,
-31.0137757194408));
#33584=CARTESIAN_POINT('Ctrl Pts',(-3.74387664835538,-3.39066664475822,
-30.8821120697405));
#33585=CARTESIAN_POINT('Ctrl Pts',(-3.04862894705818,-3.96746986254389,
-30.8620029267808));
#33586=CARTESIAN_POINT('Ctrl Pts',(-2.8912176764087,-4.08412243600022,-30.8653304951571));
#33587=CARTESIAN_POINT('Ctrl Pts',(-2.7252308025327,-4.19203018511639,-30.8799792272101));
#33588=CARTESIAN_POINT('Origin',(0.,0.,-39.));
#33589=CARTESIAN_POINT('Origin',(0.,0.,0.));
#33590=CARTESIAN_POINT('Ctrl Pts',(1.52655665885959E-15,5.,-28.));
#33591=CARTESIAN_POINT('Ctrl Pts',(0.629253024152622,5.,-28.));
#33592=CARTESIAN_POINT('Ctrl Pts',(1.29953505458189,4.87396779126795,-27.9766356618315));
#33593=CARTESIAN_POINT('Ctrl Pts',(2.53104134263485,4.3632766282051,-27.8921989820475));
#33594=CARTESIAN_POINT('Ctrl Pts',(3.09237623737018,3.97869157449529,-27.832297423241));
#33595=CARTESIAN_POINT('Ctrl Pts',(3.97870723422023,3.09236057764524,-27.7194782327905));
#33596=CARTESIAN_POINT('Ctrl Pts',(4.36328000904426,2.53103238085929,-27.6591541770631));
#33597=CARTESIAN_POINT('Ctrl Pts',(4.87396226264421,1.29954919562912,-27.5737468441049));
#33598=CARTESIAN_POINT('Ctrl Pts',(5.,0.629275259871354,-27.5499546279118));
#33599=CARTESIAN_POINT('Ctrl Pts',(5.,-0.629275259871354,-27.5499546279118));
#33600=CARTESIAN_POINT('Ctrl Pts',(4.87396226264421,-1.29954919562912,-27.5737468441049));
#33601=CARTESIAN_POINT('Ctrl Pts',(4.36328000904425,-2.53103238085929,-27.6591541770631));
#33602=CARTESIAN_POINT('Ctrl Pts',(3.97870723422023,-3.09236057764524,-27.7194782327905));
#33603=CARTESIAN_POINT('Ctrl Pts',(3.09237623737018,-3.9786915744953,-27.832297423241));
#33604=CARTESIAN_POINT('Ctrl Pts',(2.53104134263485,-4.3632766282051,-27.8921989820475));
#33605=CARTESIAN_POINT('Ctrl Pts',(1.29953505458189,-4.87396779126795,-27.9766356618315));
#33606=CARTESIAN_POINT('Ctrl Pts',(0.629253024152619,-5.,-28.));
#33607=CARTESIAN_POINT('Ctrl Pts',(-8.32667268468867E-16,-5.,-28.));
#33608=CARTESIAN_POINT('Origin',(0.,0.,0.));
#33609=CARTESIAN_POINT('Ctrl Pts',(1.87350135405495E-15,5.,-28.));
#33610=CARTESIAN_POINT('Ctrl Pts',(-0.629253024152618,5.,-28.));
#33611=CARTESIAN_POINT('Ctrl Pts',(-1.29953505458189,4.87396779126795,-27.9766356618315));
#33612=CARTESIAN_POINT('Ctrl Pts',(-2.53104134263485,4.3632766282051,-27.8921989820475));
#33613=CARTESIAN_POINT('Ctrl Pts',(-3.09237623737018,3.9786915744953,-27.832297423241));
#33614=CARTESIAN_POINT('Ctrl Pts',(-3.97870723422023,3.09236057764524,-27.7194782327905));
#33615=CARTESIAN_POINT('Ctrl Pts',(-4.36328000904426,2.53103238085929,-27.6591541770631));
#33616=CARTESIAN_POINT('Ctrl Pts',(-4.87396226264421,1.29954919562912,-27.5737468441049));
#33617=CARTESIAN_POINT('Ctrl Pts',(-5.,0.629275259871354,-27.5499546279118));
#33618=CARTESIAN_POINT('Ctrl Pts',(-5.,0.,-27.5499546279118));
#33619=CARTESIAN_POINT('Ctrl Pts',(-5.,-0.629275259871354,-27.5499546279118));
#33620=CARTESIAN_POINT('Ctrl Pts',(-4.87396226264421,-1.29954919562912,
-27.5737468441049));
#33621=CARTESIAN_POINT('Ctrl Pts',(-4.36328000904425,-2.53103238085929,
-27.6591541770631));
#33622=CARTESIAN_POINT('Ctrl Pts',(-3.97870723422023,-3.09236057764524,
-27.7194782327905));
#33623=CARTESIAN_POINT('Ctrl Pts',(-3.09237623737018,-3.9786915744953,-27.832297423241));
#33624=CARTESIAN_POINT('Ctrl Pts',(-2.53104134263485,-4.3632766282051,-27.8921989820475));
#33625=CARTESIAN_POINT('Ctrl Pts',(-1.29953505458189,-4.87396779126795,
-27.9766356618315));
#33626=CARTESIAN_POINT('Ctrl Pts',(-0.629253024152621,-5.,-28.));
#33627=CARTESIAN_POINT('Ctrl Pts',(-1.45716771982052E-15,-5.,-28.));
#33628=CARTESIAN_POINT('Origin',(0.,0.,0.));
#33629=CARTESIAN_POINT('',(-5.,4.16333634234434E-16,27.5499546279118));
#33630=CARTESIAN_POINT('Ctrl Pts',(-5.,-1.38777878078145E-16,27.5499546279118));
#33631=CARTESIAN_POINT('Ctrl Pts',(-5.,-0.629275259871354,27.5499546279118));
#33632=CARTESIAN_POINT('Ctrl Pts',(-4.87396226264421,-1.29954919562912,
27.5737468441049));
#33633=CARTESIAN_POINT('Ctrl Pts',(-4.36328000904425,-2.53103238085929,
27.6591541770631));
#33634=CARTESIAN_POINT('Ctrl Pts',(-3.97870723422023,-3.09236057764524,
27.7194782327905));
#33635=CARTESIAN_POINT('Ctrl Pts',(-3.09237623737018,-3.9786915744953,27.832297423241));
#33636=CARTESIAN_POINT('Ctrl Pts',(-2.53104134263485,-4.3632766282051,27.8921989820475));
#33637=CARTESIAN_POINT('Ctrl Pts',(-1.29953505458189,-4.87396779126795,
27.9766356618315));
#33638=CARTESIAN_POINT('Ctrl Pts',(-0.629253024152621,-5.,28.));
#33639=CARTESIAN_POINT('Ctrl Pts',(0.629253024152619,-5.,28.));
#33640=CARTESIAN_POINT('Ctrl Pts',(1.29953505458189,-4.87396779126795,27.9766356618315));
#33641=CARTESIAN_POINT('Ctrl Pts',(2.53104134263485,-4.3632766282051,27.8921989820475));
#33642=CARTESIAN_POINT('Ctrl Pts',(3.09237623737018,-3.9786915744953,27.832297423241));
#33643=CARTESIAN_POINT('Ctrl Pts',(3.97870723422023,-3.09236057764524,27.7194782327905));
#33644=CARTESIAN_POINT('Ctrl Pts',(4.36328000904425,-2.53103238085929,27.6591541770631));
#33645=CARTESIAN_POINT('Ctrl Pts',(4.87396226264421,-1.29954919562912,27.5737468441049));
#33646=CARTESIAN_POINT('Ctrl Pts',(5.,-0.629275259871354,27.5499546279118));
#33647=CARTESIAN_POINT('Ctrl Pts',(5.,0.629275259871354,27.5499546279118));
#33648=CARTESIAN_POINT('Ctrl Pts',(4.87396226264421,1.29954919562912,27.5737468441049));
#33649=CARTESIAN_POINT('Ctrl Pts',(4.36328000904426,2.53103238085929,27.6591541770631));
#33650=CARTESIAN_POINT('Ctrl Pts',(3.97870723422023,3.09236057764524,27.7194782327905));
#33651=CARTESIAN_POINT('Ctrl Pts',(3.09237623737018,3.9786915744953,27.832297423241));
#33652=CARTESIAN_POINT('Ctrl Pts',(2.53104134263485,4.3632766282051,27.8921989820475));
#33653=CARTESIAN_POINT('Ctrl Pts',(1.29953505458189,4.87396779126795,27.9766356618315));
#33654=CARTESIAN_POINT('Ctrl Pts',(0.629253024152622,5.,28.));
#33655=CARTESIAN_POINT('Ctrl Pts',(-0.629253024152618,5.,28.));
#33656=CARTESIAN_POINT('Ctrl Pts',(-1.29953505458188,4.87396779126795,27.9766356618315));
#33657=CARTESIAN_POINT('Ctrl Pts',(-2.53104134263485,4.3632766282051,27.8921989820475));
#33658=CARTESIAN_POINT('Ctrl Pts',(-3.09237623737017,3.9786915744953,27.832297423241));
#33659=CARTESIAN_POINT('Ctrl Pts',(-3.97870723422023,3.09236057764525,27.7194782327905));
#33660=CARTESIAN_POINT('Ctrl Pts',(-4.36328000904425,2.5310323808593,27.6591541770631));
#33661=CARTESIAN_POINT('Ctrl Pts',(-4.87396226264421,1.29954919562912,27.5737468441049));
#33662=CARTESIAN_POINT('Ctrl Pts',(-5.,0.629275259871355,27.5499546279118));
#33663=CARTESIAN_POINT('Ctrl Pts',(-5.,-1.38777878078145E-16,27.5499546279118));
#33664=CARTESIAN_POINT('',(-5.,-6.12323399573677E-16,31.3571312154738));
#33665=CARTESIAN_POINT('',(-5.,-6.12323399573677E-16,0.));
#33666=CARTESIAN_POINT('',(-2.7252308025327,-4.19203018511639,30.8799792272101));
#33667=CARTESIAN_POINT('Ctrl Pts',(-2.7252308025327,-4.19203018511639,30.8799792272101));
#33668=CARTESIAN_POINT('Ctrl Pts',(-2.8912176764087,-4.08412243600022,30.8653304951571));
#33669=CARTESIAN_POINT('Ctrl Pts',(-3.04862894705818,-3.96746986254389,
30.8620029267808));
#33670=CARTESIAN_POINT('Ctrl Pts',(-3.74387664835538,-3.39066664475822,
30.8821120697405));
#33671=CARTESIAN_POINT('Ctrl Pts',(-4.21066500973337,-2.79554609173792,
31.0137757194408));
#33672=CARTESIAN_POINT('Ctrl Pts',(-4.83880724780192,-1.45969207554558,
31.2576781989471));
#33673=CARTESIAN_POINT('Ctrl Pts',(-5.,-0.716580051177333,31.3571312154738));
#33674=CARTESIAN_POINT('Ctrl Pts',(-5.,-3.46944695195361E-16,31.3571312154738));
#33675=CARTESIAN_POINT('',(2.7252308025327,-4.1920301851164,30.8799792272101));
#33676=CARTESIAN_POINT('Ctrl Pts',(2.7252308025327,-4.19203018511639,30.8799792272101));
#33677=CARTESIAN_POINT('Ctrl Pts',(2.47095718963918,-4.35733297434463,30.9024194716491));
#33678=CARTESIAN_POINT('Ctrl Pts',(2.1983745065567,-4.50125462875714,30.923256490722));
#33679=CARTESIAN_POINT('Ctrl Pts',(1.29915176153723,-4.87407242020745,30.9789098121903));
#33680=CARTESIAN_POINT('Ctrl Pts',(0.62898575038369,-5.,31.));
#33681=CARTESIAN_POINT('Ctrl Pts',(-0.62898575038369,-5.,31.));
#33682=CARTESIAN_POINT('Ctrl Pts',(-1.29915176153723,-4.87407242020745,
30.9789098121903));
#33683=CARTESIAN_POINT('Ctrl Pts',(-2.1983745065567,-4.50125462875714,30.923256490722));
#33684=CARTESIAN_POINT('Ctrl Pts',(-2.47095718963918,-4.35733297434463,
30.9024194716491));
#33685=CARTESIAN_POINT('Ctrl Pts',(-2.7252308025327,-4.19203018511639,30.8799792272101));
#33686=CARTESIAN_POINT('',(2.7252308025327,4.1920301851164,30.8799792272101));
#33687=CARTESIAN_POINT('Ctrl Pts',(2.7252308025327,4.19203018511639,30.8799792272101));
#33688=CARTESIAN_POINT('Ctrl Pts',(2.89121767640869,4.08412243600022,30.8653304951571));
#33689=CARTESIAN_POINT('Ctrl Pts',(3.04862894705818,3.9674698625439,30.8620029267808));
#33690=CARTESIAN_POINT('Ctrl Pts',(3.74387664835538,3.39066664475823,30.8821120697405));
#33691=CARTESIAN_POINT('Ctrl Pts',(4.21066500973337,2.79554609173792,31.0137757194408));
#33692=CARTESIAN_POINT('Ctrl Pts',(4.83880724780192,1.45969207554558,31.2576781989471));
#33693=CARTESIAN_POINT('Ctrl Pts',(5.,0.716580051177333,31.3571312154738));
#33694=CARTESIAN_POINT('Ctrl Pts',(5.,-0.716580051177333,31.3571312154738));
#33695=CARTESIAN_POINT('Ctrl Pts',(4.83880724780192,-1.45969207554558,31.2576781989471));
#33696=CARTESIAN_POINT('Ctrl Pts',(4.21066500973337,-2.79554609173792,31.0137757194408));
#33697=CARTESIAN_POINT('Ctrl Pts',(3.74387664835538,-3.39066664475823,30.8821120697405));
#33698=CARTESIAN_POINT('Ctrl Pts',(3.04862894705818,-3.9674698625439,30.8620029267808));
#33699=CARTESIAN_POINT('Ctrl Pts',(2.89121767640869,-4.08412243600022,30.8653304951571));
#33700=CARTESIAN_POINT('Ctrl Pts',(2.7252308025327,-4.19203018511639,30.8799792272101));
#33701=CARTESIAN_POINT('',(-2.7252308025327,4.19203018511639,30.8799792272101));
#33702=CARTESIAN_POINT('Ctrl Pts',(-2.7252308025327,4.19203018511639,30.8799792272101));
#33703=CARTESIAN_POINT('Ctrl Pts',(-2.47095718963918,4.35733297434463,30.9024194716491));
#33704=CARTESIAN_POINT('Ctrl Pts',(-2.1983745065567,4.50125462875714,30.923256490722));
#33705=CARTESIAN_POINT('Ctrl Pts',(-1.29915176153723,4.87407242020745,30.9789098121903));
#33706=CARTESIAN_POINT('Ctrl Pts',(-0.62898575038369,5.,31.));
#33707=CARTESIAN_POINT('Ctrl Pts',(0.62898575038369,5.,31.));
#33708=CARTESIAN_POINT('Ctrl Pts',(1.29915176153722,4.87407242020745,30.9789098121903));
#33709=CARTESIAN_POINT('Ctrl Pts',(2.1983745065567,4.50125462875714,30.923256490722));
#33710=CARTESIAN_POINT('Ctrl Pts',(2.47095718963918,4.35733297434463,30.9024194716491));
#33711=CARTESIAN_POINT('Ctrl Pts',(2.7252308025327,4.1920301851164,30.8799792272101));
#33712=CARTESIAN_POINT('Ctrl Pts',(-5.,4.85722573273506E-16,31.3571312154738));
#33713=CARTESIAN_POINT('Ctrl Pts',(-5.,0.716580051177333,31.3571312154738));
#33714=CARTESIAN_POINT('Ctrl Pts',(-4.83880724780192,1.45969207554558,31.2576781989471));
#33715=CARTESIAN_POINT('Ctrl Pts',(-4.21066500973337,2.79554609173792,31.0137757194408));
#33716=CARTESIAN_POINT('Ctrl Pts',(-3.74387664835538,3.39066664475822,30.8821120697405));
#33717=CARTESIAN_POINT('Ctrl Pts',(-3.04862894705818,3.9674698625439,30.8620029267808));
#33718=CARTESIAN_POINT('Ctrl Pts',(-2.8912176764087,4.08412243600022,30.8653304951571));
#33719=CARTESIAN_POINT('Ctrl Pts',(-2.7252308025327,4.19203018511639,30.8799792272101));
#33720=CARTESIAN_POINT('Origin',(-3.07687348673047,0.,34.8644926758824));
#33721=CARTESIAN_POINT('',(-2.7252308025327,5.5,30.8799792272101));
#33722=CARTESIAN_POINT('',(-2.7252308025327,0.,30.8799792272101));
#33723=CARTESIAN_POINT('',(-6.78850072387334,5.5,33.3732437856903));
#33724=CARTESIAN_POINT('Origin',(-3.07687348673047,5.5,34.8644926758824));
#33725=CARTESIAN_POINT('',(-6.78850072387334,-5.5,33.3732437856903));
#33726=CARTESIAN_POINT('',(-6.78850072387334,0.,33.3732437856903));
#33727=CARTESIAN_POINT('',(-2.7252308025327,-5.5,30.8799792272101));
#33728=CARTESIAN_POINT('Origin',(-3.07687348673047,-5.5,34.8644926758824));
#33729=CARTESIAN_POINT('',(-2.7252308025327,0.,30.8799792272101));
#33730=CARTESIAN_POINT('Origin',(0.,0.,0.));
#33731=CARTESIAN_POINT('',(2.7252308025327,5.5,30.8799792272101));
#33732=CARTESIAN_POINT('',(2.7252308025327,0.,30.8799792272101));
#33733=CARTESIAN_POINT('Origin',(0.,5.5,0.));
#33734=CARTESIAN_POINT('Origin',(-3.07687348673047,0.,-34.8644926758824));
#33735=CARTESIAN_POINT('',(-2.7252308025327,-5.5,-30.8799792272101));
#33736=CARTESIAN_POINT('',(-2.7252308025327,0.,-30.8799792272101));
#33737=CARTESIAN_POINT('',(-6.78850072387334,-5.5,-33.3732437856903));
#33738=CARTESIAN_POINT('Origin',(-3.07687348673047,-5.5,-34.8644926758824));
#33739=CARTESIAN_POINT('',(-6.78850072387334,5.5,-33.3732437856903));
#33740=CARTESIAN_POINT('',(-6.78850072387334,0.,-33.3732437856903));
#33741=CARTESIAN_POINT('',(-2.7252308025327,5.5,-30.8799792272101));
#33742=CARTESIAN_POINT('Origin',(-3.07687348673047,5.5,-34.8644926758824));
#33743=CARTESIAN_POINT('',(-2.7252308025327,0.,-30.8799792272101));
#33744=CARTESIAN_POINT('Origin',(0.,0.,0.));
#33745=CARTESIAN_POINT('',(2.72523080253269,-5.5,-30.8799792272101));
#33746=CARTESIAN_POINT('',(2.72523080253269,0.,-30.8799792272101));
#33747=CARTESIAN_POINT('Origin',(0.,-5.5,0.));
#33748=CARTESIAN_POINT('Origin',(-3.07687348673047,5.5,34.8644926758824));
#33749=CARTESIAN_POINT('',(-2.68127546700798,6.,30.3819150461261));
#33750=CARTESIAN_POINT('Origin',(-2.68127546700798,5.5,30.3819150461261));
#33751=CARTESIAN_POINT('',(-7.2524541285162,6.,33.1868376744163));
#33752=CARTESIAN_POINT('Origin',(-3.07687348673047,6.,34.8644926758824));
#33753=CARTESIAN_POINT('Origin',(-7.2524541285162,5.5,33.1868376744163));
#33754=CARTESIAN_POINT('Origin',(-12.8198949842305,5.5,30.9499643391281));
#33755=CARTESIAN_POINT('',(-18.3383784711987,6.,28.5948974602351));
#33756=CARTESIAN_POINT('',(-18.7982520951128,5.5,28.398641886994));
#33757=CARTESIAN_POINT('Origin',(-18.3383784711987,5.5,28.5948974602351));
#33758=CARTESIAN_POINT('Origin',(-12.8198949842305,5.5,30.9499643391281));
#33759=CARTESIAN_POINT('Origin',(-12.8198949842305,6.,30.9499643391281));
#33760=CARTESIAN_POINT('Origin',(-22.4772410864249,5.5,26.8285973010654));
#33761=CARTESIAN_POINT('',(-19.5873100895989,6.,23.3792062194998));
#33762=CARTESIAN_POINT('',(-19.9084135336906,5.5,23.7624718952293));
#33763=CARTESIAN_POINT('Origin',(-19.5873100895989,5.5,23.3792062194998));
#33764=CARTESIAN_POINT('Origin',(-22.4772410864249,5.5,26.8285973010654));
#33765=CARTESIAN_POINT('Origin',(-22.4772410864249,6.,26.8285973010654));
#33766=CARTESIAN_POINT('Origin',(0.,5.5,0.));
#33767=CARTESIAN_POINT('',(-23.3792062194998,6.,19.5873100895989));
#33768=CARTESIAN_POINT('',(-23.7624718952293,5.5,19.9084135336906));
#33769=CARTESIAN_POINT('Origin',(-23.3792062194998,5.5,19.5873100895989));
#33770=CARTESIAN_POINT('Origin',(0.,5.5,0.));
#33771=CARTESIAN_POINT('Origin',(0.,6.,0.));
#33772=CARTESIAN_POINT('Origin',(-26.8285973010653,5.5,22.4772410864249));
#33773=CARTESIAN_POINT('',(-28.5948974602351,6.,18.3383784711987));
#33774=CARTESIAN_POINT('',(-28.398641886994,5.5,18.7982520951128));
#33775=CARTESIAN_POINT('Origin',(-28.5948974602351,5.5,18.3383784711987));
#33776=CARTESIAN_POINT('Origin',(-26.8285973010653,5.5,22.4772410864249));
#33777=CARTESIAN_POINT('Origin',(-26.8285973010653,6.,22.4772410864249));
#33778=CARTESIAN_POINT('Origin',(-30.9499643391281,5.5,12.8198949842305));
#33779=CARTESIAN_POINT('',(-33.1868376744162,6.,7.2524541285162));
#33780=CARTESIAN_POINT('',(-33.3732437856903,5.5,6.78850072387334));
#33781=CARTESIAN_POINT('Origin',(-33.1868376744162,5.5,7.2524541285162));
#33782=CARTESIAN_POINT('Origin',(-30.9499643391281,5.5,12.8198949842305));
#33783=CARTESIAN_POINT('Origin',(-30.9499643391281,6.,12.8198949842305));
#33784=CARTESIAN_POINT('Origin',(-34.8644926758824,5.5,3.07687348673047));
#33785=CARTESIAN_POINT('',(-30.3819150461261,6.,2.68127546700798));
#33786=CARTESIAN_POINT('',(-30.8799792272101,5.5,2.7252308025327));
#33787=CARTESIAN_POINT('Origin',(-30.3819150461261,5.5,2.68127546700798));
#33788=CARTESIAN_POINT('Origin',(-34.8644926758824,5.5,3.07687348673047));
#33789=CARTESIAN_POINT('Origin',(-34.8644926758824,6.,3.07687348673047));
#33790=CARTESIAN_POINT('Origin',(0.,5.5,0.));
#33791=CARTESIAN_POINT('',(-30.3819150461261,6.,-2.68127546700797));
#33792=CARTESIAN_POINT('',(-30.8799792272101,5.5,-2.7252308025327));
#33793=CARTESIAN_POINT('Origin',(-30.3819150461261,5.5,-2.68127546700797));
#33794=CARTESIAN_POINT('Origin',(0.,5.5,0.));
#33795=CARTESIAN_POINT('Origin',(0.,6.,0.));
#33796=CARTESIAN_POINT('Origin',(-34.8644926758824,5.5,-3.07687348673046));
#33797=CARTESIAN_POINT('',(-33.1868376744163,6.,-7.2524541285162));
#33798=CARTESIAN_POINT('',(-33.3732437856903,5.5,-6.78850072387334));
#33799=CARTESIAN_POINT('Origin',(-33.1868376744163,5.5,-7.2524541285162));
#33800=CARTESIAN_POINT('Origin',(-34.8644926758824,5.5,-3.07687348673046));
#33801=CARTESIAN_POINT('Origin',(-34.8644926758824,6.,-3.07687348673046));
#33802=CARTESIAN_POINT('Origin',(-30.9499643391281,5.5,-12.8198949842305));
#33803=CARTESIAN_POINT('',(-28.5948974602351,6.,-18.3383784711987));
#33804=CARTESIAN_POINT('',(-28.398641886994,5.5,-18.7982520951128));
#33805=CARTESIAN_POINT('Origin',(-28.5948974602351,5.5,-18.3383784711987));
#33806=CARTESIAN_POINT('Origin',(-30.9499643391281,5.5,-12.8198949842305));
#33807=CARTESIAN_POINT('Origin',(-30.9499643391281,6.,-12.8198949842305));
#33808=CARTESIAN_POINT('Origin',(-26.8285973010653,5.5,-22.4772410864249));
#33809=CARTESIAN_POINT('',(-23.3792062194998,6.,-19.5873100895989));
#33810=CARTESIAN_POINT('',(-23.7624718952293,5.5,-19.9084135336907));
#33811=CARTESIAN_POINT('Origin',(-23.3792062194998,5.5,-19.5873100895989));
#33812=CARTESIAN_POINT('Origin',(-26.8285973010653,5.5,-22.4772410864249));
#33813=CARTESIAN_POINT('Origin',(-26.8285973010653,6.,-22.4772410864249));
#33814=CARTESIAN_POINT('Origin',(0.,5.5,0.));
#33815=CARTESIAN_POINT('',(-19.5873100895989,6.,-23.3792062194998));
#33816=CARTESIAN_POINT('',(-19.9084135336907,5.5,-23.7624718952293));
#33817=CARTESIAN_POINT('Origin',(-19.5873100895989,5.5,-23.3792062194998));
#33818=CARTESIAN_POINT('Origin',(0.,5.5,0.));
#33819=CARTESIAN_POINT('Origin',(0.,6.,0.));
#33820=CARTESIAN_POINT('Origin',(-22.4772410864249,5.5,-26.8285973010653));
#33821=CARTESIAN_POINT('',(-18.3383784711988,6.,-28.5948974602351));
#33822=CARTESIAN_POINT('',(-18.7982520951128,5.5,-28.398641886994));
#33823=CARTESIAN_POINT('Origin',(-18.3383784711988,5.5,-28.5948974602351));
#33824=CARTESIAN_POINT('Origin',(-22.4772410864249,5.5,-26.8285973010653));
#33825=CARTESIAN_POINT('Origin',(-22.4772410864249,6.,-26.8285973010653));
#33826=CARTESIAN_POINT('Origin',(-12.8198949842305,5.5,-30.9499643391281));
#33827=CARTESIAN_POINT('',(-7.2524541285162,6.,-33.1868376744162));
#33828=CARTESIAN_POINT('Origin',(-7.2524541285162,5.5,-33.1868376744162));
#33829=CARTESIAN_POINT('Origin',(-12.8198949842305,5.5,-30.9499643391281));
#33830=CARTESIAN_POINT('Origin',(-12.8198949842305,6.,-30.9499643391281));
#33831=CARTESIAN_POINT('Origin',(-3.07687348673047,5.5,-34.8644926758824));
#33832=CARTESIAN_POINT('',(-2.68127546700798,6.,-30.3819150461261));
#33833=CARTESIAN_POINT('Origin',(-2.68127546700798,5.5,-30.3819150461261));
#33834=CARTESIAN_POINT('Origin',(-3.07687348673047,6.,-34.8644926758824));
#33835=CARTESIAN_POINT('Origin',(0.,5.5,0.));
#33836=CARTESIAN_POINT('',(2.68127546700797,6.,-30.3819150461261));
#33837=CARTESIAN_POINT('',(2.72523080253269,5.5,-30.8799792272101));
#33838=CARTESIAN_POINT('Origin',(2.68127546700797,5.5,-30.3819150461261));
#33839=CARTESIAN_POINT('Origin',(0.,5.5,0.));
#33840=CARTESIAN_POINT('Origin',(0.,6.,0.));
#33841=CARTESIAN_POINT('Origin',(3.07687348673046,5.5,-34.8644926758824));
#33842=CARTESIAN_POINT('',(7.25245412851619,6.,-33.1868376744163));
#33843=CARTESIAN_POINT('',(6.78850072387333,5.5,-33.3732437856903));
#33844=CARTESIAN_POINT('Origin',(7.25245412851619,5.5,-33.1868376744163));
#33845=CARTESIAN_POINT('Origin',(3.07687348673046,5.5,-34.8644926758824));
#33846=CARTESIAN_POINT('Origin',(3.07687348673046,6.,-34.8644926758824));
#33847=CARTESIAN_POINT('Origin',(12.8198949842305,5.5,-30.9499643391281));
#33848=CARTESIAN_POINT('',(18.3383784711987,6.,-28.5948974602351));
#33849=CARTESIAN_POINT('',(18.7982520951128,5.5,-28.398641886994));
#33850=CARTESIAN_POINT('Origin',(18.3383784711987,5.5,-28.5948974602351));
#33851=CARTESIAN_POINT('Origin',(12.8198949842305,5.5,-30.9499643391281));
#33852=CARTESIAN_POINT('Origin',(12.8198949842305,6.,-30.9499643391281));
#33853=CARTESIAN_POINT('Origin',(22.4772410864249,5.5,-26.8285973010653));
#33854=CARTESIAN_POINT('',(19.5873100895989,6.,-23.3792062194998));
#33855=CARTESIAN_POINT('',(19.9084135336907,5.5,-23.7624718952293));
#33856=CARTESIAN_POINT('Origin',(19.5873100895989,5.5,-23.3792062194998));
#33857=CARTESIAN_POINT('Origin',(22.4772410864249,5.5,-26.8285973010653));
#33858=CARTESIAN_POINT('Origin',(22.4772410864249,6.,-26.8285973010653));
#33859=CARTESIAN_POINT('Origin',(0.,5.5,0.));
#33860=CARTESIAN_POINT('',(23.3792062194998,6.,-19.5873100895989));
#33861=CARTESIAN_POINT('',(23.7624718952293,5.5,-19.9084135336907));
#33862=CARTESIAN_POINT('Origin',(23.3792062194998,5.5,-19.5873100895989));
#33863=CARTESIAN_POINT('Origin',(0.,5.5,0.));
#33864=CARTESIAN_POINT('Origin',(0.,6.,0.));
#33865=CARTESIAN_POINT('Origin',(26.8285973010653,5.5,-22.4772410864249));
#33866=CARTESIAN_POINT('',(28.5948974602351,6.,-18.3383784711987));
#33867=CARTESIAN_POINT('',(28.398641886994,5.5,-18.7982520951128));
#33868=CARTESIAN_POINT('Origin',(28.5948974602351,5.5,-18.3383784711987));
#33869=CARTESIAN_POINT('Origin',(26.8285973010653,5.5,-22.4772410864249));
#33870=CARTESIAN_POINT('Origin',(26.8285973010653,6.,-22.4772410864249));
#33871=CARTESIAN_POINT('Origin',(30.9499643391281,5.5,-12.8198949842305));
#33872=CARTESIAN_POINT('',(33.1868376744162,6.,-7.25245412851619));
#33873=CARTESIAN_POINT('',(33.3732437856903,5.5,-6.78850072387333));
#33874=CARTESIAN_POINT('Origin',(33.1868376744162,5.5,-7.25245412851619));
#33875=CARTESIAN_POINT('Origin',(30.9499643391281,5.5,-12.8198949842305));
#33876=CARTESIAN_POINT('Origin',(30.9499643391281,6.,-12.8198949842305));
#33877=CARTESIAN_POINT('Origin',(34.8644926758824,5.5,-3.07687348673046));
#33878=CARTESIAN_POINT('',(30.3819150461261,6.,-2.68127546700797));
#33879=CARTESIAN_POINT('',(30.8799792272101,5.5,-2.72523080253269));
#33880=CARTESIAN_POINT('Origin',(30.3819150461261,5.5,-2.68127546700797));
#33881=CARTESIAN_POINT('Origin',(34.8644926758824,5.5,-3.07687348673046));
#33882=CARTESIAN_POINT('Origin',(34.8644926758824,6.,-3.07687348673046));
#33883=CARTESIAN_POINT('Origin',(0.,5.5,0.));
#33884=CARTESIAN_POINT('',(30.3819150461261,6.,2.68127546700798));
#33885=CARTESIAN_POINT('',(30.8799792272101,5.5,2.7252308025327));
#33886=CARTESIAN_POINT('Origin',(30.3819150461261,5.5,2.68127546700798));
#33887=CARTESIAN_POINT('Origin',(0.,5.5,0.));
#33888=CARTESIAN_POINT('Origin',(0.,6.,0.));
#33889=CARTESIAN_POINT('Origin',(34.8644926758824,5.5,3.07687348673047));
#33890=CARTESIAN_POINT('',(33.1868376744163,6.,7.2524541285162));
#33891=CARTESIAN_POINT('',(33.3732437856903,5.5,6.78850072387334));
#33892=CARTESIAN_POINT('Origin',(33.1868376744163,5.5,7.2524541285162));
#33893=CARTESIAN_POINT('Origin',(34.8644926758824,5.5,3.07687348673047));
#33894=CARTESIAN_POINT('Origin',(34.8644926758824,6.,3.07687348673047));
#33895=CARTESIAN_POINT('Origin',(30.9499643391281,5.5,12.8198949842305));
#33896=CARTESIAN_POINT('',(28.5948974602351,6.,18.3383784711987));
#33897=CARTESIAN_POINT('',(28.398641886994,5.5,18.7982520951128));
#33898=CARTESIAN_POINT('Origin',(28.5948974602351,5.5,18.3383784711987));
#33899=CARTESIAN_POINT('Origin',(30.9499643391281,5.5,12.8198949842305));
#33900=CARTESIAN_POINT('Origin',(30.9499643391281,6.,12.8198949842305));
#33901=CARTESIAN_POINT('Origin',(26.8285973010654,5.5,22.4772410864249));
#33902=CARTESIAN_POINT('',(23.3792062194998,6.,19.5873100895989));
#33903=CARTESIAN_POINT('',(23.7624718952293,5.5,19.9084135336906));
#33904=CARTESIAN_POINT('Origin',(23.3792062194998,5.5,19.5873100895989));
#33905=CARTESIAN_POINT('Origin',(26.8285973010654,5.5,22.4772410864249));
#33906=CARTESIAN_POINT('Origin',(26.8285973010654,6.,22.4772410864249));
#33907=CARTESIAN_POINT('Origin',(0.,5.5,0.));
#33908=CARTESIAN_POINT('',(19.5873100895989,6.,23.3792062194998));
#33909=CARTESIAN_POINT('',(19.9084135336907,5.5,23.7624718952293));
#33910=CARTESIAN_POINT('Origin',(19.5873100895989,5.5,23.3792062194998));
#33911=CARTESIAN_POINT('Origin',(0.,5.5,0.));
#33912=CARTESIAN_POINT('Origin',(0.,6.,0.));
#33913=CARTESIAN_POINT('Origin',(22.4772410864249,5.5,26.8285973010653));
#33914=CARTESIAN_POINT('',(18.3383784711988,6.,28.5948974602351));
#33915=CARTESIAN_POINT('',(18.7982520951128,5.5,28.398641886994));
#33916=CARTESIAN_POINT('Origin',(18.3383784711988,5.5,28.5948974602351));
#33917=CARTESIAN_POINT('Origin',(22.4772410864249,5.5,26.8285973010653));
#33918=CARTESIAN_POINT('Origin',(22.4772410864249,6.,26.8285973010653));
#33919=CARTESIAN_POINT('Origin',(12.8198949842305,5.5,30.9499643391281));
#33920=CARTESIAN_POINT('',(7.2524541285162,6.,33.1868376744162));
#33921=CARTESIAN_POINT('',(6.78850072387334,5.5,33.3732437856903));
#33922=CARTESIAN_POINT('Origin',(7.2524541285162,5.5,33.1868376744162));
#33923=CARTESIAN_POINT('Origin',(12.8198949842305,5.5,30.9499643391281));
#33924=CARTESIAN_POINT('Origin',(12.8198949842305,6.,30.9499643391281));
#33925=CARTESIAN_POINT('Origin',(3.07687348673046,5.5,34.8644926758824));
#33926=CARTESIAN_POINT('',(2.68127546700797,6.,30.3819150461261));
#33927=CARTESIAN_POINT('Origin',(2.68127546700797,5.5,30.3819150461261));
#33928=CARTESIAN_POINT('Origin',(3.07687348673046,5.5,34.8644926758824));
#33929=CARTESIAN_POINT('Origin',(3.07687348673046,6.,34.8644926758824));
#33930=CARTESIAN_POINT('Origin',(0.,5.5,0.));
#33931=CARTESIAN_POINT('Origin',(0.,6.,0.));
#33932=CARTESIAN_POINT('Origin',(12.8198949842305,0.,-30.9499643391281));
#33933=CARTESIAN_POINT('',(18.7982520951128,-5.5,-28.398641886994));
#33934=CARTESIAN_POINT('',(18.7982520951128,0.,-28.398641886994));
#33935=CARTESIAN_POINT('',(6.78850072387333,-5.5,-33.3732437856903));
#33936=CARTESIAN_POINT('Origin',(12.8198949842305,-5.5,-30.9499643391281));
#33937=CARTESIAN_POINT('',(6.78850072387333,0.,-33.3732437856903));
#33938=CARTESIAN_POINT('Origin',(22.4772410864249,0.,-26.8285973010653));
#33939=CARTESIAN_POINT('',(19.9084135336907,-5.5,-23.7624718952293));
#33940=CARTESIAN_POINT('',(19.9084135336907,0.,-23.7624718952293));
#33941=CARTESIAN_POINT('Origin',(22.4772410864249,-5.5,-26.8285973010653));
#33942=CARTESIAN_POINT('Origin',(0.,0.,0.));
#33943=CARTESIAN_POINT('',(23.7624718952293,-5.5,-19.9084135336907));
#33944=CARTESIAN_POINT('',(23.7624718952293,0.,-19.9084135336907));
#33945=CARTESIAN_POINT('Origin',(0.,-5.5,0.));
#33946=CARTESIAN_POINT('Origin',(26.8285973010653,0.,-22.4772410864249));
#33947=CARTESIAN_POINT('',(28.398641886994,-5.5,-18.7982520951128));
#33948=CARTESIAN_POINT('',(28.398641886994,0.,-18.7982520951128));
#33949=CARTESIAN_POINT('Origin',(26.8285973010653,-5.5,-22.4772410864249));
#33950=CARTESIAN_POINT('Origin',(30.9499643391281,0.,-12.8198949842305));
#33951=CARTESIAN_POINT('',(33.3732437856903,-5.5,-6.78850072387333));
#33952=CARTESIAN_POINT('',(33.3732437856903,0.,-6.78850072387333));
#33953=CARTESIAN_POINT('Origin',(30.9499643391281,-5.5,-12.8198949842305));
#33954=CARTESIAN_POINT('Origin',(34.8644926758824,0.,-3.07687348673046));
#33955=CARTESIAN_POINT('',(30.8799792272101,-5.5,-2.72523080253269));
#33956=CARTESIAN_POINT('',(30.8799792272101,0.,-2.72523080253269));
#33957=CARTESIAN_POINT('Origin',(34.8644926758824,-5.5,-3.07687348673046));
#33958=CARTESIAN_POINT('Origin',(0.,0.,0.));
#33959=CARTESIAN_POINT('',(30.8799792272101,-5.5,2.7252308025327));
#33960=CARTESIAN_POINT('',(30.8799792272101,0.,2.7252308025327));
#33961=CARTESIAN_POINT('Origin',(0.,-5.5,0.));
#33962=CARTESIAN_POINT('Origin',(34.8644926758824,0.,3.07687348673047));
#33963=CARTESIAN_POINT('',(33.3732437856903,-5.5,6.78850072387334));
#33964=CARTESIAN_POINT('',(33.3732437856903,0.,6.78850072387334));
#33965=CARTESIAN_POINT('Origin',(34.8644926758824,-5.5,3.07687348673047));
#33966=CARTESIAN_POINT('Origin',(30.9499643391281,0.,12.8198949842305));
#33967=CARTESIAN_POINT('',(28.398641886994,-5.5,18.7982520951128));
#33968=CARTESIAN_POINT('',(28.398641886994,0.,18.7982520951128));
#33969=CARTESIAN_POINT('Origin',(30.9499643391281,-5.5,12.8198949842305));
#33970=CARTESIAN_POINT('Origin',(26.8285973010654,0.,22.4772410864249));
#33971=CARTESIAN_POINT('',(23.7624718952293,-5.5,19.9084135336906));
#33972=CARTESIAN_POINT('',(23.7624718952293,0.,19.9084135336906));
#33973=CARTESIAN_POINT('Origin',(26.8285973010654,-5.5,22.4772410864249));
#33974=CARTESIAN_POINT('Origin',(0.,0.,0.));
#33975=CARTESIAN_POINT('',(19.9084135336907,-5.5,23.7624718952293));
#33976=CARTESIAN_POINT('',(19.9084135336907,0.,23.7624718952293));
#33977=CARTESIAN_POINT('Origin',(0.,-5.5,0.));
#33978=CARTESIAN_POINT('Origin',(22.4772410864249,0.,26.8285973010653));
#33979=CARTESIAN_POINT('',(18.7982520951128,-5.5,28.398641886994));
#33980=CARTESIAN_POINT('',(18.7982520951128,0.,28.398641886994));
#33981=CARTESIAN_POINT('Origin',(22.4772410864249,-5.5,26.8285973010653));
#33982=CARTESIAN_POINT('Origin',(12.8198949842305,0.,30.9499643391281));
#33983=CARTESIAN_POINT('',(6.78850072387334,-5.5,33.3732437856903));
#33984=CARTESIAN_POINT('',(6.78850072387334,0.,33.3732437856903));
#33985=CARTESIAN_POINT('Origin',(12.8198949842305,-5.5,30.9499643391281));
#33986=CARTESIAN_POINT('Origin',(3.07687348673046,0.,34.8644926758824));
#33987=CARTESIAN_POINT('',(2.7252308025327,-5.5,30.8799792272101));
#33988=CARTESIAN_POINT('',(2.7252308025327,0.,30.8799792272101));
#33989=CARTESIAN_POINT('Origin',(3.07687348673046,-5.5,34.8644926758824));
#33990=CARTESIAN_POINT('Origin',(0.,0.,0.));
#33991=CARTESIAN_POINT('Origin',(0.,-5.5,0.));
#33992=CARTESIAN_POINT('Origin',(0.,6.,0.));
#33993=CARTESIAN_POINT('',(-3.49024337756996E-15,6.,28.5));
#33994=CARTESIAN_POINT('Origin',(0.,6.,0.));
#33995=CARTESIAN_POINT('',(-12.2458698356829,6.,-29.5641450403612));
#33996=CARTESIAN_POINT('Origin',(-12.8198949842305,6.,-30.9499643391281));
#33997=CARTESIAN_POINT('',(-29.5641450403612,6.,12.2458698356829));
#33998=CARTESIAN_POINT('Origin',(-30.9499643391281,6.,12.8198949842305));
#33999=CARTESIAN_POINT('',(-29.5641450403612,6.,-12.2458698356829));
#34000=CARTESIAN_POINT('Origin',(-30.9499643391281,6.,-12.8198949842305));
#34001=CARTESIAN_POINT('',(29.5641450403612,6.,-12.2458698356829));
#34002=CARTESIAN_POINT('Origin',(30.9499643391281,6.,-12.8198949842305));
#34003=CARTESIAN_POINT('',(29.5641450403612,6.,12.2458698356829));
#34004=CARTESIAN_POINT('Origin',(30.9499643391281,6.,12.8198949842305));
#34005=CARTESIAN_POINT('',(12.2458698356829,6.,-29.5641450403612));
#34006=CARTESIAN_POINT('Origin',(12.8198949842305,6.,-30.9499643391281));
#34007=CARTESIAN_POINT('',(12.2458698356829,6.,29.5641450403612));
#34008=CARTESIAN_POINT('Origin',(12.8198949842305,6.,30.9499643391281));
#34009=CARTESIAN_POINT('',(-12.2458698356829,6.,29.5641450403612));
#34010=CARTESIAN_POINT('Origin',(-12.8198949842305,6.,30.9499643391281));
#34011=CARTESIAN_POINT('Origin',(-22.4772410864249,-5.5,26.8285973010654));
#34012=CARTESIAN_POINT('',(-19.9084135336906,-5.5,23.7624718952293));
#34013=CARTESIAN_POINT('',(-19.5873100895989,-6.,23.3792062194998));
#34014=CARTESIAN_POINT('Origin',(-19.5873100895989,-5.5,23.3792062194998));
#34015=CARTESIAN_POINT('',(-18.3383784711987,-6.,28.5948974602351));
#34016=CARTESIAN_POINT('Origin',(-22.4772410864249,-6.,26.8285973010654));
#34017=CARTESIAN_POINT('',(-18.7982520951128,-5.5,28.398641886994));
#34018=CARTESIAN_POINT('Origin',(-18.3383784711987,-5.5,28.5948974602351));
#34019=CARTESIAN_POINT('Origin',(-22.4772410864249,-5.5,26.8285973010654));
#34020=CARTESIAN_POINT('Origin',(-12.8198949842305,-5.5,30.9499643391281));
#34021=CARTESIAN_POINT('',(-7.2524541285162,-6.,33.1868376744163));
#34022=CARTESIAN_POINT('Origin',(-7.2524541285162,-5.5,33.1868376744163));
#34023=CARTESIAN_POINT('Origin',(-12.8198949842305,-5.5,30.9499643391281));
#34024=CARTESIAN_POINT('Origin',(-12.8198949842305,-6.,30.9499643391281));
#34025=CARTESIAN_POINT('Origin',(-3.07687348673047,-5.5,34.8644926758824));
#34026=CARTESIAN_POINT('',(-2.68127546700798,-6.,30.3819150461261));
#34027=CARTESIAN_POINT('Origin',(-2.68127546700798,-5.5,30.3819150461261));
#34028=CARTESIAN_POINT('Origin',(-3.07687348673047,-6.,34.8644926758824));
#34029=CARTESIAN_POINT('Origin',(0.,-5.5,0.));
#34030=CARTESIAN_POINT('',(2.68127546700797,-6.,30.3819150461261));
#34031=CARTESIAN_POINT('Origin',(2.68127546700797,-5.5,30.3819150461261));
#34032=CARTESIAN_POINT('Origin',(0.,-6.,0.));
#34033=CARTESIAN_POINT('Origin',(3.07687348673046,-5.5,34.8644926758824));
#34034=CARTESIAN_POINT('',(7.2524541285162,-6.,33.1868376744163));
#34035=CARTESIAN_POINT('Origin',(7.2524541285162,-5.5,33.1868376744163));
#34036=CARTESIAN_POINT('Origin',(3.07687348673046,-6.,34.8644926758824));
#34037=CARTESIAN_POINT('Origin',(12.8198949842305,-5.5,30.9499643391281));
#34038=CARTESIAN_POINT('',(18.3383784711987,-6.,28.5948974602351));
#34039=CARTESIAN_POINT('Origin',(18.3383784711987,-5.5,28.5948974602351));
#34040=CARTESIAN_POINT('Origin',(12.8198949842305,-6.,30.9499643391281));
#34041=CARTESIAN_POINT('Origin',(22.4772410864249,-5.5,26.8285973010653));
#34042=CARTESIAN_POINT('',(19.5873100895989,-6.,23.3792062194998));
#34043=CARTESIAN_POINT('Origin',(19.5873100895989,-5.5,23.3792062194998));
#34044=CARTESIAN_POINT('Origin',(22.4772410864249,-6.,26.8285973010653));
#34045=CARTESIAN_POINT('Origin',(0.,-5.5,0.));
#34046=CARTESIAN_POINT('',(23.3792062194998,-6.,19.5873100895989));
#34047=CARTESIAN_POINT('Origin',(23.3792062194998,-5.5,19.5873100895989));
#34048=CARTESIAN_POINT('Origin',(0.,-6.,0.));
#34049=CARTESIAN_POINT('Origin',(26.8285973010654,-5.5,22.4772410864249));
#34050=CARTESIAN_POINT('',(28.5948974602351,-6.,18.3383784711987));
#34051=CARTESIAN_POINT('Origin',(28.5948974602351,-5.5,18.3383784711987));
#34052=CARTESIAN_POINT('Origin',(26.8285973010654,-6.,22.4772410864249));
#34053=CARTESIAN_POINT('Origin',(30.9499643391281,-5.5,12.8198949842305));
#34054=CARTESIAN_POINT('',(33.1868376744163,-6.,7.2524541285162));
#34055=CARTESIAN_POINT('Origin',(33.1868376744163,-5.5,7.2524541285162));
#34056=CARTESIAN_POINT('Origin',(30.9499643391281,-6.,12.8198949842305));
#34057=CARTESIAN_POINT('Origin',(34.8644926758824,-5.5,3.07687348673047));
#34058=CARTESIAN_POINT('',(30.3819150461261,-6.,2.68127546700798));
#34059=CARTESIAN_POINT('Origin',(30.3819150461261,-5.5,2.68127546700798));
#34060=CARTESIAN_POINT('Origin',(34.8644926758824,-6.,3.07687348673047));
#34061=CARTESIAN_POINT('Origin',(0.,-5.5,0.));
#34062=CARTESIAN_POINT('',(30.3819150461261,-6.,-2.68127546700797));
#34063=CARTESIAN_POINT('Origin',(30.3819150461261,-5.5,-2.68127546700797));
#34064=CARTESIAN_POINT('Origin',(0.,-6.,0.));
#34065=CARTESIAN_POINT('Origin',(34.8644926758824,-5.5,-3.07687348673046));
#34066=CARTESIAN_POINT('',(33.1868376744163,-6.,-7.25245412851619));
#34067=CARTESIAN_POINT('Origin',(33.1868376744163,-5.5,-7.25245412851619));
#34068=CARTESIAN_POINT('Origin',(34.8644926758824,-6.,-3.07687348673046));
#34069=CARTESIAN_POINT('Origin',(30.9499643391281,-5.5,-12.8198949842305));
#34070=CARTESIAN_POINT('',(28.5948974602351,-6.,-18.3383784711987));
#34071=CARTESIAN_POINT('Origin',(28.5948974602351,-5.5,-18.3383784711987));
#34072=CARTESIAN_POINT('Origin',(30.9499643391281,-6.,-12.8198949842305));
#34073=CARTESIAN_POINT('Origin',(26.8285973010653,-5.5,-22.4772410864249));
#34074=CARTESIAN_POINT('',(23.3792062194998,-6.,-19.5873100895989));
#34075=CARTESIAN_POINT('Origin',(23.3792062194998,-5.5,-19.5873100895989));
#34076=CARTESIAN_POINT('Origin',(26.8285973010653,-6.,-22.4772410864249));
#34077=CARTESIAN_POINT('Origin',(0.,-5.5,0.));
#34078=CARTESIAN_POINT('',(19.5873100895989,-6.,-23.3792062194998));
#34079=CARTESIAN_POINT('Origin',(19.5873100895989,-5.5,-23.3792062194998));
#34080=CARTESIAN_POINT('Origin',(0.,-6.,0.));
#34081=CARTESIAN_POINT('Origin',(22.4772410864249,-5.5,-26.8285973010653));
#34082=CARTESIAN_POINT('',(18.3383784711987,-6.,-28.5948974602351));
#34083=CARTESIAN_POINT('Origin',(18.3383784711987,-5.5,-28.5948974602351));
#34084=CARTESIAN_POINT('Origin',(22.4772410864249,-6.,-26.8285973010653));
#34085=CARTESIAN_POINT('Origin',(12.8198949842305,-5.5,-30.9499643391281));
#34086=CARTESIAN_POINT('',(7.25245412851619,-6.,-33.1868376744163));
#34087=CARTESIAN_POINT('Origin',(7.25245412851619,-5.5,-33.1868376744163));
#34088=CARTESIAN_POINT('Origin',(12.8198949842305,-6.,-30.9499643391281));
#34089=CARTESIAN_POINT('Origin',(3.07687348673046,-5.5,-34.8644926758824));
#34090=CARTESIAN_POINT('',(2.68127546700797,-6.,-30.3819150461261));
#34091=CARTESIAN_POINT('Origin',(2.68127546700797,-5.5,-30.3819150461261));
#34092=CARTESIAN_POINT('Origin',(3.07687348673046,-5.5,-34.8644926758824));
#34093=CARTESIAN_POINT('Origin',(3.07687348673046,-6.,-34.8644926758824));
#34094=CARTESIAN_POINT('Origin',(0.,-5.5,0.));
#34095=CARTESIAN_POINT('',(-2.68127546700798,-6.,-30.3819150461261));
#34096=CARTESIAN_POINT('Origin',(-2.68127546700798,-5.5,-30.3819150461261));
#34097=CARTESIAN_POINT('Origin',(0.,-6.,0.));
#34098=CARTESIAN_POINT('Origin',(-3.07687348673047,-5.5,-34.8644926758824));
#34099=CARTESIAN_POINT('',(-7.2524541285162,-6.,-33.1868376744162));
#34100=CARTESIAN_POINT('Origin',(-7.2524541285162,-5.5,-33.1868376744162));
#34101=CARTESIAN_POINT('Origin',(-3.07687348673047,-6.,-34.8644926758824));
#34102=CARTESIAN_POINT('Origin',(-12.8198949842305,-5.5,-30.9499643391281));
#34103=CARTESIAN_POINT('',(-18.3383784711988,-6.,-28.5948974602351));
#34104=CARTESIAN_POINT('',(-18.7982520951128,-5.5,-28.398641886994));
#34105=CARTESIAN_POINT('Origin',(-18.3383784711988,-5.5,-28.5948974602351));
#34106=CARTESIAN_POINT('Origin',(-12.8198949842305,-5.5,-30.9499643391281));
#34107=CARTESIAN_POINT('Origin',(-12.8198949842305,-6.,-30.9499643391281));
#34108=CARTESIAN_POINT('Origin',(-22.4772410864249,-5.5,-26.8285973010653));
#34109=CARTESIAN_POINT('',(-19.5873100895989,-6.,-23.3792062194998));
#34110=CARTESIAN_POINT('',(-19.9084135336907,-5.5,-23.7624718952293));
#34111=CARTESIAN_POINT('Origin',(-19.5873100895989,-5.5,-23.3792062194998));
#34112=CARTESIAN_POINT('Origin',(-22.4772410864249,-5.5,-26.8285973010653));
#34113=CARTESIAN_POINT('Origin',(-22.4772410864249,-6.,-26.8285973010653));
#34114=CARTESIAN_POINT('Origin',(0.,-5.5,0.));
#34115=CARTESIAN_POINT('',(-23.3792062194998,-6.,-19.5873100895989));
#34116=CARTESIAN_POINT('',(-23.7624718952293,-5.5,-19.9084135336907));
#34117=CARTESIAN_POINT('Origin',(-23.3792062194998,-5.5,-19.5873100895989));
#34118=CARTESIAN_POINT('Origin',(0.,-5.5,0.));
#34119=CARTESIAN_POINT('Origin',(0.,-6.,0.));
#34120=CARTESIAN_POINT('Origin',(-26.8285973010653,-5.5,-22.4772410864249));
#34121=CARTESIAN_POINT('',(-28.5948974602351,-6.,-18.3383784711987));
#34122=CARTESIAN_POINT('',(-28.398641886994,-5.5,-18.7982520951128));
#34123=CARTESIAN_POINT('Origin',(-28.5948974602351,-5.5,-18.3383784711987));
#34124=CARTESIAN_POINT('Origin',(-26.8285973010653,-5.5,-22.4772410864249));
#34125=CARTESIAN_POINT('Origin',(-26.8285973010653,-6.,-22.4772410864249));
#34126=CARTESIAN_POINT('Origin',(-30.9499643391281,-5.5,-12.8198949842305));
#34127=CARTESIAN_POINT('',(-33.1868376744163,-6.,-7.2524541285162));
#34128=CARTESIAN_POINT('',(-33.3732437856903,-5.5,-6.78850072387334));
#34129=CARTESIAN_POINT('Origin',(-33.1868376744163,-5.5,-7.2524541285162));
#34130=CARTESIAN_POINT('Origin',(-30.9499643391281,-5.5,-12.8198949842305));
#34131=CARTESIAN_POINT('Origin',(-30.9499643391281,-6.,-12.8198949842305));
#34132=CARTESIAN_POINT('Origin',(-34.8644926758824,-5.5,-3.07687348673046));
#34133=CARTESIAN_POINT('',(-30.3819150461261,-6.,-2.68127546700797));
#34134=CARTESIAN_POINT('',(-30.8799792272101,-5.5,-2.7252308025327));
#34135=CARTESIAN_POINT('Origin',(-30.3819150461261,-5.5,-2.68127546700797));
#34136=CARTESIAN_POINT('Origin',(-34.8644926758824,-5.5,-3.07687348673046));
#34137=CARTESIAN_POINT('Origin',(-34.8644926758824,-6.,-3.07687348673046));
#34138=CARTESIAN_POINT('Origin',(0.,-5.5,0.));
#34139=CARTESIAN_POINT('',(-30.3819150461261,-6.,2.68127546700798));
#34140=CARTESIAN_POINT('',(-30.8799792272101,-5.5,2.7252308025327));
#34141=CARTESIAN_POINT('Origin',(-30.3819150461261,-5.5,2.68127546700798));
#34142=CARTESIAN_POINT('Origin',(0.,-5.5,0.));
#34143=CARTESIAN_POINT('Origin',(0.,-6.,0.));
#34144=CARTESIAN_POINT('Origin',(-34.8644926758824,-5.5,3.07687348673047));
#34145=CARTESIAN_POINT('',(-33.1868376744162,-6.,7.2524541285162));
#34146=CARTESIAN_POINT('',(-33.3732437856903,-5.5,6.78850072387334));
#34147=CARTESIAN_POINT('Origin',(-33.1868376744162,-5.5,7.2524541285162));
#34148=CARTESIAN_POINT('Origin',(-34.8644926758824,-5.5,3.07687348673047));
#34149=CARTESIAN_POINT('Origin',(-34.8644926758824,-6.,3.07687348673047));
#34150=CARTESIAN_POINT('Origin',(-30.9499643391281,-5.5,12.8198949842305));
#34151=CARTESIAN_POINT('',(-28.5948974602351,-6.,18.3383784711987));
#34152=CARTESIAN_POINT('',(-28.398641886994,-5.5,18.7982520951128));
#34153=CARTESIAN_POINT('Origin',(-28.5948974602351,-5.5,18.3383784711987));
#34154=CARTESIAN_POINT('Origin',(-30.9499643391281,-5.5,12.8198949842305));
#34155=CARTESIAN_POINT('Origin',(-30.9499643391281,-6.,12.8198949842305));
#34156=CARTESIAN_POINT('Origin',(-26.8285973010653,-5.5,22.4772410864249));
#34157=CARTESIAN_POINT('',(-23.3792062194998,-6.,19.5873100895989));
#34158=CARTESIAN_POINT('',(-23.7624718952293,-5.5,19.9084135336906));
#34159=CARTESIAN_POINT('Origin',(-23.3792062194998,-5.5,19.5873100895989));
#34160=CARTESIAN_POINT('Origin',(-26.8285973010653,-5.5,22.4772410864249));
#34161=CARTESIAN_POINT('Origin',(-26.8285973010653,-6.,22.4772410864249));
#34162=CARTESIAN_POINT('Origin',(0.,-5.5,0.));
#34163=CARTESIAN_POINT('Origin',(0.,-6.,0.));
#34164=CARTESIAN_POINT('Origin',(0.,-5.5,0.));
#34165=CARTESIAN_POINT('Origin',(3.07687348673046,0.,-34.8644926758824));
#34166=CARTESIAN_POINT('',(2.72523080253269,0.,-30.8799792272101));
#34167=CARTESIAN_POINT('Origin',(0.,0.,0.));
#34168=CARTESIAN_POINT('Origin',(-12.8198949842305,0.,-30.9499643391281));
#34169=CARTESIAN_POINT('',(-18.7982520951128,0.,-28.398641886994));
#34170=CARTESIAN_POINT('Origin',(-22.4772410864249,0.,-26.8285973010653));
#34171=CARTESIAN_POINT('',(-19.9084135336907,0.,-23.7624718952293));
#34172=CARTESIAN_POINT('Origin',(0.,0.,0.));
#34173=CARTESIAN_POINT('',(-23.7624718952293,0.,-19.9084135336907));
#34174=CARTESIAN_POINT('Origin',(-26.8285973010653,0.,-22.4772410864249));
#34175=CARTESIAN_POINT('',(-28.398641886994,0.,-18.7982520951128));
#34176=CARTESIAN_POINT('Origin',(-30.9499643391281,0.,-12.8198949842305));
#34177=CARTESIAN_POINT('',(-33.3732437856903,0.,-6.78850072387334));
#34178=CARTESIAN_POINT('Origin',(-34.8644926758824,0.,-3.07687348673046));
#34179=CARTESIAN_POINT('',(-30.8799792272101,0.,-2.7252308025327));
#34180=CARTESIAN_POINT('Origin',(0.,0.,0.));
#34181=CARTESIAN_POINT('',(-30.8799792272101,0.,2.7252308025327));
#34182=CARTESIAN_POINT('Origin',(-34.8644926758824,0.,3.07687348673047));
#34183=CARTESIAN_POINT('',(-33.3732437856903,0.,6.78850072387334));
#34184=CARTESIAN_POINT('Origin',(-30.9499643391281,0.,12.8198949842305));
#34185=CARTESIAN_POINT('',(-28.398641886994,0.,18.7982520951128));
#34186=CARTESIAN_POINT('Origin',(-26.8285973010653,0.,22.4772410864249));
#34187=CARTESIAN_POINT('',(-23.7624718952293,0.,19.9084135336906));
#34188=CARTESIAN_POINT('Origin',(0.,0.,0.));
#34189=CARTESIAN_POINT('',(-19.9084135336906,0.,23.7624718952293));
#34190=CARTESIAN_POINT('Origin',(-22.4772410864249,0.,26.8285973010654));
#34191=CARTESIAN_POINT('',(-18.7982520951128,0.,28.398641886994));
#34192=CARTESIAN_POINT('Origin',(0.,-6.,0.));
#34193=CARTESIAN_POINT('',(-3.49024337756996E-15,-6.,-28.5));
#34194=CARTESIAN_POINT('Origin',(0.,-6.,0.));
#34195=CARTESIAN_POINT('',(-12.2458698356829,-6.,-29.5641450403612));
#34196=CARTESIAN_POINT('Origin',(-12.8198949842305,-6.,-30.9499643391281));
#34197=CARTESIAN_POINT('',(29.5641450403612,-6.,12.2458698356829));
#34198=CARTESIAN_POINT('Origin',(30.9499643391281,-6.,12.8198949842305));
#34199=CARTESIAN_POINT('',(29.5641450403612,-6.,-12.2458698356829));
#34200=CARTESIAN_POINT('Origin',(30.9499643391281,-6.,-12.8198949842305));
#34201=CARTESIAN_POINT('',(12.2458698356829,-6.,-29.5641450403612));
#34202=CARTESIAN_POINT('Origin',(12.8198949842305,-6.,-30.9499643391281));
#34203=CARTESIAN_POINT('',(-29.5641450403612,-6.,-12.2458698356829));
#34204=CARTESIAN_POINT('Origin',(-30.9499643391281,-6.,-12.8198949842305));
#34205=CARTESIAN_POINT('',(12.2458698356829,-6.,29.5641450403612));
#34206=CARTESIAN_POINT('Origin',(12.8198949842305,-6.,30.9499643391281));
#34207=CARTESIAN_POINT('',(-29.5641450403612,-6.,12.2458698356829));
#34208=CARTESIAN_POINT('Origin',(-30.9499643391281,-6.,12.8198949842305));
#34209=CARTESIAN_POINT('',(-12.2458698356829,-6.,29.5641450403612));
#34210=CARTESIAN_POINT('Origin',(-12.8198949842305,-6.,30.9499643391281));
#34211=CARTESIAN_POINT('Origin',(0.,5.5,0.));
#34212=CARTESIAN_POINT('',(-3.42901103761259E-15,5.5,28.));
#34213=CARTESIAN_POINT('Origin',(-3.49024337756996E-15,5.5,28.5));
#34214=CARTESIAN_POINT('',(-28.,5.5,-3.42901103761259E-15));
#34215=CARTESIAN_POINT('Origin',(0.,5.5,0.));
#34216=CARTESIAN_POINT('Origin',(0.,5.5,0.));
#34217=CARTESIAN_POINT('Origin',(0.,0.,0.));
#34218=CARTESIAN_POINT('',(-28.,-5.5,-3.42901103761259E-15));
#34219=CARTESIAN_POINT('',(-28.,0.,-3.42901103761259E-15));
#34220=CARTESIAN_POINT('',(-3.42901103761259E-15,-5.5,-28.));
#34221=CARTESIAN_POINT('Origin',(0.,-5.5,0.));
#34222=CARTESIAN_POINT('Origin',(0.,-5.5,0.));
#34223=CARTESIAN_POINT('Origin',(0.,-5.5,0.));
#34224=CARTESIAN_POINT('Origin',(-3.49024337756996E-15,-5.5,-28.5));
#34225=CARTESIAN_POINT('Origin',(-12.8198949842305,0.,30.9499643391281));
#34226=CARTESIAN_POINT('Origin',(-12.8198949842305,0.,-30.9499643391281));
#34227=CARTESIAN_POINT('',(-12.2458698356829,0.,-29.5641450403612));
#34228=CARTESIAN_POINT('Origin',(-12.8198949842305,0.,30.9499643391281));
#34229=CARTESIAN_POINT('',(-12.2458698356829,0.,29.5641450403612));
#34230=CARTESIAN_POINT('Origin',(-30.9499643391281,0.,12.8198949842305));
#34231=CARTESIAN_POINT('',(-29.5641450403612,0.,12.2458698356829));
#34232=CARTESIAN_POINT('Origin',(12.8198949842305,0.,30.9499643391281));
#34233=CARTESIAN_POINT('',(12.2458698356829,0.,29.5641450403612));
#34234=CARTESIAN_POINT('Origin',(-30.9499643391281,0.,-12.8198949842305));
#34235=CARTESIAN_POINT('',(-29.5641450403612,0.,-12.2458698356829));
#34236=CARTESIAN_POINT('Origin',(12.8198949842305,0.,-30.9499643391281));
#34237=CARTESIAN_POINT('',(12.2458698356829,0.,-29.5641450403612));
#34238=CARTESIAN_POINT('Origin',(30.9499643391281,0.,-12.8198949842305));
#34239=CARTESIAN_POINT('',(29.5641450403612,0.,-12.2458698356829));
#34240=CARTESIAN_POINT('Origin',(30.9499643391281,0.,12.8198949842305));
#34241=CARTESIAN_POINT('',(29.5641450403612,0.,12.2458698356829));
#34391=UNCERTAINTY_MEASURE_WITH_UNIT(LENGTH_MEASURE(0.01),#34404,
'DISTANCE_ACCURACY_VALUE',
'Maximum model space distance between geometric entities at asserted c
onnectivities');
#34393=UNCERTAINTY_MEASURE_WITH_UNIT(LENGTH_MEASURE(0.01),#34404,
'DISTANCE_ACCURACY_VALUE',
'Maximum model space distance between geometric entities at asserted c
onnectivities');
#34401=(
GEOMETRIC_REPRESENTATION_CONTEXT(3)
GLOBAL_UNCERTAINTY_ASSIGNED_CONTEXT((#34391))
GLOBAL_UNIT_ASSIGNED_CONTEXT((#34404,#34406,#34407))
REPRESENTATION_CONTEXT('','3D')
);
#34403=(
GEOMETRIC_REPRESENTATION_CONTEXT(3)
GLOBAL_UNCERTAINTY_ASSIGNED_CONTEXT((#34393))
GLOBAL_UNIT_ASSIGNED_CONTEXT((#34404,#34406,#34407))
REPRESENTATION_CONTEXT('','3D')
);
#34404=(
LENGTH_UNIT()
NAMED_UNIT(*)
SI_UNIT(.MILLI.,.METRE.)
);
#34406=(
NAMED_UNIT(*)
PLANE_ANGLE_UNIT()
SI_UNIT($,.RADIAN.)
);
#34407=(
NAMED_UNIT(*)
SI_UNIT($,.STERADIAN.)
SOLID_ANGLE_UNIT()
);
#34415=SHAPE_DEFINITION_REPRESENTATION(#34424,#34441);
#34424=PRODUCT_DEFINITION_SHAPE('',$,#34451);
#34441=SHAPE_REPRESENTATION('',(#4604),#34401);
#34443=PRODUCT_DEFINITION_CONTEXT('part definition',#34472,'design');
#34451=PRODUCT_DEFINITION('Steel_Body','Steel_Body',#34460,#34443);
#34460=PRODUCT_DEFINITION_FORMATION('',$,#34481);
#34472=APPLICATION_CONTEXT(
'Core Data for Automotive Mechanical Design Process');
#34473=PRODUCT_CONTEXT('part definition',#34472,'mechanical');
#34481=PRODUCT('Steel_Body','Steel_Body',$,(#34473));
#34484=PRESENTATION_STYLE_ASSIGNMENT((#34486));
#34486=SURFACE_STYLE_USAGE(.BOTH.,#34488);
#34488=SURFACE_SIDE_STYLE('',(#34490));
#34490=SURFACE_STYLE_FILL_AREA(#34492);
#34492=FILL_AREA_STYLE('Opaque(160,160,160)',(#34494));
#34494=FILL_AREA_STYLE_COLOUR('Opaque(160,160,160)',#34496);
#34496=COLOUR_RGB('Opaque(160,160,160)', 0.09019608, 0.27058824, 0.51372549);
ENDSEC;
END-ISO-10303-21;
